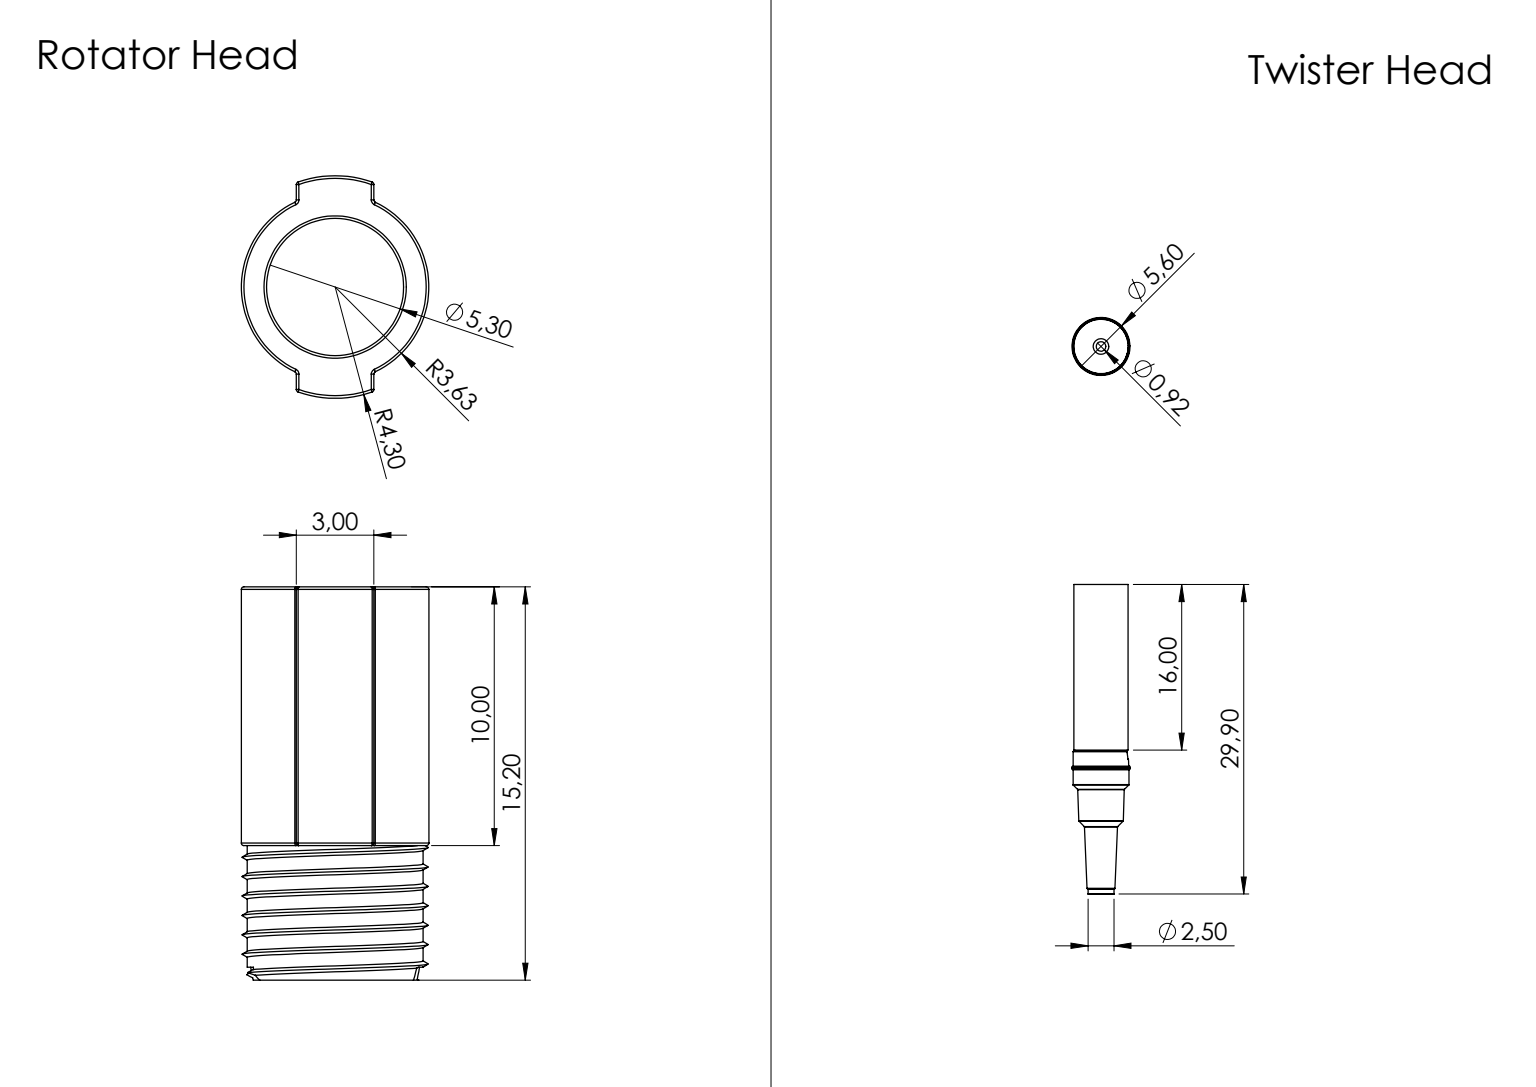
ISO-10303-21;
HEADER;
FILE_DESCRIPTION (('STEP AP214'),
    '1' );
FILE_NAME ('Rotator Head.step',
    '2026-10-06T14:00:01',
    ( '' ),
    ( '' ),
    'SwSTEP 2.0',
    'SolidWorks 2020',
    '' );
FILE_SCHEMA (( 'AUTOMOTIVE_DESIGN' ));
ENDSEC;

DATA;
#20=FACE_OUTER_BOUND ( 'NONE', #25184, .T. ) ;
#32=CARTESIAN_POINT ( 'NONE',  ( -59.59999999999998721, -2.157671697750204842, 1.538490443495526216 ) ) ;
#34=CARTESIAN_POINT ( 'NONE',  ( -60.95655989232410121, 1.962990915244748891, -3.400000000000207301 ) ) ;
#37=PRODUCT_DEFINITION_SHAPE ( 'NONE', 'NONE',  #1193 ) ;
#38=ORIENTED_EDGE ( 'NONE', *, *, #18350, .T. ) ;
#40=CARTESIAN_POINT ( 'NONE',  ( -59.74999999999995737, 2.023778652682510945E-14, -3.400000000000212186 ) ) ;
#45=EDGE_CURVE ( 'NONE', #27818, #13704, #24501, .T. ) ;
#46=CARTESIAN_POINT ( 'NONE',  ( -59.69999999999997442, -3.399999999999991473, -2.235080921937235780E-13 ) ) ;
#65=CARTESIAN_POINT ( 'NONE',  ( -57.19702994616204705, 4.156921938165313080, -1.880369327726949834E-13 ) ) ;
#71=CARTESIAN_POINT ( 'NONE',  ( -55.63452994616205416, 3.117691453623979481, 1.799999999999814415 ) ) ;
#72=EDGE_LOOP ( 'NONE', ( #23840, #15915, #20433, #20236, #22335, #16297, #17891, #10389 ) ) ;
#81=CARTESIAN_POINT ( 'NONE',  ( -59.60604010435355349, 3.187076279294280390, -1.184290838417780600 ) ) ;
#86=CARTESIAN_POINT ( 'NONE',  ( -59.59999999999997300, -2.337126060168364994, -1.249136413240117038 ) ) ;
#92=ORIENTED_EDGE ( 'NONE', *, *, #412, .F. ) ;
#106=( BOUNDED_CURVE ( )  B_SPLINE_CURVE ( 2, ( #27982, #6938, #12441, #31145, #14352, #9477, #26546, #29083, #5166 ),
 .UNSPECIFIED., .F., .T. ) 
 B_SPLINE_CURVE_WITH_KNOTS ( ( 3, 2, 2, 2, 3 ),
 ( 0.5833333333333333703, 0.5925925925925925597, 0.6111111111111111605, 0.6296296296296296502, 0.6388888888888889506 ),
 .UNSPECIFIED. ) 
 CURVE ( )  GEOMETRIC_REPRESENTATION_ITEM ( )  RATIONAL_B_SPLINE_CURVE ( ( 0.9330127018922194093, 0.9330127018922197424, 1.000000000000000000, 0.8660254037844387076, 1.000000000000000000, 0.8660254037844387076, 1.000000000000000000, 0.9330127018922189652, 0.9330127018922194093 ) ) 
 REPRESENTATION_ITEM ( '' )  );
#114=CARTESIAN_POINT ( 'NONE',  ( -56.89405989232413674, -3.920666489018330156E-15, 3.399999999999796962 ) ) ;
#151=DIRECTION ( 'NONE',  ( 1.000000000000000000, -1.219044193948983948E-29, 3.491481338843133355E-15 ) ) ;
#160=CARTESIAN_POINT ( 'NONE',  ( -54.49999999999996447, 1.400000000000023670, -3.959797974644871044 ) ) ;
#174=ORIENTED_EDGE ( 'NONE', *, *, #24601, .T. ) ;
#175=DIRECTION ( 'NONE',  ( -3.491481338843133355E-15, -3.491481338843133355E-15, 1.000000000000000000 ) ) ;
#185=CARTESIAN_POINT ( 'NONE',  ( -59.88452994616203995, -3.117691453623976816, 1.799999999999775335 ) ) ;
#197=CARTESIAN_POINT ( 'NONE',  ( -54.49999999999997868, 8.366749974758489177E-15, -2.216533082070116467E-13 ) ) ;
#202=DIRECTION ( 'NONE',  ( 0.000000000000000000, -1.000000000000000000, 0.000000000000000000 ) ) ;
#208=EDGE_CURVE ( 'NONE', #30643, #11413, #10315, .T. ) ;
#214=CARTESIAN_POINT ( 'NONE',  ( -55.32202994616205416, -4.156921938165296204, -2.115361882398036228E-13 ) ) ;
#222=CARTESIAN_POINT ( 'NONE',  ( -54.99999999999997868, 2.944486372867092250, 1.699999999999816103 ) ) ;
#231=CARTESIAN_POINT ( 'NONE',  ( -59.63746166535423043, 3.180335144039268869, -1.202432085119870431 ) ) ;
#259=CARTESIAN_POINT ( 'NONE',  ( -54.45655989232412963, -3.925981830489445379, -2.076939516179772989E-13 ) ) ;
#267=FACE_OUTER_BOUND ( 'NONE', #20625, .T. ) ;
#287=EDGE_LOOP ( 'NONE', ( #23710, #1168, #11704, #9445, #24779, #21712, #30444 ) ) ;
#294=FACE_OUTER_BOUND ( 'NONE', #8468, .T. ) ;
#298=AXIS2_PLACEMENT_3D ( 'NONE', #23512, #1809, #21167 ) ;
#303=CARTESIAN_POINT ( 'NONE',  ( -54.49999999999996447, -1.499999999999978684, -4.029888335922192866 ) ) ;
#309=ORIENTED_EDGE ( 'NONE', *, *, #15470, .F. ) ;
#331=EDGE_CURVE ( 'NONE', #21866, #1670, #17624, .T. ) ;
#334=DIRECTION ( 'NONE',  ( -3.208218335192195507E-15, 0.9428090415820656878, 0.3333333333333268200 ) ) ;
#336=AXIS2_PLACEMENT_3D ( 'NONE', #3654, #22838, #15841 ) ;
#339=CARTESIAN_POINT ( 'NONE',  ( -58.44702994616205416, -2.078460969082657872, 3.599999999999784261 ) ) ;
#375=CARTESIAN_POINT ( 'NONE',  ( -54.33155989232412253, -1.962990915244706924, -3.400000000000199751 ) ) ;
#387=CARTESIAN_POINT ( 'NONE',  ( -59.66183546925923764, -3.174920041538525251, -1.216504307364950854 ) ) ;
#396=DIRECTION ( 'NONE',  ( 0.000000000000000000, -1.000000000000000000, -3.491481338843133355E-15 ) ) ;
#397=CIRCLE ( 'NONE', #4439, 0.1000000000000000472 ) ;
#400=ORIENTED_EDGE ( 'NONE', *, *, #15115, .F. ) ;
#405=CARTESIAN_POINT ( 'NONE',  ( -54.56249999999997158, -1.962990915244707368, -3.400000000000200640 ) ) ;
#412=EDGE_CURVE ( 'NONE', #3421, #11190, #26852, .T. ) ;
#419=CARTESIAN_POINT ( 'NONE',  ( -44.59999999999998721, -1.557046979865776226, 3.273565289174722448 ) ) ;
#421=CARTESIAN_POINT ( 'NONE',  ( -60.13452994616204705, 3.117691453623979481, 1.799999999999798428 ) ) ;
#429=( BOUNDED_CURVE ( )  B_SPLINE_CURVE ( 2, ( #24054, #26755, #4426, #29116, #12032, #9964, #7268, #5054, #28814 ),
 .UNSPECIFIED., .F., .T. ) 
 B_SPLINE_CURVE_WITH_KNOTS ( ( 3, 2, 2, 2, 3 ),
 ( 0.4722222222222222654, 0.4814814814814814548, 0.5000000000000000000, 0.5185185185185184897, 0.5277777777777777901 ),
 .UNSPECIFIED. ) 
 CURVE ( )  GEOMETRIC_REPRESENTATION_ITEM ( )  RATIONAL_B_SPLINE_CURVE ( ( 0.9330127018922194093, 0.9330127018922197424, 1.000000000000000000, 0.8660254037844387076, 1.000000000000000000, 0.8660254037844387076, 1.000000000000000000, 0.9330127018922194093, 0.9330127018922194093 ) ) 
 REPRESENTATION_ITEM ( '' )  );
#435=CARTESIAN_POINT ( 'NONE',  ( -44.49999999999999289, 1.399999999999998135, 3.363870538531281262 ) ) ;
#437=( LENGTH_UNIT ( ) NAMED_UNIT ( * ) SI_UNIT ( .MILLI., .METRE. ) );
#453=DIRECTION ( 'NONE',  ( -2.095850865446309212E-30, -1.000000000000000000, -2.891205793294679411E-15 ) ) ;
#459=DIRECTION ( 'NONE',  ( 1.000000000000000000, -1.219044193948983948E-29, 3.491481338843133355E-15 ) ) ;
#461=B_SPLINE_CURVE_WITH_KNOTS ( 'NONE', 3,
 ( #4222, #6930, #25918, #30983 ),
 .UNSPECIFIED., .F., .F.,
 ( 4, 4 ),
 ( 0.0002256372043837409917, 0.0002420867138521805458 ),
 .UNSPECIFIED. ) ;
#462=CARTESIAN_POINT ( 'NONE',  ( -59.37009172985672478, 3.234433134214944161, -1.048065980887175952 ) ) ;
#470=CARTESIAN_POINT ( 'NONE',  ( -54.46975615167505680, -2.293836137973780165, -2.770930891520435146 ) ) ;
#488=B_SPLINE_CURVE_WITH_KNOTS ( 'NONE', 3,
 ( #12965, #29908, #15508, #8530, #3628, #17581, #20429, #20126, #6019, #10443, #30224, #18216, #25166, #5538, #13122, #20591 ),
 .UNSPECIFIED., .F., .F.,
 ( 4, 3, 3, 3, 3, 4 ),
 ( -2.161317903555403524E-06, 0.000000000000000000, 3.447636036923519868E-05, 7.048537632665564262E-05, 0.0001024680845135426304, 0.0001336460163216753082 ),
 .UNSPECIFIED. ) ;
#492=CARTESIAN_POINT ( 'NONE',  ( -58.50952994616205416, -4.643455692769885398E-15, 3.599999999999791367 ) ) ;
#495=CARTESIAN_POINT ( 'NONE',  ( -59.69999999999998153, -2.279157448682842091, 1.538811659727345349 ) ) ;
#525=CARTESIAN_POINT ( 'NONE',  ( -58.94702994616203284, -2.078460969082631227, -3.600000000000215472 ) ) ;
#527=CARTESIAN_POINT ( 'NONE',  ( -56.49999999999997868, 2.944486372867090029, 1.699999999999814548 ) ) ;
#532=CARTESIAN_POINT ( 'NONE',  ( -44.59999999999999432, -1.400000000000006795, 3.959797974644484242 ) ) ;
#544=FACE_BOUND ( 'NONE', #24096, .T. ) ;
#553=FACE_OUTER_BOUND ( 'NONE', #21182, .T. ) ;
#556=VERTEX_POINT ( 'NONE', #12979 ) ;
#559=DIRECTION ( 'NONE',  ( 1.000000000000000000, -1.219044193948983948E-29, 3.491481338843133355E-15 ) ) ;
#569=CARTESIAN_POINT ( 'NONE',  ( -59.94702994616205416, -2.078460969082657872, 3.599999999999778932 ) ) ;
#572=DIRECTION ( 'NONE',  ( 0.000000000000000000, -1.000000000000000000, -4.336808689942015369E-15 ) ) ;
#576=CARTESIAN_POINT ( 'NONE',  ( -59.67987798884427519, 2.349476376206463879, -1.226921160904890451 ) ) ;
#577=CIRCLE ( 'NONE', #19806, 3.624999999999996447 ) ;
#591=LINE ( 'NONE', #5506, #15902 ) ;
#625=ORIENTED_EDGE ( 'NONE', *, *, #7840, .T. ) ;
#629=CARTESIAN_POINT ( 'NONE',  ( -59.07202994616203995, -4.156921938165296204, -2.246292432604653256E-13 ) ) ;
#632=AXIS2_PLACEMENT_3D ( 'NONE', #9663, #16780, #24048 ) ;
#639=ORIENTED_EDGE ( 'NONE', *, *, #7228, .F. ) ;
#640=CARTESIAN_POINT ( 'NONE',  ( -59.07202994616203995, -4.156921938165296204, -2.246292432604653256E-13 ) ) ;
#642=CARTESIAN_POINT ( 'NONE',  ( -56.58155989232411542, -1.962990915244702483, -3.400000000000209077 ) ) ;
#645=CARTESIAN_POINT ( 'NONE',  ( -56.89405989232413674, -6.418945959278930492E-15, 3.399999999999796962 ) ) ;
#663=ORIENTED_EDGE ( 'NONE', *, *, #21235, .F. ) ;
#664=DIRECTION ( 'NONE',  ( 1.000000000000000000, -1.219044193948983948E-29, 3.491481338843133355E-15 ) ) ;
#671=CARTESIAN_POINT ( 'NONE',  ( -59.69702994616202574, -2.078460969082631227, -3.600000000000218137 ) ) ;
#676=DIRECTION ( 'NONE',  ( 3.491481338843133355E-15, 3.491481338843133355E-15, -1.000000000000000000 ) ) ;
#677=EDGE_CURVE ( 'NONE', #30092, #3236, #13549, .T. ) ;
#682=DIRECTION ( 'NONE',  ( 3.491481338843133355E-15, 3.491481338843133355E-15, -1.000000000000000000 ) ) ;
#683=CARTESIAN_POINT ( 'NONE',  ( -54.39999999999996305, 1.500000000000021538, -3.363870538531680054 ) ) ;
#713=EDGE_CURVE ( 'NONE', #19668, #15709, #16819, .T. ) ;
#717=CARTESIAN_POINT ( 'NONE',  ( -60.20655989232410832, 1.962990915244748891, -3.400000000000205969 ) ) ;
#721=DIRECTION ( 'NONE',  ( 0.000000000000000000, -1.000000000000000000, -3.491481338843137694E-15 ) ) ;
#725=CARTESIAN_POINT ( 'NONE',  ( -59.13207863537445519, -2.357771006092566513, 1.210922106982256663 ) ) ;
#752=ORIENTED_EDGE ( 'NONE', *, *, #11276, .F. ) ;
#758=CARTESIAN_POINT ( 'NONE',  ( -55.19702994616203284, -2.078460969082631227, -3.600000000000202593 ) ) ;
#780=CIRCLE ( 'NONE', #17971, 0.2000000000000000944 ) ;
#786=CARTESIAN_POINT ( 'NONE',  ( -59.63452994616203284, 2.093608279459373297E-14, -3.600000000000211475 ) ) ;
#789=CIRCLE ( 'NONE', #15973, 4.200000000000016165 ) ;
#794=EDGE_CURVE ( 'NONE', #2131, #1323, #2362, .T. ) ;
#796=AXIS2_PLACEMENT_3D ( 'NONE', #14846, #19782, #453 ) ;
#801=DIRECTION ( 'NONE',  ( 1.000000000000000000, -1.219044193948983948E-29, 3.491481338843133355E-15 ) ) ;
#807=AXIS2_PLACEMENT_3D ( 'NONE', #26000, #20498, #30125 ) ;
#817=EDGE_CURVE ( 'NONE', #4631, #20056, #25479, .T. ) ;
#826=VERTEX_POINT ( 'NONE', #15796 ) ;
#827=CYLINDRICAL_SURFACE ( 'NONE', #3289, 4.300000000000016698 ) ;
#828=ORIENTED_EDGE ( 'NONE', *, *, #31168, .F. ) ;
#836=CARTESIAN_POINT ( 'NONE',  ( -59.25952994616205416, -4.643455692769875931E-15, 3.599999999999788702 ) ) ;
#837=EDGE_LOOP ( 'NONE', ( #6700, #8690, #2350, #12267, #14721 ) ) ;
#840=ORIENTED_EDGE ( 'NONE', *, *, #14681, .F. ) ;
#841=CYLINDRICAL_SURFACE ( 'NONE', #1547, 0.1000000000000000472 ) ;
#842=AXIS2_PLACEMENT_3D ( 'NONE', #30434, #23332, #18747 ) ;
#846=CARTESIAN_POINT ( 'NONE',  ( -54.68749999999998579, -3.925981830489445379, -2.085002746943179415E-13 ) ) ;
#860=B_SPLINE_CURVE_WITH_KNOTS ( 'NONE', 3,
 ( #900, #8173, #17841, #27478, #25267, #5795, #1051, #10702, #11800, #2291 ),
 .UNSPECIFIED., .F., .F.,
 ( 4, 3, 3, 4 ),
 ( 1.063942921725272085E-15, 0.0001291030634103491155, 0.0002330573485935334081, 0.0003370282537953245587 ),
 .UNSPECIFIED. ) ;
#864=EDGE_CURVE ( 'NONE', #2131, #12851, #29047, .T. ) ;
#874=CARTESIAN_POINT ( 'NONE',  ( -59.10095151589816709, 2.309095926083573502, 1.300228524717358836 ) ) ;
#876=CARTESIAN_POINT ( 'NONE',  ( -58.81249999999996447, 3.925981830489463142, -1.945260624050196617E-13 ) ) ;
#887=CARTESIAN_POINT ( 'NONE',  ( -59.06249999999995737, -1.962990915244687828, -3.400000000000226841 ) ) ;
#888=ORIENTED_EDGE ( 'NONE', *, *, #6577, .T. ) ;
#891=CARTESIAN_POINT ( 'NONE',  ( -57.08155989232412963, 3.925981830489463142, -1.884825173204143128E-13 ) ) ;
#896=CARTESIAN_POINT ( 'NONE',  ( -59.19976204860608959, -2.440481952758566830, 1.249999143831215687 ) ) ;
#900=CARTESIAN_POINT ( 'NONE',  ( -59.41132486539680713, 3.361433066165957051, 1.250136525132557574 ) ) ;
#902=FACE_OUTER_BOUND ( 'NONE', #1457, .T. ) ;
#904=ADVANCED_FACE ( 'NONE', ( #16596 ), #23720, .F. ) ;
#908=AXIS2_PLACEMENT_3D ( 'NONE', #25148, #17875, #20268 ) ;
#915=ORIENTED_EDGE ( 'NONE', *, *, #13224, .F. ) ;
#916=CARTESIAN_POINT ( 'NONE',  ( -54.49999999999999289, 1.399999999999998135, 3.363870538531246179 ) ) ;
#920=ORIENTED_EDGE ( 'NONE', *, *, #8697, .T. ) ;
#921=CARTESIAN_POINT ( 'NONE',  ( -44.59999999999998721, 1.399999999999995914, 3.959797974644454488 ) ) ;
#922=LINE ( 'NONE', #27667, #8950 ) ;
#928=EDGE_LOOP ( 'NONE', ( #6714, #5334, #16373 ) ) ;
#931=DIRECTION ( 'NONE',  ( 0.000000000000000000, 1.000000000000000000, 4.336808689942015369E-15 ) ) ;
#945=CARTESIAN_POINT ( 'NONE',  ( -58.94702994616202574, -2.078460969082611243, -3.600000000000227018 ) ) ;
#950=VERTEX_POINT ( 'NONE', #419 ) ;
#952=CARTESIAN_POINT ( 'NONE',  ( -54.49305485193549003, -2.337873507123006345, -2.687031364304292680 ) ) ;
#955=ORIENTED_EDGE ( 'NONE', *, *, #22566, .T. ) ;
#961=CARTESIAN_POINT ( 'NONE',  ( -56.19702994616206837, -2.078460969082657872, 3.599999999999791811 ) ) ;
#968=ORIENTED_EDGE ( 'NONE', *, *, #28279, .T. ) ;
#971=ADVANCED_FACE ( 'NONE', ( #9768 ), #9919, .T. ) ;
#973=LINE ( 'NONE', #29606, #20741 ) ;
#977=CARTESIAN_POINT ( 'NONE',  ( -56.68749999999996447, 1.962990915244759771, -3.400000000000186873 ) ) ;
#981=CARTESIAN_POINT ( 'NONE',  ( -59.24236485150797904, -3.064388189877631063, 1.492323961017689493 ) ) ;
#985=FACE_OUTER_BOUND ( 'NONE', #19485, .T. ) ;
#988=CARTESIAN_POINT ( 'NONE',  ( -59.60127941732039147, -2.337454683938988698, -1.248534441610049450 ) ) ;
#995=CARTESIAN_POINT ( 'NONE',  ( -54.49999999999997868, 8.366749974758391359E-15, -1.938977325913827332E-13 ) ) ;
#1002=CARTESIAN_POINT ( 'NONE',  ( -58.63452994616204705, 3.117691453623979481, 1.799999999999803757 ) ) ;
#1004=ORIENTED_EDGE ( 'NONE', *, *, #24904, .T. ) ;
#1010=CARTESIAN_POINT ( 'NONE',  ( -58.87499999999996447, 2.944486372867106905, -1.700000000000196465 ) ) ;
#1032=CARTESIAN_POINT ( 'NONE',  ( -57.62499999999996447, -2.944486372867076707, -1.700000000000215117 ) ) ;
#1040=DIRECTION ( 'NONE',  ( -1.000000000000000000, 1.219044193948983948E-29, -3.491481338843133355E-15 ) ) ;
#1041=DIRECTION ( 'NONE',  ( 0.000000000000000000, -1.000000000000000000, -5.267838178243386187E-15 ) ) ;
#1043=EDGE_CURVE ( 'NONE', #13704, #26101, #4146, .T. ) ;
#1045=CARTESIAN_POINT ( 'NONE',  ( -57.95655989232411542, 1.962990915244748891, -3.400000000000197087 ) ) ;
#1051=CARTESIAN_POINT ( 'NONE',  ( -59.48031779539610397, 3.173620585043683384, 1.369635785239876169 ) ) ;
#1053=CARTESIAN_POINT ( 'NONE',  ( -54.39999999999996305, -1.599999999999981215, -3.363870538531692045 ) ) ;
#1057=ORIENTED_EDGE ( 'NONE', *, *, #12567, .T. ) ;
#1084=STYLED_ITEM ( 'NONE', ( #12456 ), #4756 ) ;
#1087=EDGE_CURVE ( 'NONE', #6214, #21890, #26505, .T. ) ;
#1090=CARTESIAN_POINT ( 'NONE',  ( -59.25952994616205416, -2.272369910876824241E-14, 3.599999999999788702 ) ) ;
#1095=CARTESIAN_POINT ( 'NONE',  ( -54.62499999999997158, -2.944486372867076707, -1.700000000000204903 ) ) ;
#1096=ORIENTED_EDGE ( 'NONE', *, *, #14201, .T. ) ;
#1106=CARTESIAN_POINT ( 'NONE',  ( -58.57202994616204705, 2.078460969082646770, 3.599999999999799805 ) ) ;
#1112=( BOUNDED_CURVE ( )  B_SPLINE_CURVE ( 2, ( #81, #29045, #4984, #14637, #24302 ),
 .UNSPECIFIED., .F., .T. ) 
 B_SPLINE_CURVE_WITH_KNOTS ( ( 3, 2, 3 ),
 ( 0.7562128299816163191, 0.7592592592592593004, 0.7702506610550023947 ),
 .UNSPECIFIED. ) 
 CURVE ( )  GEOMETRIC_REPRESENTATION_ITEM ( )  RATIONAL_B_SPLINE_CURVE ( ( 0.9631718388946364229, 0.9779602168519400118, 1.000000000000000000, 0.9204812946589053801, 0.9353569697113883752 ) ) 
 REPRESENTATION_ITEM ( '' )  );
#1116=CARTESIAN_POINT ( 'NONE',  ( -61.07202994616202574, 2.078460969082674747, -3.600000000000208367 ) ) ;
#1119=AXIS2_PLACEMENT_3D ( 'NONE', #13564, #20726, #23248 ) ;
#1132=CARTESIAN_POINT ( 'NONE',  ( -59.60063969940316042, -2.337287690019610231, -1.248834004845451373 ) ) ;
#1146=CARTESIAN_POINT ( 'NONE',  ( -56.20655989232413674, 1.962990915244722245, 3.399999999999807621 ) ) ;
#1151=CARTESIAN_POINT ( 'NONE',  ( -56.43749999999998579, 1.962990915244722689, 3.399999999999807621 ) ) ;
#1159=DIRECTION ( 'NONE',  ( 0.000000000000000000, 1.000000000000000000, 3.491481338843130594E-15 ) ) ;
#1161=CARTESIAN_POINT ( 'NONE',  ( -59.69999999999997442, 3.400000000000007905, -2.001823990013003858E-13 ) ) ;
#1168=ORIENTED_EDGE ( 'NONE', *, *, #3930, .F. ) ;
#1171=CARTESIAN_POINT ( 'NONE',  ( -59.09999999999998010, 2.308634493194285486, 1.301040651491358169 ) ) ;
#1174=CARTESIAN_POINT ( 'NONE',  ( -57.68749999999996447, -3.925981830489445379, -2.189747187108473037E-13 ) ) ;
#1178=CARTESIAN_POINT ( 'NONE',  ( -44.59999999999998010, 8.366749974758271452E-15, -1.593320673368357319E-13 ) ) ;
#1186=CARTESIAN_POINT ( 'NONE',  ( -59.26905989232412253, 2.944486372867092250, 1.699999999999800782 ) ) ;
#1187=DIRECTION ( 'NONE',  ( 0.000000000000000000, -1.000000000000000000, -4.336808689942015369E-15 ) ) ;
#1189=DIRECTION ( 'NONE',  ( -1.000000000000000000, 1.219044193948983948E-29, -3.491481338843133355E-15 ) ) ;
#1193=PRODUCT_DEFINITION ( 'UNKNOWN', '', #11600, #13260 ) ;
#1202=CARTESIAN_POINT ( 'NONE',  ( -59.58155989232410832, -1.962990915244687384, -3.400000000000229061 ) ) ;
#1233=ORIENTED_EDGE ( 'NONE', *, *, #11080, .T. ) ;
#1252=CARTESIAN_POINT ( 'NONE',  ( -54.39999999999999147, -1.600000000000004530, 3.363870538531237742 ) ) ;
#1264=DIRECTION ( 'NONE',  ( 1.000000000000000000, -1.219044193948983948E-29, 3.491481338843133355E-15 ) ) ;
#1272=EDGE_CURVE ( 'NONE', #16489, #14828, #18956, .T. ) ;
#1274=DIRECTION ( 'NONE',  ( -1.000000000000000000, 1.219044193948983948E-29, -3.491481338843133355E-15 ) ) ;
#1275=CARTESIAN_POINT ( 'NONE',  ( -59.64819772016205235, -2.360117159334204739, -1.232121303804351919 ) ) ;
#1278=EDGE_LOOP ( 'NONE', ( #7304, #6677, #15002, #25727 ) ) ;
#1281=AXIS2_PLACEMENT_3D ( 'NONE', #11954, #1983, #11794 ) ;
#1286=ORIENTED_EDGE ( 'NONE', *, *, #5679, .F. ) ;
#1292=CARTESIAN_POINT ( 'NONE',  ( -59.33155989232412253, 3.925981830489463142, -1.963383503328113345E-13 ) ) ;
#1295=ORIENTED_EDGE ( 'NONE', *, *, #23328, .F. ) ;
#1299=CARTESIAN_POINT ( 'NONE',  ( -55.49999999999997868, -2.944486372867089141, 1.699999999999791678 ) ) ;
#1306=EDGE_CURVE ( 'NONE', #30092, #16115, #28416, .T. ) ;
#1308=FACE_OUTER_BOUND ( 'NONE', #31128, .T. ) ;
#1311=CARTESIAN_POINT ( 'NONE',  ( -59.69464122902330416, 2.086944863889884871, 1.740854861534822273 ) ) ;
#1323=VERTEX_POINT ( 'NONE', #6412 ) ;
#1324=CARTESIAN_POINT ( 'NONE',  ( -59.19999999999997442, 4.156921938165309527, 1.250136525132554910 ) ) ;
#1326=CARTESIAN_POINT ( 'NONE',  ( -58.37499999999996447, -2.944486372867076707, -1.700000000000217781 ) ) ;
#1329=CIRCLE ( 'NONE', #6904, 3.399999999999999911 ) ;
#1342=CARTESIAN_POINT ( 'NONE',  ( -58.58155989232412253, 3.925981830489463142, -1.937197393286790192E-13 ) ) ;
#1344=ADVANCED_FACE ( 'NONE', ( #13352 ), #18735, .T. ) ;
#1376=DIRECTION ( 'NONE',  ( 1.000000000000000000, -1.219044193948983948E-29, 3.491481338843133355E-15 ) ) ;
#1390=CARTESIAN_POINT ( 'NONE',  ( -59.19999999999996732, -3.264622394567714192, -0.9498634748674711359 ) ) ;
#1409=ORIENTED_EDGE ( 'NONE', *, *, #26244, .T. ) ;
#1419=CARTESIAN_POINT ( 'NONE',  ( -59.35470925280786503, 2.309531243787677379, 1.299482330928217300 ) ) ;
#1425=DIRECTION ( 'NONE',  ( 1.216509871872722247E-14, 3.491481338843133355E-15, -1.000000000000000000 ) ) ;
#1430=CIRCLE ( 'NONE', #23702, 0.09999999999999992228 ) ;
#1439=CARTESIAN_POINT ( 'NONE',  ( -59.60191903105511813, -2.337626997591211619, -1.248237806062580058 ) ) ;
#1441=ORIENTED_EDGE ( 'NONE', *, *, #3910, .T. ) ;
#1451=VERTEX_POINT ( 'NONE', #23907 ) ;
#1452=SURFACE_STYLE_USAGE ( .BOTH. , #15858 ) ;
#1453=CARTESIAN_POINT ( 'NONE',  ( -55.19702994616203995, -2.078460969082628118, -3.600000000000204814 ) ) ;
#1454=CARTESIAN_POINT ( 'NONE',  ( -59.58155989232410832, -1.962990915244706924, -3.400000000000217515 ) ) ;
#1457=EDGE_LOOP ( 'NONE', ( #15335, #7101, #17819, #1921 ) ) ;
#1458=ORIENTED_EDGE ( 'NONE', *, *, #4399, .T. ) ;
#1461=CARTESIAN_POINT ( 'NONE',  ( -55.43749999999997158, -3.925981830489445379, -2.111188856984502568E-13 ) ) ;
#1465=CARTESIAN_POINT ( 'NONE',  ( -54.49999999999996447, -0.3490374893396158695, -3.419248390956425965 ) ) ;
#1470=CARTESIAN_POINT ( 'NONE',  ( -59.63821477905805324, 2.352792697908280495, -1.234285180173720020 ) ) ;
#1485=CARTESIAN_POINT ( 'NONE',  ( -44.59999999999995879, -1.433333333333312254, -4.054078878803053954 ) ) ;
#1486=CARTESIAN_POINT ( 'NONE',  ( -55.06249999999997158, 3.925981830489463142, -1.814330073843579337E-13 ) ) ;
#1488=ORIENTED_EDGE ( 'NONE', *, *, #4608, .T. ) ;
#1494=ORIENTED_EDGE ( 'NONE', *, *, #13570, .F. ) ;
#1507=CIRCLE ( 'NONE', #14142, 3.399999999999999911 ) ;
#1512=CARTESIAN_POINT ( 'NONE',  ( -59.51662234188409428, -2.295381144444371913, 1.432938519450777326 ) ) ;
#1530=ORIENTED_EDGE ( 'NONE', *, *, #16640, .F. ) ;
#1534=CARTESIAN_POINT ( 'NONE',  ( -56.29806624327023457, 3.400000000000004352, 0.9110272542656333572 ) ) ;
#1541=CARTESIAN_POINT ( 'NONE',  ( -57.82202994616206126, 2.078460969082646770, 3.599999999999802025 ) ) ;
#1546=DIRECTION ( 'NONE',  ( 1.000000000000000000, -1.219044193948983948E-29, 3.491481338843133355E-15 ) ) ;
#1547=AXIS2_PLACEMENT_3D ( 'NONE', #10510, #4108, #5912 ) ;
#1558=CARTESIAN_POINT ( 'NONE',  ( -59.50169947458152819, -2.403253767585091349, -1.124049747732174032 ) ) ;
#1560=DIRECTION ( 'NONE',  ( 0.000000000000000000, -1.000000000000000000, 0.000000000000000000 ) ) ;
#1562=CARTESIAN_POINT ( 'NONE',  ( -60.57202994616203995, -4.156921938165296204, -2.298664652687300067E-13 ) ) ;
#1577=DIRECTION ( 'NONE',  ( 0.000000000000000000, -1.000000000000000000, -4.379659758543263321E-15 ) ) ;
#1579=CARTESIAN_POINT ( 'NONE',  ( -54.39999999999996305, 1.400000000000023670, -3.959797974644871044 ) ) ;
#1587=DIRECTION ( 'NONE',  ( 0.000000000000000000, -1.000000000000000000, -3.491481338843133355E-15 ) ) ;
#1593=ORIENTED_EDGE ( 'NONE', *, *, #1272, .T. ) ;
#1597=CARTESIAN_POINT ( 'NONE',  ( -59.69999999999996732, -2.937205337104083380, -1.958225367202403921 ) ) ;
#1600=CARTESIAN_POINT ( 'NONE',  ( -56.45655989232411542, 1.962990915244748891, -3.400000000000191314 ) ) ;
#1602=ORIENTED_EDGE ( 'NONE', *, *, #208, .T. ) ;
#1607=CARTESIAN_POINT ( 'NONE',  ( -57.12499999999997868, -3.920666489018328579E-15, 3.399999999999796518 ) ) ;
#1608=DIRECTION ( 'NONE',  ( 0.000000000000000000, 1.000000000000000000, 3.491481338843130594E-15 ) ) ;
#1611=CARTESIAN_POINT ( 'NONE',  ( -44.49999999999997868, -2.749999999999991562, -1.685844928847700069E-13 ) ) ;
#1615=CARTESIAN_POINT ( 'NONE',  ( -59.65728261716281366, 2.366782727822268839, -1.230152085140874263 ) ) ;
#1622=CARTESIAN_POINT ( 'NONE',  ( -54.49999999999995737, -3.485114741320604281, -0.1344221940317323061 ) ) ;
#1627=CARTESIAN_POINT ( 'NONE',  ( -59.62499999999996447, 2.944486372867106905, -1.700000000000199130 ) ) ;
#1639=CARTESIAN_POINT ( 'NONE',  ( -54.47481206296395584, -2.548105035733319035, -2.538836448934781664 ) ) ;
#1644=DIRECTION ( 'NONE',  ( 7.637891338979824674E-45, -1.000000000000000000, -3.491481338843135327E-15 ) ) ;
#1646=CARTESIAN_POINT ( 'NONE',  ( -59.41132486540516311, 2.423250918913632201, 1.250136525132548027 ) ) ;
#1670=VERTEX_POINT ( 'NONE', #21711 ) ;
#1684=CARTESIAN_POINT ( 'NONE',  ( -58.88452994616202574, 2.093608279459372350E-14, -3.600000000000208811 ) ) ;
#1690=CARTESIAN_POINT ( 'NONE',  ( -54.39999999999997016, 1.514093959731561467, -3.183260039818582854 ) ) ;
#1697=CARTESIAN_POINT ( 'NONE',  ( -57.24999999999997158, 2.944486372867089585, 1.699999999999812772 ) ) ;
#1705=CARTESIAN_POINT ( 'NONE',  ( -59.14665968485343228, -2.559517124687094913, -0.9190674295589560394 ) ) ;
#1707=CARTESIAN_POINT ( 'NONE',  ( -60.00952994616204705, -4.643455692769866465E-15, 3.599999999999786038 ) ) ;
#1711=VECTOR ( 'NONE', #4485, 1000.000000000000000 ) ;
#1724=DIRECTION ( 'NONE',  ( 1.000000000000000000, -1.219044193948983948E-29, 3.491481338843133355E-15 ) ) ;
#1745=DIRECTION ( 'NONE',  ( 0.000000000000000000, -1.000000000000000000, 0.000000000000000000 ) ) ;
#1750=VERTEX_POINT ( 'NONE', #1390 ) ;
#1753=( NAMED_UNIT ( * ) PLANE_ANGLE_UNIT ( ) SI_UNIT ( $, .RADIAN. ) );
#1755=CARTESIAN_POINT ( 'NONE',  ( -57.08155989232412963, 3.925981830489463142, -1.884825173204143128E-13 ) ) ;
#1761=CARTESIAN_POINT ( 'NONE',  ( -59.24999999999997158, -2.944486372867089141, 1.699999999999778799 ) ) ;
#1762=CARTESIAN_POINT ( 'NONE',  ( -54.95655989232412963, 1.962990915244748891, -3.400000000000186873 ) ) ;
#1764=CIRCLE ( 'NONE', #11908, 0.1000000000000000472 ) ;
#1769=FACE_OUTER_BOUND ( 'NONE', #8576, .T. ) ;
#1780=ADVANCED_FACE ( 'NONE', ( #27682 ), #17831, .T. ) ;
#1783=CARTESIAN_POINT ( 'NONE',  ( -59.69142724121850563, 2.412383461849218591, -1.233589124872089826 ) ) ;
#1784=CARTESIAN_POINT ( 'NONE',  ( -55.82202994616203995, 2.078460969082674747, -3.600000000000189715 ) ) ;
#1788=CIRCLE ( 'NONE', #16470, 0.1000000000000000749 ) ;
#1797=AXIS2_PLACEMENT_3D ( 'NONE', #7442, #459, #10123 ) ;
#1798=EDGE_CURVE ( 'NONE', #21024, #15281, #30548, .T. ) ;
#1804=CIRCLE ( 'NONE', #13399, 0.1000000000000000472 ) ;
#1809=DIRECTION ( 'NONE',  ( 1.000000000000000000, -1.219044193948983948E-29, 3.491481338843133355E-15 ) ) ;
#1817=B_SPLINE_CURVE_WITH_KNOTS ( 'NONE', 3,
 ( #2704, #19960, #3016, #15045, #17748, #10143, #7918 ),
 .UNSPECIFIED., .F., .F.,
 ( 4, 3, 4 ),
 ( 0.000000000000000000, 4.155177920956839920E-05, 5.510430741949099299E-05 ),
 .UNSPECIFIED. ) ;
#1820=CIRCLE ( 'NONE', #4856, 0.1000000000000000472 ) ;
#1821=LINE ( 'NONE', #11495, #16058 ) ;
#1825=VERTEX_POINT ( 'NONE', #11482 ) ;
#1840=CARTESIAN_POINT ( 'NONE',  ( -59.69999999999997442, 8.366749974758454467E-15, -2.120534355533670266E-13 ) ) ;
#1848=VECTOR ( 'NONE', #24236, 1000.000000000000000 ) ;
#1854=CARTESIAN_POINT ( 'NONE',  ( -59.57202994616203995, 2.078460969082674747, -3.600000000000202593 ) ) ;
#1855=VECTOR ( 'NONE', #18825, 1000.000000000000000 ) ;
#1857=AXIS2_PLACEMENT_3D ( 'NONE', #23515, #15768, #11021 ) ;
#1873=SPHERICAL_SURFACE ( 'NONE', #24635, 0.1000000000000000056 ) ;
#1874=ORIENTED_EDGE ( 'NONE', *, *, #12571, .T. ) ;
#1879=DIRECTION ( 'NONE',  ( 0.000000000000000000, -1.000000000000000000, -3.491481338843129017E-15 ) ) ;
#1893=CARTESIAN_POINT ( 'NONE',  ( -55.24005354137803181, -3.399999999999995026, 0.9110272542656064898 ) ) ;
#1909=VECTOR ( 'NONE', #16588, 1000.000000000000000 ) ;
#1921=ORIENTED_EDGE ( 'NONE', *, *, #16414, .T. ) ;
#1934=CARTESIAN_POINT ( 'NONE',  ( -60.14405989232410832, 2.944486372867106461, -1.700000000000200684 ) ) ;
#1938=EDGE_LOOP ( 'NONE', ( #12459, #23077, #1593, #2183, #2772, #8705, #7012, #6440, #1602, #10918, #15569, #29963, #25365, #13655, #18880, #9456, #23543 ) ) ;
#1940=CARTESIAN_POINT ( 'NONE',  ( -56.13452994616205416, -3.117691453623976816, 1.799999999999788436 ) ) ;
#1953=CARTESIAN_POINT ( 'NONE',  ( -59.44102194137920492, 2.226395001412990737, 1.446970701571959728 ) ) ;
#1956=LINE ( 'NONE', #28548, #26629 ) ;
#1957=CARTESIAN_POINT ( 'NONE',  ( -54.39999999999999147, -1.433333333333339343, 4.054078878802656938 ) ) ;
#1962=CARTESIAN_POINT ( 'NONE',  ( -59.74999999999995737, 2.023778652682510945E-14, -3.400000000000212186 ) ) ;
#1964=ORIENTED_EDGE ( 'NONE', *, *, #8148, .T. ) ;
#1970=CARTESIAN_POINT ( 'NONE',  ( -54.38452994616203995, 2.093608279459366986E-14, -3.600000000000193268 ) ) ;
#1975=CARTESIAN_POINT ( 'NONE',  ( -54.49400863111429061, -3.204489435302700695, -1.562885166739987008 ) ) ;
#1983=DIRECTION ( 'NONE',  ( -1.000000000000000000, 1.219044193948983948E-29, -3.491481338843133355E-15 ) ) ;
#2008=CARTESIAN_POINT ( 'NONE',  ( -59.19999999999996732, 3.264622394567737729, -0.9498634748674483763 ) ) ;
#2015=CARTESIAN_POINT ( 'NONE',  ( -54.39999999999996305, -1.399999999999979039, -3.959797974644881258 ) ) ;
#2016=CARTESIAN_POINT ( 'NONE',  ( -58.38452994616204705, -3.117691453623976816, 1.799999999999780442 ) ) ;
#2017=CARTESIAN_POINT ( 'NONE',  ( -59.37009172985672478, 3.234433134214944161, -1.048065980887175952 ) ) ;
#2020=CARTESIAN_POINT ( 'NONE',  ( -59.19999999999997442, -3.371540527096009932, 0.6493167879416990029 ) ) ;
#2032=CARTESIAN_POINT ( 'NONE',  ( -57.37499999999996447, 2.944486372867110902, -1.700000000000183809 ) ) ;
#2041=CARTESIAN_POINT ( 'NONE',  ( -54.49999999999996447, 1.400000000000021450, -3.363870538531680943 ) ) ;
#2048=CARTESIAN_POINT ( 'NONE',  ( -59.69464122902330416, 2.086944863889884871, 1.740854861534822273 ) ) ;
#2057=DIRECTION ( 'NONE',  ( 0.000000000000000000, 1.000000000000000000, 3.491481338843132961E-15 ) ) ;
#2065=CARTESIAN_POINT ( 'NONE',  ( -59.69999999999996732, -1.873569517744609447, -3.074042495181142698 ) ) ;
#2072=ORIENTED_EDGE ( 'NONE', *, *, #4979, .F. ) ;
#2083=CARTESIAN_POINT ( 'NONE',  ( -60.33155989232410121, -1.962990915244706924, -3.400000000000220179 ) ) ;
#2087=CARTESIAN_POINT ( 'NONE',  ( -59.56249999999996447, 3.925981830489463142, -1.971446734091520023E-13 ) ) ;
#2088=PLANE ( 'NONE',  #22096 ) ;
#2095=EDGE_CURVE ( 'NONE', #20905, #12969, #10805, .T. ) ;
#2103=EDGE_LOOP ( 'NONE', ( #1874, #13106, #955, #8764, #22442, #24197 ) ) ;
#2109=ORIENTED_EDGE ( 'NONE', *, *, #20115, .T. ) ;
#2111=DIRECTION ( 'NONE',  ( 1.000000000000000000, -1.219044193948983948E-29, 3.491481338843133355E-15 ) ) ;
#2112=CARTESIAN_POINT ( 'NONE',  ( -60.24999999999997158, 2.944486372867092250, 1.699999999999797673 ) ) ;
#2116=CARTESIAN_POINT ( 'NONE',  ( -59.53611077946203523, 3.324882312671999518, -1.143917123867393304 ) ) ;
#2119=AXIS2_PLACEMENT_3D ( 'NONE', #12111, #21793, #7351 ) ;
#2120=CARTESIAN_POINT ( 'NONE',  ( -54.69702994616206837, -2.078460969082657872, 3.599999999999797584 ) ) ;
#2123=CARTESIAN_POINT ( 'NONE',  ( -59.53056271719990633, -2.463209972446139595, -1.140713948626901120 ) ) ;
#2131=VERTEX_POINT ( 'NONE', #683 ) ;
#2135=CARTESIAN_POINT ( 'NONE',  ( -54.39999999999996305, -1.499999999999981126, -3.363870538531691601 ) ) ;
#2157=VERTEX_POINT ( 'NONE', #4300 ) ;
#2165=CARTESIAN_POINT ( 'NONE',  ( -56.50952994616203995, 3.117691453623994580, -1.800000000000187006 ) ) ;
#2172=CARTESIAN_POINT ( 'NONE',  ( -59.19999999999997442, 4.156921938165317520, -0.9498634748674451567 ) ) ;
#2183=ORIENTED_EDGE ( 'NONE', *, *, #11013, .T. ) ;
#2195=CARTESIAN_POINT ( 'NONE',  ( -55.51905989232413674, 2.944486372867090029, 1.699999999999817213 ) ) ;
#2203=CARTESIAN_POINT ( 'NONE',  ( -57.31249999999996447, 3.400000000000008349, -1.881930883448047941E-13 ) ) ;
#2215=CARTESIAN_POINT ( 'NONE',  ( -55.06249999999997158, 3.400000000000007905, -1.826733775103631524E-13 ) ) ;
#2219=CARTESIAN_POINT ( 'NONE',  ( -59.69999999999997442, 3.400000000000007905, -2.001823990013003858E-13 ) ) ;
#2222=VERTEX_POINT ( 'NONE', #11267 ) ;
#2233=CARTESIAN_POINT ( 'NONE',  ( -59.89405989232412963, -3.920666489018293080E-15, 3.399999999999786304 ) ) ;
#2237=B_SPLINE_CURVE_WITH_KNOTS ( 'NONE', 3,
 ( #11135, #20811, #30132, #1622, #10989, #18434, #20669, #18135 ),
 .UNSPECIFIED., .F., .F.,
 ( 4, 2, 2, 4 ),
 ( 0.001352388525252836175, 0.001863402819022369787, 0.002374417112791903615, 0.003396445700330970839 ),
 .UNSPECIFIED. ) ;
#2238=CARTESIAN_POINT ( 'NONE',  ( -54.44702994616203995, -2.078460969082631227, -3.600000000000199485 ) ) ;
#2260=LINE ( 'NONE', #26488, #13429 ) ;
#2263=CIRCLE ( 'NONE', #18464, 0.1000000000000000472 ) ;
#2266=CARTESIAN_POINT ( 'NONE',  ( -54.75952994616206837, -4.643455692769931152E-15, 3.599999999999804245 ) ) ;
#2270=CARTESIAN_POINT ( 'NONE',  ( -59.56618930482535745, 3.265896025948629600, -1.161282968582738162 ) ) ;
#2273=CARTESIAN_POINT ( 'NONE',  ( -54.75952994616206837, -4.643455692769931152E-15, 3.599999999999804245 ) ) ;
#2288=CARTESIAN_POINT ( 'NONE',  ( -59.40743313238012036, 2.395752775956333291, 1.250136525132548027 ) ) ;
#2290=AXIS2_PLACEMENT_3D ( 'NONE', #12031, #18847, #14381 ) ;
#2291=CARTESIAN_POINT ( 'NONE',  ( -59.51024032614731851, 3.088598804228899652, 1.421463128792039843 ) ) ;
#2302=CARTESIAN_POINT ( 'NONE',  ( -59.11588618124505246, -2.336267030162283653, 1.253430707195199334 ) ) ;
#2317=AXIS2_PLACEMENT_3D ( 'NONE', #23251, #22931, #30357 ) ;
#2318=ORIENTED_EDGE ( 'NONE', *, *, #23511, .F. ) ;
#2325=EDGE_CURVE ( 'NONE', #9593, #10413, #9631, .T. ) ;
#2326=CARTESIAN_POINT ( 'NONE',  ( -56.39405989232412253, 2.944486372867106461, -1.700000000000187583 ) ) ;
#2335=CARTESIAN_POINT ( 'NONE',  ( -59.68658240507107138, -2.223882124562203799, 1.531065007683262591 ) ) ;
#2350=ORIENTED_EDGE ( 'NONE', *, *, #13832, .F. ) ;
#2353=FACE_OUTER_BOUND ( 'NONE', #837, .T. ) ;
#2357=EDGE_LOOP ( 'NONE', ( #7788, #752, #639, #20784 ) ) ;
#2362=LINE ( 'NONE', #12030, #8793 ) ;
#2388=CYLINDRICAL_SURFACE ( 'NONE', #28487, 0.09999999999999982514 ) ;
#2406=DIRECTION ( 'NONE',  ( -2.095850865446309212E-30, -1.000000000000000000, -2.891205793294679411E-15 ) ) ;
#2411=CARTESIAN_POINT ( 'NONE',  ( -60.93749999999997868, 1.962990915244722689, 3.399999999999791633 ) ) ;
#2425=DIRECTION ( 'NONE',  ( 0.000000000000000000, 1.000000000000000000, 3.491481338843130594E-15 ) ) ;
#2439=CARTESIAN_POINT ( 'NONE',  ( -57.13452994616205416, 3.117691453623979481, 1.799999999999809086 ) ) ;
#2442=CARTESIAN_POINT ( 'NONE',  ( -59.48573950359912743, 3.423031164920794289, -1.114835254188495162 ) ) ;
#2446=CARTESIAN_POINT ( 'NONE',  ( -56.07202994616204705, -4.156921938165296204, -2.141547992439359634E-13 ) ) ;
#2449=EDGE_CURVE ( 'NONE', #950, #3421, #973, .T. ) ;
#2463=B_SPLINE_CURVE_WITH_KNOTS ( 'NONE', 3,
 ( #10047, #7803, #29654, #14781 ),
 .UNSPECIFIED., .F., .F.,
 ( 4, 4 ),
 ( 0.000000000000000000, 7.924777108412403711E-05 ),
 .UNSPECIFIED. ) ;
#2468=EDGE_CURVE ( 'NONE', #11413, #17625, #14760, .T. ) ;
#2470=CIRCLE ( 'NONE', #20185, 0.1000000000000001721 ) ;
#2480=EDGE_LOOP ( 'NONE', ( #29463, #7474, #4333, #26667, #1530 ) ) ;
#2493=CARTESIAN_POINT ( 'NONE',  ( -56.14405989232413674, -3.920666489018339623E-15, 3.399999999999799627 ) ) ;
#2504=CARTESIAN_POINT ( 'NONE',  ( -44.59999999999997300, -3.624999999999988010, -1.997442628057709707E-13 ) ) ;
#2511=( BOUNDED_CURVE ( )  B_SPLINE_CURVE ( 3, ( #2017, #28308, #24021, #8986 ),
 .UNSPECIFIED., .F., .T. ) 
 B_SPLINE_CURVE_WITH_KNOTS ( ( 4, 4 ),
 ( 4.399031134232678220, 4.429249381401446861 ),
 .UNSPECIFIED. ) 
 CURVE ( )  GEOMETRIC_REPRESENTATION_ITEM ( )  RATIONAL_B_SPLINE_CURVE ( ( 1.000000000000000000, 0.9999239062424463143, 0.9999239062424463143, 1.000000000000000000 ) ) 
 REPRESENTATION_ITEM ( '' )  );
#2512=AXIS2_PLACEMENT_3D ( 'NONE', #8226, #3489, #30379 ) ;
#2530=CARTESIAN_POINT ( 'NONE',  ( -55.18749999999996447, 1.962990915244749557, -3.400000000000187761 ) ) ;
#2542=CARTESIAN_POINT ( 'NONE',  ( -59.51761855918065436, 2.467398989037824286, -1.133240635510041727 ) ) ;
#2549=EDGE_CURVE ( 'NONE', #28731, #28363, #7089, .T. ) ;
#2573=CARTESIAN_POINT ( 'NONE',  ( -57.50952994616203995, -3.117691453623963938, -1.800000000000215206 ) ) ;
#2575=DIRECTION ( 'NONE',  ( 0.000000000000000000, -1.000000000000000000, -3.491481338843139666E-15 ) ) ;
#2592=VERTEX_POINT ( 'NONE', #6332 ) ;
#2601=EDGE_CURVE ( 'NONE', #10532, #10212, #24224, .T. ) ;
#2602=CARTESIAN_POINT ( 'NONE',  ( -57.13452994616205416, 3.117691453623979481, 1.799999999999809086 ) ) ;
#2609=CARTESIAN_POINT ( 'NONE',  ( -54.81249999999998579, -1.962990915244731793, 3.399999999999796962 ) ) ;
#2640=SPHERICAL_SURFACE ( 'NONE', #24366, 0.1000000000000000056 ) ;
#2641=CARTESIAN_POINT ( 'NONE',  ( -55.45655989232413674, 1.962990915244722245, 3.399999999999810285 ) ) ;
#2642=AXIS2_PLACEMENT_3D ( 'NONE', #10077, #5160, #14512 ) ;
#2648=CARTESIAN_POINT ( 'NONE',  ( -59.09999999999997300, -2.465712773623968790, -0.9709585562669303949 ) ) ;
#2652=( BOUNDED_SURFACE ( )  B_SPLINE_SURFACE ( 3, 2, ( 
 ( #8152, #20210, #20514 ),
 ( #17823, #8465, #27782 ),
 ( #29840, #3566, #20039 ),
 ( #13341, #6097, #15119 ) ),
 .UNSPECIFIED., .F., .F., .F. ) 
 B_SPLINE_SURFACE_WITH_KNOTS ( ( 4, 4 ),
 ( 3, 3 ),
 ( 0.8603049414497402347, 1.079657356097645904 ),
 ( 0.000000000000000000, 1.000000000000000000 ),
 .UNSPECIFIED. ) 
 GEOMETRIC_REPRESENTATION_ITEM ( )  RATIONAL_B_SPLINE_SURFACE ( (
 ( 1.000000000000000000, 0.8142797953134848221, 1.000000000000000000),
 ( 1.000000000000000000, 0.8057719789464390381, 1.000000000000000000),
 ( 1.000000000000000000, 0.7963243424565560336, 1.000000000000000000),
 ( 1.000000000000000000, 0.7860710104634932582, 1.000000000000000000) ) ) 
 REPRESENTATION_ITEM ( '' )  SURFACE ( )  );
#2675=CARTESIAN_POINT ( 'NONE',  ( -44.49999999999999289, -1.514093959731547701, 3.183260039818174292 ) ) ;
#2676=CARTESIAN_POINT ( 'NONE',  ( -55.12499999999997158, 2.944486372867106905, -1.700000000000183364 ) ) ;
#2695=DIRECTION ( 'NONE',  ( 0.000000000000000000, 1.000000000000000000, 3.491481338843133355E-15 ) ) ;
#2703=EDGE_LOOP ( 'NONE', ( #25204, #3417, #7605 ) ) ;
#2704=CARTESIAN_POINT ( 'NONE',  ( -59.19999999999997442, 2.449420067797480893, 1.250136525132548693 ) ) ;
#2712=CARTESIAN_POINT ( 'NONE',  ( -60.13452994616204705, 3.117691453623979481, 1.799999999999798428 ) ) ;
#2713=EDGE_CURVE ( 'NONE', #12851, #3601, #26251, .T. ) ;
#2744=CARTESIAN_POINT ( 'NONE',  ( -55.00952994616204705, 3.117691453623994580, -1.800000000000181899 ) ) ;
#2746=CARTESIAN_POINT ( 'NONE',  ( -56.22099364905387375, -3.399999999999995026, 0.9110272542656009387 ) ) ;
#2764=EDGE_LOOP ( 'NONE', ( #7716, #25036, #18191, #9218, #27487 ) ) ;
#2772=ORIENTED_EDGE ( 'NONE', *, *, #817, .T. ) ;
#2785=CARTESIAN_POINT ( 'NONE',  ( -54.76905989232412963, 2.944486372867092250, 1.699999999999816769 ) ) ;
#2802=SURFACE_STYLE_FILL_AREA ( #7571 ) ;
#2808=CARTESIAN_POINT ( 'NONE',  ( -57.45655989232412253, -3.399999999999991029, -2.148039047887444390E-13 ) ) ;
#2865=EDGE_CURVE ( 'NONE', #6165, #5500, #8545, .T. ) ;
#2868=CARTESIAN_POINT ( 'NONE',  ( -59.69702994616202574, -2.078460969082631227, -3.600000000000218137 ) ) ;
#2885=AXIS2_PLACEMENT_3D ( 'NONE', #24703, #175, #26916 ) ;
#2903=VECTOR ( 'NONE', #1376, 1000.000000000000000 ) ;
#2904=CARTESIAN_POINT ( 'NONE',  ( -61.07202994616202574, 2.078460969082674747, -3.600000000000208367 ) ) ;
#2914=B_SPLINE_CURVE_WITH_KNOTS ( 'NONE', 3,
 ( #22658, #17582, #24989, #27524, #29909, #952, #9988, #27055, #19655, #27226, #10604, #3007, #10444, #22333, #470, #12497 ),
 .UNSPECIFIED., .F., .F.,
 ( 4, 2, 2, 2, 2, 2, 2, 4 ),
 ( 4.367276169273258306E-17, 0.0003166453355160177481, 0.0003958066693950119258, 0.0004353873363345080118, 0.0004452825030693815318, 0.0004551776698042549977, 0.0004749680032740019836, 0.0006332906710319628546 ),
 .UNSPECIFIED. ) ;
#2917=AXIS2_PLACEMENT_3D ( 'NONE', #6284, #15934, #25594 ) ;
#2929=EDGE_LOOP ( 'NONE', ( #4413, #1004, #26925, #14132, #17816, #15391 ) ) ;
#2930=EDGE_CURVE ( 'NONE', #27818, #20905, #21739, .T. ) ;
#2937=DIRECTION ( 'NONE',  ( 0.000000000000000000, -1.000000000000000000, -3.491481338843252079E-15 ) ) ;
#2949=EDGE_CURVE ( 'NONE', #30858, #5493, #3451, .T. ) ;
#2951=CARTESIAN_POINT ( 'NONE',  ( -56.01905989232412963, -2.944486372867088697, 1.699999999999789679 ) ) ;
#2960=( BOUNDED_CURVE ( )  B_SPLINE_CURVE ( 2, ( #17855, #15155, #22614 ),
 .UNSPECIFIED., .F., .T. ) 
 B_SPLINE_CURVE_WITH_KNOTS ( ( 3, 3 ),
 ( 0.6944444444444445308, 0.6961765869809276586 ),
 .UNSPECIFIED. ) 
 CURVE ( )  GEOMETRIC_REPRESENTATION_ITEM ( )  RATIONAL_B_SPLINE_CURVE ( ( 0.9330127018922194093, 0.9330127018922194093, 0.9353569697113865988 ) ) 
 REPRESENTATION_ITEM ( '' )  );
#2967=EDGE_CURVE ( 'NONE', #15088, #12969, #19693, .T. ) ;
#2970=ADVANCED_FACE ( 'NONE', ( #20839 ), #16151, .T. ) ;
#2987=CIRCLE ( 'NONE', #21207, 4.299999999999954525 ) ;
#2995=AXIS2_PLACEMENT_3D ( 'NONE', #6423, #20993, #16391 ) ;
#3007=CARTESIAN_POINT ( 'NONE',  ( -54.48229591105965142, -2.371389875144092496, -2.684526205802663767 ) ) ;
#3015=CARTESIAN_POINT ( 'NONE',  ( -59.00952994616203284, -3.117691453623963938, -1.800000000000220757 ) ) ;
#3016=CARTESIAN_POINT ( 'NONE',  ( -59.19766939034450104, 2.421524988789188093, 1.250136525132548693 ) ) ;
#3024=CARTESIAN_POINT ( 'NONE',  ( -57.88452994616205416, 3.117691453623979481, 1.799999999999806422 ) ) ;
#3031=CARTESIAN_POINT ( 'NONE',  ( -59.69999999999997442, 8.366749974758454467E-15, -2.120534355533670266E-13 ) ) ;
#3038=ORIENTED_EDGE ( 'NONE', *, *, #18261, .F. ) ;
#3046=CARTESIAN_POINT ( 'NONE',  ( -58.12499999999996447, 2.944486372867111346, -1.700000000000185585 ) ) ;
#3051=ORIENTED_EDGE ( 'NONE', *, *, #29412, .F. ) ;
#3059=CARTESIAN_POINT ( 'NONE',  ( -60.57202994616203995, -4.156921938165296204, -2.298664652687300067E-13 ) ) ;
#3098=CARTESIAN_POINT ( 'NONE',  ( -59.58155989232410832, -1.962990915244706924, -3.400000000000217515 ) ) ;
#3104=ADVANCED_FACE ( 'NONE', ( #4517 ), #13166, .T. ) ;
#3119=EDGE_LOOP ( 'NONE', ( #8561, #10506, #21653, #15777 ) ) ;
#3128=CARTESIAN_POINT ( 'NONE',  ( -57.58155989232413674, -1.962990915244744006, 3.399999999999780087 ) ) ;
#3135=EDGE_LOOP ( 'NONE', ( #3562, #28766, #24879, #14573 ) ) ;
#3145=EDGE_CURVE ( 'NONE', #23000, #3568, #6893, .T. ) ;
#3150=CARTESIAN_POINT ( 'NONE',  ( -59.40362242792826919, 3.375967812128700452, 1.250136525132546916 ) ) ;
#3165=CARTESIAN_POINT ( 'NONE',  ( -56.63452994616203284, 2.093608279459369510E-14, -3.600000000000201261 ) ) ;
#3175=CARTESIAN_POINT ( 'NONE',  ( -57.32202994616202574, 2.078460969082674747, -3.600000000000194600 ) ) ;
#3177=CARTESIAN_POINT ( 'NONE',  ( -56.45655989232411542, 1.962990915244759771, -3.400000000000185540 ) ) ;
#3178=CARTESIAN_POINT ( 'NONE',  ( -54.49999999999999289, -1.400000000000006795, 3.959797974644449603 ) ) ;
#3190=CARTESIAN_POINT ( 'NONE',  ( -59.09999999999998010, 2.308634493194285486, 1.301040651491358169 ) ) ;
#3207=CARTESIAN_POINT ( 'NONE',  ( -60.50952994616203284, -3.117691453623963938, -1.800000000000225864 ) ) ;
#3211=AXIS2_PLACEMENT_3D ( 'NONE', #5499, #20080, #29257 ) ;
#3213=AXIS2_PLACEMENT_3D ( 'NONE', #19230, #16692, #27261 ) ;
#3218=CARTESIAN_POINT ( 'NONE',  ( -54.49999999999996447, 2.023778652682504319E-14, -3.400000000000193978 ) ) ;
#3228=CARTESIAN_POINT ( 'NONE',  ( -59.69999155897362186, 2.119262223567999648, 1.750121904846017262 ) ) ;
#3234=CARTESIAN_POINT ( 'NONE',  ( -59.69931151237160805, -2.442379059721019541, -1.238141110944712242 ) ) ;
#3236=VERTEX_POINT ( 'NONE', #27428 ) ;
#3248=ORIENTED_EDGE ( 'NONE', *, *, #7501, .F. ) ;
#3257=CARTESIAN_POINT ( 'NONE',  ( -60.89405989232410121, 2.944486372867106461, -1.700000000000203348 ) ) ;
#3281=ORIENTED_EDGE ( 'NONE', *, *, #20931, .F. ) ;
#3289=AXIS2_PLACEMENT_3D ( 'NONE', #995, #664, #22701 ) ;
#3291=ORIENTED_EDGE ( 'NONE', *, *, #3449, .F. ) ;
#3297=CARTESIAN_POINT ( 'NONE',  ( -59.69999999999998153, 0.3248756580930906579, -3.465281767758778386 ) ) ;
#3298=CARTESIAN_POINT ( 'NONE',  ( -54.63452994616206126, -3.117691453623976816, 1.799999999999793765 ) ) ;
#3305=CARTESIAN_POINT ( 'NONE',  ( -58.24005354137801049, -3.399999999999994138, 0.9110272542655853956 ) ) ;
#3306=CARTESIAN_POINT ( 'NONE',  ( -58.44702994616205416, -2.078460969082659648, 3.599999999999782929 ) ) ;
#3319=FACE_OUTER_BOUND ( 'NONE', #18096, .T. ) ;
#3323=EDGE_LOOP ( 'NONE', ( #11808, #25670, #7534, #21347 ) ) ;
#3324=CARTESIAN_POINT ( 'NONE',  ( -56.88452994616205416, -3.117691453623976816, 1.799999999999785993 ) ) ;
#3332=( BOUNDED_CURVE ( )  B_SPLINE_CURVE ( 2, ( #7629, #10156, #18939, #19824, #645, #29455, #29319, #12361, #12673 ),
 .UNSPECIFIED., .F., .T. ) 
 B_SPLINE_CURVE_WITH_KNOTS ( ( 3, 2, 2, 2, 3 ),
 ( 0.3611111111111111605, 0.3703703703703703498, 0.3888888888888888951, 0.4074074074074073848, 0.4166666666666666852 ),
 .UNSPECIFIED. ) 
 CURVE ( )  GEOMETRIC_REPRESENTATION_ITEM ( )  RATIONAL_B_SPLINE_CURVE ( ( 0.9330127018922194093, 0.9330127018922197424, 1.000000000000000000, 0.8660254037844387076, 1.000000000000000000, 0.8660254037844387076, 1.000000000000000000, 0.9330127018922191873, 0.9330127018922194093 ) ) 
 REPRESENTATION_ITEM ( '' )  );
#3336=EDGE_CURVE ( 'NONE', #7185, #19715, #17395, .T. ) ;
#3337=CARTESIAN_POINT ( 'NONE',  ( -54.39999999999997726, -4.766731106216463600E-14, -1.831402436016377855E-13 ) ) ;
#3343=CARTESIAN_POINT ( 'NONE',  ( -55.02900635094608361, 3.400000000000004352, 0.9110272542656342454 ) ) ;
#3344=VECTOR ( 'NONE', #22872, 1000.000000000000000 ) ;
#3352=CARTESIAN_POINT ( 'NONE',  ( -59.67193011664021185, 2.054846984738300186, 1.719925937563907548 ) ) ;
#3374=CARTESIAN_POINT ( 'NONE',  ( -61.13452994616202574, 2.093608279459375190E-14, -3.600000000000216804 ) ) ;
#3378=DIRECTION ( 'NONE',  ( 2.265029845352616032E-44, -1.000000000000000000, -3.491481338843140061E-15 ) ) ;
#3384=CARTESIAN_POINT ( 'NONE',  ( -58.56249999999997868, -1.962990915244731793, 3.399999999999783640 ) ) ;
#3390=CARTESIAN_POINT ( 'NONE',  ( -54.49999999999999289, -1.400000000000007017, 3.959797974644449603 ) ) ;
#3396=CARTESIAN_POINT ( 'NONE',  ( -59.59999999999997300, 2.337126060168390307, -1.249136413240100607 ) ) ;
#3413=CARTESIAN_POINT ( 'NONE',  ( -56.18749999999997158, -3.925981830489445379, -2.137374967025826226E-13 ) ) ;
#3417=ORIENTED_EDGE ( 'NONE', *, *, #15374, .T. ) ;
#3419=VERTEX_POINT ( 'NONE', #14051 ) ;
#3421=VERTEX_POINT ( 'NONE', #16433 ) ;
#3427=CARTESIAN_POINT ( 'NONE',  ( -44.49999999999996447, -1.399999999999981037, -3.363870538531656518 ) ) ;
#3428=CARTESIAN_POINT ( 'NONE',  ( -59.95655989232412963, 1.962990915244722245, 3.399999999999794742 ) ) ;
#3446=CARTESIAN_POINT ( 'NONE',  ( -59.19999999999996732, -2.580747833305891970, -0.9498634748674686934 ) ) ;
#3449=EDGE_CURVE ( 'NONE', #11045, #19715, #20242, .T. ) ;
#3451=B_SPLINE_CURVE_WITH_KNOTS ( 'NONE', 3,
 ( #10380, #27946, #25101, #20064, #896, #6261, #5639 ),
 .UNSPECIFIED., .F., .F.,
 ( 4, 3, 4 ),
 ( 0.000000000000000000, 3.139320973900864084E-05, 4.461998577547471821E-05 ),
 .UNSPECIFIED. ) ;
#3459=CARTESIAN_POINT ( 'NONE',  ( -44.49999999999999289, -1.400000000000004574, 3.363870538531273269 ) ) ;
#3470=EDGE_CURVE ( 'NONE', #11984, #12035, #23081, .T. ) ;
#3474=CARTESIAN_POINT ( 'NONE',  ( -57.25952994616203995, 3.117691453623998576, -1.800000000000181899 ) ) ;
#3481=DIRECTION ( 'NONE',  ( 0.000000000000000000, 1.000000000000000000, 3.491481338843130594E-15 ) ) ;
#3489=DIRECTION ( 'NONE',  ( -1.163827112947670229E-15, 0.9428090415820664649, 0.3333333333333248771 ) ) ;
#3491=CARTESIAN_POINT ( 'NONE',  ( -59.82202994616204705, -4.156921938165296204, -2.272478542645976661E-13 ) ) ;
#3493=( BOUNDED_CURVE ( )  B_SPLINE_CURVE ( 2, ( #6525, #27899, #25515, #8722, #25834, #20939, #30569, #23169, #8880, #13472, #28220, #16185, #8578, #1453, #4141, #13778, #23461, #11111, #11423, #18728, #21113, #30751, #8427, #6067, #15720, #3673, #13309, #23001, #10956, #20644, #18260, #15499, #20422, #25311, #30047, #27690, #19943, #15183, #24685, #10893, #20272, #5840, #8212, #17880, #18206, #25156, #3474, #22944, #29902, #8362, #12956, #27371, #15024, #12791, #22471, #17730, #20582, #13114, #12641, #18044, #3621, #10740, #30217, #7897, #6009, #3306, #27515, #5682, #22649, #22803, #8064, #15663, #29578, #945, #15332, #24981, #8524, #10595, #1090, #17573, #5531, #5363, #3150 ),
 .UNSPECIFIED., .F., .T. ) 
 B_SPLINE_CURVE_WITH_KNOTS ( ( 3, 2, 2, 2, 2, 2, 2, 2, 2, 2, 2, 2, 2, 2, 2, 2, 2, 2, 2, 2, 2, 2, 2, 2, 2, 2, 2, 2, 2, 2, 2, 2, 2, 2, 2, 2, 2, 2, 2, 2, 2, 3 ),
 ( 0.01191687898796012397, 0.01851851851851851749, 0.03703703703703703498, 0.05555555555555555941, 0.07407407407407406996, 0.09259259259259258745, 0.1111111111111111049, 0.1296296296296296224, 0.1481481481481481399, 0.1666666666666666574, 0.1851851851851851749, 0.2037037037037037202, 0.2222222222222222099, 0.2407407407407407274, 0.2592592592592593004, 0.2777777777777777901, 0.2962962962962962798, 0.3148148148148148251, 0.3333333333333333148, 0.3518518518518518601, 0.3703703703703703498, 0.3888888888888888951, 0.4074074074074073293, 0.4259259259259259855, 0.4444444444444444198, 0.4629629629629629650, 0.4814814814814814548, 0.5000000000000000000, 0.5185185185185184897, 0.5370370370370370905, 0.5555555555555555802, 0.5740740740740740700, 0.5925925925925925597, 0.6111111111111111605, 0.6296296296296296502, 0.6481481481481481399, 0.6666666666666666297, 0.6851851851851852304, 0.7037037037037037202, 0.7222222222222220989, 0.7407407407407408106, 0.7438073466758352570 ),
 .UNSPECIFIED. ) 
 CURVE ( )  GEOMETRIC_REPRESENTATION_ITEM ( )  RATIONAL_B_SPLINE_CURVE ( ( 0.9385312603869460091, 0.9522395925147686402, 1.000000000000000000, 0.8660254037844387076, 1.000000000000000000, 0.8660254037844387076, 1.000000000000000000, 0.8660254037844387076, 1.000000000000000000, 0.8660254037844387076, 1.000000000000000000, 0.8660254037844387076, 1.000000000000000000, 0.8660254037844387076, 1.000000000000000000, 0.8660254037844387076, 1.000000000000000000, 0.8660254037844387076, 1.000000000000000000, 0.8660254037844387076, 1.000000000000000000, 0.8660254037844387076, 1.000000000000000000, 0.8660254037844387076, 1.000000000000000000, 0.8660254037844387076, 1.000000000000000000, 0.8660254037844387076, 1.000000000000000000, 0.8660254037844387076, 1.000000000000000000, 0.8660254037844387076, 1.000000000000000000, 0.8660254037844387076, 1.000000000000000000, 0.8660254037844387076, 1.000000000000000000, 0.8660254037844387076, 1.000000000000000000, 0.8660254037844387076, 1.000000000000000000, 0.8660254037844387076, 1.000000000000000000, 0.8660254037844387076, 1.000000000000000000, 0.8660254037844387076, 1.000000000000000000, 0.8660254037844387076, 1.000000000000000000, 0.8660254037844387076, 1.000000000000000000, 0.8660254037844387076, 1.000000000000000000, 0.8660254037844387076, 1.000000000000000000, 0.8660254037844387076, 1.000000000000000000, 0.8660254037844387076, 1.000000000000000000, 0.8660254037844387076, 1.000000000000000000, 0.8660254037844387076, 1.000000000000000000, 0.8660254037844387076, 1.000000000000000000, 0.8660254037844387076, 1.000000000000000000, 0.8660254037844387076, 1.000000000000000000, 0.8660254037844387076, 1.000000000000000000, 0.8660254037844387076, 1.000000000000000000, 0.8660254037844387076, 1.000000000000000000, 0.8660254037844387076, 1.000000000000000000, 0.8660254037844387076, 1.000000000000000000, 0.8660254037844387076, 1.000000000000000000, 0.9778142462370478238, 0.9629762686038090269 ) ) 
 REPRESENTATION_ITEM ( '' )  );
#3499=CARTESIAN_POINT ( 'NONE',  ( -60.32202994616201863, 2.078460969082674747, -3.600000000000205258 ) ) ;
#3513=DIRECTION ( 'NONE',  ( -1.000000000000000000, 1.219044193948983948E-29, -3.491481338843133355E-15 ) ) ;
#3535=CARTESIAN_POINT ( 'NONE',  ( -59.82202994616204705, -4.156921938165296204, -2.272478542645976661E-13 ) ) ;
#3541=CARTESIAN_POINT ( 'NONE',  ( -57.81249999999998579, -1.962990915244731793, 3.399999999999786304 ) ) ;
#3550=CARTESIAN_POINT ( 'NONE',  ( -59.62735476476905205, 2.346806195053369848, -1.237686616523536287 ) ) ;
#3562=ORIENTED_EDGE ( 'NONE', *, *, #16812, .F. ) ;
#3565=CARTESIAN_POINT ( 'NONE',  ( -58.62499999999998579, -3.920666489018310435E-15, 3.399999999999791189 ) ) ;
#3566=CARTESIAN_POINT ( 'NONE',  ( -59.49223166990491762, 2.264560344927355917, 1.390271221205179986 ) ) ;
#3568=VERTEX_POINT ( 'NONE', #19300 ) ;
#3571=CARTESIAN_POINT ( 'NONE',  ( -59.19999999999996732, 2.580747833305914618, -0.9498634748674507078 ) ) ;
#3575=CARTESIAN_POINT ( 'NONE',  ( -59.18749999999995737, -3.399999999999991029, -2.288065396424332102E-13 ) ) ;
#3577=CARTESIAN_POINT ( 'NONE',  ( -58.20655989232411542, -3.925981830489445379, -2.207870066386390016E-13 ) ) ;
#3601=VERTEX_POINT ( 'NONE', #28936 ) ;
#3612=VERTEX_POINT ( 'NONE', #2504 ) ;
#3614=CIRCLE ( 'NONE', #25350, 2.750000000000000000 ) ;
#3620=CARTESIAN_POINT ( 'NONE',  ( -58.26905989232412253, -2.944486372867094914, 1.699999999999771472 ) ) ;
#3621=CARTESIAN_POINT ( 'NONE',  ( -58.13452994616202574, 3.813458051520598461E-14, -3.600000000000206146 ) ) ;
#3628=CARTESIAN_POINT ( 'NONE',  ( -59.11195455104547136, 2.468319916663101576, -0.9648999906351578559 ) ) ;
#3629=FACE_OUTER_BOUND ( 'NONE', #22604, .T. ) ;
#3635=DIRECTION ( 'NONE',  ( -1.000000000000000000, 1.219044193948983948E-29, -3.491481338843133355E-15 ) ) ;
#3640=CARTESIAN_POINT ( 'NONE',  ( -59.39944685111014877, 2.372743686651884953, 1.252203205371202666 ) ) ;
#3643=CARTESIAN_POINT ( 'NONE',  ( -60.25952994616203284, 3.117691453623994580, -1.800000000000200329 ) ) ;
#3648=CARTESIAN_POINT ( 'NONE',  ( -54.39999999999996305, -1.433333333333312254, -4.054078878803088593 ) ) ;
#3654=CARTESIAN_POINT ( 'NONE',  ( -44.59999999999997300, -4.766731106216475591E-14, -1.489237264809750408E-13 ) ) ;
#3660=CARTESIAN_POINT ( 'NONE',  ( -44.49999999999997868, 8.366749974758366115E-15, -1.867384948185803131E-13 ) ) ;
#3667=ORIENTED_EDGE ( 'NONE', *, *, #24173, .T. ) ;
#3673=CARTESIAN_POINT ( 'NONE',  ( -55.94702994616203995, -2.078460969082627230, -3.600000000000206590 ) ) ;
#3674=CARTESIAN_POINT ( 'NONE',  ( -59.14405989232412963, -3.920666489018302546E-15, 3.399999999999788969 ) ) ;
#3678=CARTESIAN_POINT ( 'NONE',  ( -57.43749999999996447, 1.962990915244749557, -3.400000000000195310 ) ) ;
#3687=B_SPLINE_CURVE_WITH_KNOTS ( 'NONE', 3,
 ( #13294, #23303, #30735, #20925 ),
 .UNSPECIFIED., .F., .F.,
 ( 4, 4 ),
 ( 0.000000000000000000, 3.288265101740379156E-05 ),
 .UNSPECIFIED. ) ;
#3694=CARTESIAN_POINT ( 'NONE',  ( -59.48573950359912743, 3.423031164920794289, -1.114835254188495162 ) ) ;
#3700=CARTESIAN_POINT ( 'NONE',  ( -56.81249999999997158, -1.962990915244707368, -3.400000000000208633 ) ) ;
#3703=AXIS2_PLACEMENT_3D ( 'NONE', #27561, #15705, #6053 ) ;
#3715=CARTESIAN_POINT ( 'NONE',  ( -60.64405989232412253, -3.920666489018283614E-15, 3.399999999999783640 ) ) ;
#3722=CYLINDRICAL_SURFACE ( 'NONE', #15409, 3.399999999999999911 ) ;
#3731=CARTESIAN_POINT ( 'NONE',  ( -59.38263816597098099, 3.123852333407923787, -1.389329043195103752 ) ) ;
#3752=CARTESIAN_POINT ( 'NONE',  ( -44.49999999999997868, 8.366749974758269874E-15, -1.589829192029513996E-13 ) ) ;
#3761=CIRCLE ( 'NONE', #4786, 0.1000000000000000472 ) ;
#3790=EDGE_CURVE ( 'NONE', #11190, #29758, #4787, .T. ) ;
#3791=CARTESIAN_POINT ( 'NONE',  ( -61.13452994616202574, 2.093608279459375190E-14, -3.600000000000216804 ) ) ;
#3798=DIRECTION ( 'NONE',  ( 0.000000000000000000, -1.000000000000000000, -4.336808689942015369E-15 ) ) ;
#3800=AXIS2_PLACEMENT_3D ( 'NONE', #1579, #9352, #28351 ) ;
#3801=CARTESIAN_POINT ( 'NONE',  ( -54.49999999999999289, -1.400000000000007017, 4.029888335921757658 ) ) ;
#3804=CIRCLE ( 'NONE', #8860, 0.1000000000000000472 ) ;
#3806=DIRECTION ( 'NONE',  ( 2.265029845352616032E-44, -1.000000000000000000, -3.491481338843140061E-15 ) ) ;
#3810=FACE_OUTER_BOUND ( 'NONE', #12170, .T. ) ;
#3827=CARTESIAN_POINT ( 'NONE',  ( -57.20655989232410832, 1.962990915244748891, -3.400000000000194422 ) ) ;
#3828=EDGE_LOOP ( 'NONE', ( #23113, #13981, #14538, #25545 ) ) ;
#3833=CARTESIAN_POINT ( 'NONE',  ( -57.68749999999996447, -3.925981830489445379, -2.189747187108473037E-13 ) ) ;
#3846=DIRECTION ( 'NONE',  ( 0.000000000000000000, -1.000000000000000000, -3.491481338843130594E-15 ) ) ;
#3851=DIRECTION ( 'NONE',  ( 1.000000000000000000, -1.219044193948983948E-29, 3.491481338843133355E-15 ) ) ;
#3861=CARTESIAN_POINT ( 'NONE',  ( -55.12499999999997158, 2.944486372867106905, -1.700000000000183364 ) ) ;
#3865=ORIENTED_EDGE ( 'NONE', *, *, #9634, .T. ) ;
#3872=CARTESIAN_POINT ( 'NONE',  ( -59.59999999999997300, -2.337126060168364994, -1.249136413240117038 ) ) ;
#3873=CYLINDRICAL_SURFACE ( 'NONE', #8606, 2.649999999999999911 ) ;
#3891=EDGE_CURVE ( 'NONE', #14560, #10413, #6245, .T. ) ;
#3910=EDGE_CURVE ( 'NONE', #14828, #5117, #7265, .T. ) ;
#3914=CARTESIAN_POINT ( 'NONE',  ( -55.95655989232413674, -3.399999999999990585, -2.144552914728849773E-13 ) ) ;
#3921=DIRECTION ( 'NONE',  ( 0.000000000000000000, 1.000000000000000000, 4.336808689942015369E-15 ) ) ;
#3925=CARTESIAN_POINT ( 'NONE',  ( -57.00952994616205416, -4.643455692769903542E-15, 3.599999999999796696 ) ) ;
#3928=AXIS2_PLACEMENT_3D ( 'NONE', #21061, #3635, #28165 ) ;
#3930=EDGE_CURVE ( 'NONE', #12969, #26147, #10284, .T. ) ;
#3937=CARTESIAN_POINT ( 'NONE',  ( -54.49999999999997868, 3.624999999999963585, -2.089966883537054476E-13 ) ) ;
#3948=EDGE_LOOP ( 'NONE', ( #3291, #7536, #24172, #10290, #12318 ) ) ;
#3952=CARTESIAN_POINT ( 'NONE',  ( -59.40743313238012036, 2.395752775956333291, 1.250136525132548027 ) ) ;
#3955=ORIENTED_EDGE ( 'NONE', *, *, #25501, .F. ) ;
#3974=CARTESIAN_POINT ( 'NONE',  ( -59.60675767627768096, -2.338930541566021759, -1.245993773302377816 ) ) ;
#3982=EDGE_LOOP ( 'NONE', ( #16502, #9555, #23547, #29036 ) ) ;
#3987=CARTESIAN_POINT ( 'NONE',  ( -56.01905989232412963, -2.944486372867088697, 1.699999999999789679 ) ) ;
#3994=CIRCLE ( 'NONE', #4994, 0.1000000000000000472 ) ;
#3995=CARTESIAN_POINT ( 'NONE',  ( -57.99999999999997868, 2.944486372867092250, 1.699999999999805667 ) ) ;
#3996=CARTESIAN_POINT ( 'NONE',  ( -54.83155989232413674, 3.400000000000008349, -1.845326485282803322E-13 ) ) ;
#3998=CARTESIAN_POINT ( 'NONE',  ( -57.45655989232412253, -3.399999999999991029, -2.148039047887444390E-13 ) ) ;
#4001=CARTESIAN_POINT ( 'NONE',  ( -59.09999999999997300, 2.465712773623992327, -0.9709585562669131864 ) ) ;
#4015=AXIS2_PLACEMENT_3D ( 'NONE', #27264, #14906, #5582 ) ;
#4019=CARTESIAN_POINT ( 'NONE',  ( -59.06249999999995737, -1.962990915244707368, -3.400000000000216627 ) ) ;
#4029=PLANE ( 'NONE',  #20658 ) ;
#4030=CARTESIAN_POINT ( 'NONE',  ( -54.39999999999999147, -1.500000000000006661, 3.959797974644449603 ) ) ;
#4034=LINE ( 'NONE', #29999, #8663 ) ;
#4064=VERTEX_POINT ( 'NONE', #20627 ) ;
#4067=DIRECTION ( 'NONE',  ( 1.000000000000000000, -1.219044193948984088E-29, 3.491481338843133750E-15 ) ) ;
#4072=EDGE_CURVE ( 'NONE', #7915, #17824, #24438, .T. ) ;
#4079=CARTESIAN_POINT ( 'NONE',  ( -57.57202994616204705, -4.156921938165296204, -2.193920212522006445E-13 ) ) ;
#4090=CARTESIAN_POINT ( 'NONE',  ( -56.99999999999997158, -2.944486372867094470, 1.699999999999777689 ) ) ;
#4098=CARTESIAN_POINT ( 'NONE',  ( -59.67987798884426809, -2.349476376206443007, -1.226921160904901109 ) ) ;
#4100=CARTESIAN_POINT ( 'NONE',  ( -60.75952994616205416, -4.643455692769856999E-15, 3.599999999999783373 ) ) ;
#4108=DIRECTION ( 'NONE',  ( 1.000000000000000000, -1.219044193948983948E-29, 3.491481338843133355E-15 ) ) ;
#4113=CARTESIAN_POINT ( 'NONE',  ( -59.40362242792826919, 3.375967812128700452, 1.250136525132546916 ) ) ;
#4121=CARTESIAN_POINT ( 'NONE',  ( -44.59999999999998010, 2.650000000000008349, -1.759412204284508433E-13 ) ) ;
#4122=CARTESIAN_POINT ( 'NONE',  ( -59.60996874016036173, 2.024041967860128910, 1.710882463691307143 ) ) ;
#4141=CARTESIAN_POINT ( 'NONE',  ( -55.25952994616203995, -3.117691453623963049, -1.800000000000208544 ) ) ;
#4143=CARTESIAN_POINT ( 'NONE',  ( -58.76905989232410832, 2.023778652682509368E-14, -3.400000000000208189 ) ) ;
#4146=CIRCLE ( 'NONE', #21873, 2.649999999999999911 ) ;
#4148=CARTESIAN_POINT ( 'NONE',  ( -55.82202994616203995, 2.078460969082674747, -3.600000000000189715 ) ) ;
#4168=CARTESIAN_POINT ( 'NONE',  ( -55.75952994616203995, 3.117691453623994580, -1.800000000000184563 ) ) ;
#4174=ADVANCED_FACE ( 'NONE', ( #985 ), #10638, .T. ) ;
#4180=CARTESIAN_POINT ( 'NONE',  ( -54.47064643025908737, -2.407416487588556198, -2.678616765879081374 ) ) ;
#4186=ORIENTED_EDGE ( 'NONE', *, *, #4570, .F. ) ;
#4187=FACE_OUTER_BOUND ( 'NONE', #22497, .T. ) ;
#4208=DIRECTION ( 'NONE',  ( 0.000000000000000000, -1.000000000000000000, 0.000000000000000000 ) ) ;
#4213=DIRECTION ( 'NONE',  ( 1.000000000000000000, -1.219044193948983948E-29, 3.491481338843133355E-15 ) ) ;
#4222=CARTESIAN_POINT ( 'NONE',  ( -59.41132486539680713, 3.361433066165957051, 1.250136525132557574 ) ) ;
#4225=CARTESIAN_POINT ( 'NONE',  ( -56.25952994616206126, -4.643455692769913008E-15, 3.599999999999798916 ) ) ;
#4271=CARTESIAN_POINT ( 'NONE',  ( -59.61691039550309767, 2.025699712120192064, 1.710375399846320255 ) ) ;
#4285=ORIENTED_EDGE ( 'NONE', *, *, #12706, .F. ) ;
#4291=FILL_AREA_STYLE_COLOUR ( '', #31325 ) ;
#4293=CARTESIAN_POINT ( 'NONE',  ( -57.39405989232411542, -2.944486372867076263, -1.700000000000214451 ) ) ;
#4298=CARTESIAN_POINT ( 'NONE',  ( -56.00952994616203995, -3.117691453623963938, -1.800000000000210099 ) ) ;
#4300=CARTESIAN_POINT ( 'NONE',  ( -54.39999999999996305, -1.499999999999978906, -3.959797974644881258 ) ) ;
#4306=FACE_OUTER_BOUND ( 'NONE', #17084, .T. ) ;
#4323=CARTESIAN_POINT ( 'NONE',  ( -61.12499999999995737, 2.944486372867106905, -1.700000000000204459 ) ) ;
#4329=AXIS2_PLACEMENT_3D ( 'NONE', #28499, #21246, #18542 ) ;
#4332=FACE_OUTER_BOUND ( 'NONE', #1938, .T. ) ;
#4333=ORIENTED_EDGE ( 'NONE', *, *, #19570, .F. ) ;
#4336=AXIS2_PLACEMENT_3D ( 'NONE', #1053, #10704, #15296 ) ;
#4337=DIRECTION ( 'NONE',  ( 1.000000000000000000, -1.219044193948983948E-29, 3.491481338843133355E-15 ) ) ;
#4341=( BOUNDED_CURVE ( )  B_SPLINE_CURVE ( 3, ( #10055, #17189, #231, #9605 ),
 .UNSPECIFIED., .F., .T. ) 
 B_SPLINE_CURVE_WITH_KNOTS ( ( 4, 4 ),
 ( 4.339533644879389307, 4.356609821944394056 ),
 .UNSPECIFIED. ) 
 CURVE ( )  GEOMETRIC_REPRESENTATION_ITEM ( )  RATIONAL_B_SPLINE_CURVE ( ( 1.000000000000000000, 0.9999757004956882911, 0.9999757004956882911, 1.000000000000000000 ) ) 
 REPRESENTATION_ITEM ( '' )  );
#4354=LINE ( 'NONE', #18632, #29702 ) ;
#4356=AXIS2_PLACEMENT_3D ( 'NONE', #24271, #26938, #2425 ) ;
#4360=AXIS2_PLACEMENT_3D ( 'NONE', #7812, #17487, #20023 ) ;
#4371=EDGE_LOOP ( 'NONE', ( #29066, #28515, #5665 ) ) ;
#4388=CARTESIAN_POINT ( 'NONE',  ( -59.07202994616203995, -4.156921938165296204, -2.246292432604653256E-13 ) ) ;
#4398=DIRECTION ( 'NONE',  ( 0.000000000000000000, -0.4295302013423027421, 0.9030524935654852259 ) ) ;
#4399=EDGE_CURVE ( 'NONE', #30643, #15709, #9682, .T. ) ;
#4403=DIRECTION ( 'NONE',  ( 3.491481338843133355E-15, 3.491481338843133355E-15, -1.000000000000000000 ) ) ;
#4413=ORIENTED_EDGE ( 'NONE', *, *, #19873, .F. ) ;
#4415=CARTESIAN_POINT ( 'NONE',  ( -59.69457535546588645, -2.411387898320983769, -1.235406689480271103 ) ) ;
#4425=CARTESIAN_POINT ( 'NONE',  ( -55.39405989232414385, -4.753426312438548412E-15, 3.399999999999801847 ) ) ;
#4426=CARTESIAN_POINT ( 'NONE',  ( -57.74999999999997158, -2.944486372867094914, 1.699999999999774358 ) ) ;
#4430=ORIENTED_EDGE ( 'NONE', *, *, #4640, .T. ) ;
#4434=ADVANCED_FACE ( 'NONE', ( #24527 ), #14404, .F. ) ;
#4439=AXIS2_PLACEMENT_3D ( 'NONE', #23863, #30345, #8652 ) ;
#4441=DIRECTION ( 'NONE',  ( 0.000000000000000000, -1.000000000000000000, -4.336808689942015369E-15 ) ) ;
#4448=DIRECTION ( 'NONE',  ( 1.000000000000000000, -1.219044193948983948E-29, 3.491481338843133355E-15 ) ) ;
#4460=ORIENTED_EDGE ( 'NONE', *, *, #28019, .T. ) ;
#4462=DIRECTION ( 'NONE',  ( -1.000000000000000000, 1.219044193948983948E-29, -3.491481338843133355E-15 ) ) ;
#4466=ADVANCED_FACE ( 'NONE', ( #24076 ), #28977, .T. ) ;
#4467=ORIENTED_EDGE ( 'NONE', *, *, #11497, .T. ) ;
#4468=ADVANCED_FACE ( 'NONE', ( #20 ), #26603, .F. ) ;
#4469=CARTESIAN_POINT ( 'NONE',  ( -60.87499999999997158, -3.920666489018282036E-15, 3.399999999999783196 ) ) ;
#4473=FACE_OUTER_BOUND ( 'NONE', #10149, .T. ) ;
#4485=DIRECTION ( 'NONE',  ( 1.000000000000000000, -1.219044193948983948E-29, 3.491481338843133355E-15 ) ) ;
#4493=CARTESIAN_POINT ( 'NONE',  ( -59.37499999999997868, -3.920666489018300969E-15, 3.399999999999788525 ) ) ;
#4494=EDGE_LOOP ( 'NONE', ( #21455, #27286, #23573, #6104, #4186 ) ) ;
#4501=CARTESIAN_POINT ( 'NONE',  ( -56.69702994616203284, -2.078460969082631227, -3.600000000000207923 ) ) ;
#4517=FACE_OUTER_BOUND ( 'NONE', #27998, .T. ) ;
#4523=CIRCLE ( 'NONE', #22238, 2.649999999999999911 ) ;
#4539=( BOUNDED_CURVE ( )  B_SPLINE_CURVE ( 2, ( #3996, #23322, #6534, #1762, #16195, #25843, #13785, #11434, #29451 ),
 .UNSPECIFIED., .F., .T. ) 
 B_SPLINE_CURVE_WITH_KNOTS ( ( 3, 2, 2, 2, 3 ),
 ( 0.08333333333333334259, 0.09259259259259258745, 0.1111111111111111049, 0.1296296296296296224, 0.1388888888888888951 ),
 .UNSPECIFIED. ) 
 CURVE ( )  GEOMETRIC_REPRESENTATION_ITEM ( )  RATIONAL_B_SPLINE_CURVE ( ( 0.9330127018922192983, 0.9330127018922194093, 1.000000000000000000, 0.8660254037844387076, 1.000000000000000000, 0.8660254037844387076, 1.000000000000000000, 0.9330127018922191873, 0.9330127018922192983 ) ) 
 REPRESENTATION_ITEM ( '' )  );
#4542=DIRECTION ( 'NONE',  ( 0.000000000000000000, 1.000000000000000000, 3.491481338843252079E-15 ) ) ;
#4552=CARTESIAN_POINT ( 'NONE',  ( -56.75952994616203995, -3.117691453623963938, -1.800000000000212763 ) ) ;
#4553=VECTOR ( 'NONE', #17171, 1000.000000000000000 ) ;
#4559=PLANE ( 'NONE',  #7391 ) ;
#4570=EDGE_CURVE ( 'NONE', #26101, #24402, #488, .T. ) ;
#4573=CARTESIAN_POINT ( 'NONE',  ( -44.59999999999996589, -1.399999999999979039, -3.959797974644846619 ) ) ;
#4578=FACE_OUTER_BOUND ( 'NONE', #5736, .T. ) ;
#4583=EDGE_CURVE ( 'NONE', #16075, #17943, #1430, .T. ) ;
#4597=EDGE_LOOP ( 'NONE', ( #26376, #29185, #8642, #10821 ) ) ;
#4608=EDGE_CURVE ( 'NONE', #15357, #3421, #16631, .T. ) ;
#4613=ORIENTED_EDGE ( 'NONE', *, *, #14032, .F. ) ;
#4619=CARTESIAN_POINT ( 'NONE',  ( -59.49999999999997158, 2.944486372867092250, 1.699999999999800115 ) ) ;
#4622=CARTESIAN_POINT ( 'NONE',  ( -54.49999999999999289, -1.400000000000004574, 3.363870538531238186 ) ) ;
#4631=VERTEX_POINT ( 'NONE', #26096 ) ;
#4640=EDGE_CURVE ( 'NONE', #20201, #3601, #15751, .T. ) ;
#4646=CARTESIAN_POINT ( 'NONE',  ( -59.18749999999996447, -3.925981830489445379, -2.242119407191119848E-13 ) ) ;
#4654=CARTESIAN_POINT ( 'NONE',  ( -58.25952994616203284, -3.117691453623963938, -1.800000000000218092 ) ) ;
#4660=DIRECTION ( 'NONE',  ( -3.491481338843133355E-15, -3.491481338843133355E-15, 1.000000000000000000 ) ) ;
#4674=CARTESIAN_POINT ( 'NONE',  ( -59.15690588169601227, -2.360521237243748072, 1.241563447891223859 ) ) ;
#4678=CIRCLE ( 'NONE', #24396, 0.1000000000000000472 ) ;
#4682=VERTEX_POINT ( 'NONE', #23268 ) ;
#4696=CARTESIAN_POINT ( 'NONE',  ( -60.07202994616204705, 2.078460969082646770, 3.599999999999794031 ) ) ;
#4701=CYLINDRICAL_SURFACE ( 'NONE', #6898, 3.399999999999999911 ) ;
#4704=CARTESIAN_POINT ( 'NONE',  ( -59.09999999999997300, 8.366749974758448157E-15, -2.099585467500611340E-13 ) ) ;
#4711=CARTESIAN_POINT ( 'NONE',  ( -57.62499999999996447, -2.944486372867072710, -1.700000000000221334 ) ) ;
#4718=EDGE_LOOP ( 'NONE', ( #174, #16253, #6562, #13548 ) ) ;
#4746=DIRECTION ( 'NONE',  ( 3.491481338843133355E-15, 3.491481338843133355E-15, -1.000000000000000000 ) ) ;
#4749=ADVANCED_FACE ( 'NONE', ( #26413 ), #17230, .T. ) ;
#4756=MANIFOLD_SOLID_BREP ( 'Stock-MAS-683-1', #4905 ) ;
#4764=CARTESIAN_POINT ( 'NONE',  ( -54.39999999999996305, 1.600000000000021627, -3.363870538531679610 ) ) ;
#4768=CARTESIAN_POINT ( 'NONE',  ( -55.38452994616205416, -3.117691453623976816, 1.799999999999791100 ) ) ;
#4786=AXIS2_PLACEMENT_3D ( 'NONE', #921, #10407, #20401 ) ;
#4787=LINE ( 'NONE', #8906, #1711 ) ;
#4795=CIRCLE ( 'NONE', #23514, 2.750000000000000000 ) ;
#4797=CARTESIAN_POINT ( 'NONE',  ( -56.69702994616203284, -2.078460969082631227, -3.600000000000207923 ) ) ;
#4803=CARTESIAN_POINT ( 'NONE',  ( -56.94702994616206126, -2.078460969082657872, 3.599999999999789591 ) ) ;
#4813=AXIS2_PLACEMENT_3D ( 'NONE', #1178, #20518, #25248 ) ;
#4828=VECTOR ( 'NONE', #28314, 1000.000000000000000 ) ;
#4835=CARTESIAN_POINT ( 'NONE',  ( -54.49999999999997868, 8.366749974758391359E-15, -1.938977325913827332E-13 ) ) ;
#4847=VERTEX_POINT ( 'NONE', #916 ) ;
#4851=CARTESIAN_POINT ( 'NONE',  ( -55.39405989232414385, -3.920666489018348300E-15, 3.399999999999801847 ) ) ;
#4856=AXIS2_PLACEMENT_3D ( 'NONE', #28859, #26634, #7171 ) ;
#4863=AXIS2_PLACEMENT_3D ( 'NONE', #29333, #21923, #202 ) ;
#4905=CLOSED_SHELL ( 'NONE', ( #16569, #14887, #7630, #18173, #29915, #14900, #25480, #971, #3104, #4749, #6069, #18994, #27414, #14476, #17598, #6299, #29577, #9466, #16673, #23950, #30272, #24587, #24972, #24022, #14387, #8811, #1780, #30895, #23989, #18516, #15614, #24209, #15044, #8851, #22821, #4434, #27075, #4466, #29355, #7194, #13533, #14774, #4468, #19070, #22025, #11347, #7135, #26636, #27703, #17566, #22039, #904, #12240, #12061, #1344, #17033, #15188, #8331, #24932, #27519, #25159, #20464, #26612, #9484, #7711, #8771, #17359, #28125, #7481, #16274, #17305, #15132, #12604, #7704, #5784, #23294, #17435, #13081, #24680, #25048, #4174, #8879, #2970, #27983, #17950, #25120, #13264, #20665, #12324, #25310, #8848, #26626, #15233, #31214, #12937, #21898, #10590 ) ) ;
#4915=DIRECTION ( 'NONE',  ( -3.491481338843133355E-15, -3.491481338843133355E-15, 1.000000000000000000 ) ) ;
#4924=AXIS2_PLACEMENT_3D ( 'NONE', #28451, #31133, #4542 ) ;
#4927=ORIENTED_EDGE ( 'NONE', *, *, #4985, .T. ) ;
#4929=CIRCLE ( 'NONE', #3928, 3.625000000000024869 ) ;
#4937=CARTESIAN_POINT ( 'NONE',  ( -59.32202994616204705, 2.078460969082646770, 3.599999999999797140 ) ) ;
#4946=CIRCLE ( 'NONE', #908, 3.625000000000024869 ) ;
#4952=ORIENTED_EDGE ( 'NONE', *, *, #2601, .T. ) ;
#4964=CARTESIAN_POINT ( 'NONE',  ( -57.07202994616206126, 2.078460969082646770, 3.599999999999804690 ) ) ;
#4971=CARTESIAN_POINT ( 'NONE',  ( -55.88452994616203995, 2.093608279459368564E-14, -3.600000000000198597 ) ) ;
#4979=EDGE_CURVE ( 'NONE', #19242, #9490, #7807, .T. ) ;
#4984=CARTESIAN_POINT ( 'NONE',  ( -59.62499999999996447, 2.944486372867118895, -1.700000000000178924 ) ) ;
#4985=EDGE_CURVE ( 'NONE', #14659, #6036, #9850, .T. ) ;
#4994=AXIS2_PLACEMENT_3D ( 'NONE', #9720, #28398, #16362 ) ;
#4998=CARTESIAN_POINT ( 'NONE',  ( -54.62499999999997158, -2.944486372867076707, -1.700000000000204903 ) ) ;
#5001=EDGE_CURVE ( 'NONE', #20368, #25749, #26565, .T. ) ;
#5009=EDGE_LOOP ( 'NONE', ( #28883, #14456, #9053, #30097 ) ) ;
#5013=CARTESIAN_POINT ( 'NONE',  ( -55.01905989232411542, 2.023778652682504950E-14, -3.400000000000195310 ) ) ;
#5016=( GEOMETRIC_REPRESENTATION_CONTEXT ( 3 ) GLOBAL_UNCERTAINTY_ASSIGNED_CONTEXT ( ( #7287 ) ) GLOBAL_UNIT_ASSIGNED_CONTEXT ( ( #16339, #1753, #16184 ) ) REPRESENTATION_CONTEXT ( 'NONE', 'WORKASPACE' ) );
#5042=CARTESIAN_POINT ( 'NONE',  ( -54.39999999999996305, -1.399999999999981037, -3.363870538531691157 ) ) ;
#5054=CARTESIAN_POINT ( 'NONE',  ( -58.02900635094607651, 3.400000000000002576, 0.9110272542656318029 ) ) ;
#5063=CARTESIAN_POINT ( 'NONE',  ( -59.42113335569190014, 3.317668011003051642, -1.077534877302829264 ) ) ;
#5093=CARTESIAN_POINT ( 'NONE',  ( -59.50952994616202574, 3.117691453623994580, -1.800000000000197664 ) ) ;
#5112=ORIENTED_EDGE ( 'NONE', *, *, #11080, .F. ) ;
#5116=CARTESIAN_POINT ( 'NONE',  ( -59.37009172985672478, 3.234433134214944161, -1.048065980887175952 ) ) ;
#5117=VERTEX_POINT ( 'NONE', #6395 ) ;
#5122=CARTESIAN_POINT ( 'NONE',  ( -55.38452994616205416, -3.117691453623976816, 1.799999999999791100 ) ) ;
#5124=CARTESIAN_POINT ( 'NONE',  ( -56.31249999999998579, -1.962990915244736678, 3.399999999999788969 ) ) ;
#5135=CARTESIAN_POINT ( 'NONE',  ( -44.49999999999999289, -1.400000000000007017, 3.959797974644484242 ) ) ;
#5158=ORIENTED_EDGE ( 'NONE', *, *, #13644, .F. ) ;
#5160=DIRECTION ( 'NONE',  ( 1.000000000000000000, -1.219044193948983948E-29, 3.491481338843133355E-15 ) ) ;
#5163=CARTESIAN_POINT ( 'NONE',  ( -55.14405989232412253, -2.944486372867076263, -1.700000000000206235 ) ) ;
#5166=CARTESIAN_POINT ( 'NONE',  ( -58.81249999999996447, 3.400000000000008349, -1.915049148454697437E-13 ) ) ;
#5174=VECTOR ( 'NONE', #10057, 1000.000000000000000 ) ;
#5191=CARTESIAN_POINT ( 'NONE',  ( -59.69999999999997442, 2.444843547360534775, -1.238538609462265905 ) ) ;
#5206=EDGE_CURVE ( 'NONE', #9375, #20708, #13336, .T. ) ;
#5208=FACE_OUTER_BOUND ( 'NONE', #18727, .T. ) ;
#5234=CARTESIAN_POINT ( 'NONE',  ( -59.63452994616203284, 2.093608279459373297E-14, -3.600000000000211475 ) ) ;
#5242=CARTESIAN_POINT ( 'NONE',  ( -58.58155989232410832, 3.400000000000007905, -1.908076882137507950E-13 ) ) ;
#5249=ORIENTED_EDGE ( 'NONE', *, *, #10781, .F. ) ;
#5267=CARTESIAN_POINT ( 'NONE',  ( -55.14405989232412253, -2.944486372867076263, -1.700000000000206235 ) ) ;
#5270=FACE_OUTER_BOUND ( 'NONE', #10710, .T. ) ;
#5290=CARTESIAN_POINT ( 'NONE',  ( -59.15580762875987375, 2.348892103289441202, 1.260680929859216537 ) ) ;
#5303=CARTESIAN_POINT ( 'NONE',  ( -57.39405989232411542, -2.944486372867072710, -1.700000000000220446 ) ) ;
#5307=CARTESIAN_POINT ( 'NONE',  ( -60.25952994616203284, 3.117691453623994580, -1.800000000000200329 ) ) ;
#5314=CARTESIAN_POINT ( 'NONE',  ( -59.19126343180466421, -2.406052454186071277, 1.245092465133171844 ) ) ;
#5332=CARTESIAN_POINT ( 'NONE',  ( -57.83155989232412253, 3.400000000000007905, -1.837192174579415376E-13 ) ) ;
#5334=ORIENTED_EDGE ( 'NONE', *, *, #27663, .T. ) ;
#5335=CARTESIAN_POINT ( 'NONE',  ( -58.17306624327022746, -3.399999999999988365, -0.9110272542660463602 ) ) ;
#5336=CARTESIAN_POINT ( 'NONE',  ( -59.69142724121850563, 2.412383461849218591, -1.233589124872089826 ) ) ;
#5341=AXIS2_PLACEMENT_3D ( 'NONE', #303, #24376, #7139 ) ;
#5345=CARTESIAN_POINT ( 'NONE',  ( -59.69999999999997442, 0.8751759519302413359, -3.334367871151324714 ) ) ;
#5356=EDGE_CURVE ( 'NONE', #16069, #17883, #25759, .T. ) ;
#5363=CARTESIAN_POINT ( 'NONE',  ( -59.39369649845482257, 3.270110022916793646, 1.536003293967694860 ) ) ;
#5377=ORIENTED_EDGE ( 'NONE', *, *, #15516, .T. ) ;
#5379=CARTESIAN_POINT ( 'NONE',  ( -59.27703510351125260, 3.069728509726986854, 1.483074255709971867 ) ) ;
#5384=AXIS2_PLACEMENT_3D ( 'NONE', #26806, #26948, #17622 ) ;
#5397=AXIS2_PLACEMENT_3D ( 'NONE', #6996, #4915, #17124 ) ;
#5398=CARTESIAN_POINT ( 'NONE',  ( -57.13452994616205416, 3.117691453623979481, 1.799999999999809086 ) ) ;
#5401=DIRECTION ( 'NONE',  ( -1.000000000000000000, 1.219044193948983948E-29, -3.491481338843133355E-15 ) ) ;
#5406=DIRECTION ( 'NONE',  ( 1.000000000000000000, -1.219044193948983948E-29, 3.491481338843133355E-15 ) ) ;
#5437=CARTESIAN_POINT ( 'NONE',  ( -60.82202994616204705, 2.078460969082646770, 3.599999999999791367 ) ) ;
#5482=CARTESIAN_POINT ( 'NONE',  ( -57.58155989232413674, -1.962990915244731571, 3.399999999999786748 ) ) ;
#5491=DIRECTION ( 'NONE',  ( 0.000000000000000000, -1.000000000000000000, -3.491481338843252079E-15 ) ) ;
#5493=VERTEX_POINT ( 'NONE', #25630 ) ;
#5499=CARTESIAN_POINT ( 'NONE',  ( -44.59999999999997300, 8.366749974758367693E-15, -1.870876429524646202E-13 ) ) ;
#5500=VERTEX_POINT ( 'NONE', #20894 ) ;
#5506=CARTESIAN_POINT ( 'NONE',  ( -59.19999999999997442, 2.395752775956333291, 1.250136525132548693 ) ) ;
#5517=TOROIDAL_SURFACE ( 'NONE', #9038, 2.750000000000000000, 0.1000000000000000056 ) ;
#5520=( BOUNDED_CURVE ( )  B_SPLINE_CURVE ( 3, ( #31297, #9628, #11986, #21674 ),
 .UNSPECIFIED., .F., .T. ) 
 B_SPLINE_CURVE_WITH_KNOTS ( ( 4, 4 ),
 ( 1.070062165543571808, 1.185496055862915066 ),
 .UNSPECIFIED. ) 
 CURVE ( )  GEOMETRIC_REPRESENTATION_ITEM ( )  RATIONAL_B_SPLINE_CURVE ( ( 1.000000000000000000, 0.9988898929684264516, 0.9988898929684264516, 1.000000000000000000 ) ) 
 REPRESENTATION_ITEM ( '' )  );
#5531=CARTESIAN_POINT ( 'NONE',  ( -59.38452994616203995, 3.117691453623969711, 1.799999999999819522 ) ) ;
#5538=CARTESIAN_POINT ( 'NONE',  ( -59.18700104863290079, 2.529210612537639680, -0.9442207491878787939 ) ) ;
#5549=CARTESIAN_POINT ( 'NONE',  ( -58.25952994616203284, -3.117691453623963938, -1.800000000000218092 ) ) ;
#5550=FACE_OUTER_BOUND ( 'NONE', #22031, .T. ) ;
#5559=ORIENTED_EDGE ( 'NONE', *, *, #13622, .F. ) ;
#5560=EDGE_CURVE ( 'NONE', #950, #29758, #21243, .T. ) ;
#5562=CARTESIAN_POINT ( 'NONE',  ( -60.00952994616204705, -4.643455692769866465E-15, 3.599999999999786038 ) ) ;
#5573=LINE ( 'NONE', #3801, #28114 ) ;
#5575=LINE ( 'NONE', #15069, #23580 ) ;
#5582=DIRECTION ( 'NONE',  ( 0.000000000000000000, -1.000000000000000000, -3.491481338843131383E-15 ) ) ;
#5587=ORIENTED_EDGE ( 'NONE', *, *, #19396, .F. ) ;
#5588=EDGE_CURVE ( 'NONE', #23827, #12035, #13598, .T. ) ;
#5596=CIRCLE ( 'NONE', #19265, 0.1000000000000000472 ) ;
#5598=CARTESIAN_POINT ( 'NONE',  ( -55.45655989232413674, 1.962990915244722245, 3.399999999999810285 ) ) ;
#5603=ORIENTED_EDGE ( 'NONE', *, *, #3930, .T. ) ;
#5622=CARTESIAN_POINT ( 'NONE',  ( -59.17457605456178271, 2.372231461058813107, 1.252354863327886259 ) ) ;
#5626=ORIENTED_EDGE ( 'NONE', *, *, #794, .T. ) ;
#5636=CARTESIAN_POINT ( 'NONE',  ( -59.76905989232412253, -2.944486372867088697, 1.699999999999776579 ) ) ;
#5639=CARTESIAN_POINT ( 'NONE',  ( -59.19999999999997442, -2.449420067797476452, 1.250136525132531817 ) ) ;
#5642=DIRECTION ( 'NONE',  ( 3.491481338843133355E-15, 3.491481338843133355E-15, -1.000000000000000000 ) ) ;
#5659=DIRECTION ( 'NONE',  ( -1.000000000000000000, 1.219044193948983948E-29, -3.491481338843133355E-15 ) ) ;
#5664=CARTESIAN_POINT ( 'NONE',  ( -58.08155989232410832, -1.962990915244700707, -3.400000000000216627 ) ) ;
#5665=ORIENTED_EDGE ( 'NONE', *, *, #16880, .F. ) ;
#5679=EDGE_CURVE ( 'NONE', #13873, #14560, #21649, .T. ) ;
#5680=DIRECTION ( 'NONE',  ( 0.000000000000000000, -1.000000000000000000, -3.491481338843132961E-15 ) ) ;
#5682=CARTESIAN_POINT ( 'NONE',  ( -58.57202994616204705, 2.078460969082640997, 3.599999999999802025 ) ) ;
#5694=DIRECTION ( 'NONE',  ( 1.000000000000000000, -1.219044193948983948E-29, 3.491481338843133355E-15 ) ) ;
#5698=CARTESIAN_POINT ( 'NONE',  ( -58.69702994616204705, 4.156921938165313080, -1.932741547809596393E-13 ) ) ;
#5712=CARTESIAN_POINT ( 'NONE',  ( -59.69591307118649581, -2.246549767191792668, 1.536452070276721926 ) ) ;
#5714=CARTESIAN_POINT ( 'NONE',  ( -56.81249999999995737, -1.962990915244703150, -3.400000000000210409 ) ) ;
#5721=DIRECTION ( 'NONE',  ( 0.000000000000000000, 1.000000000000000000, 0.000000000000000000 ) ) ;
#5733=( BOUNDED_CURVE ( )  B_SPLINE_CURVE ( 2, ( #23565, #21212, #13870, #6620, #26250, #18506, #11206, #6470, #16127 ),
 .UNSPECIFIED., .F., .T. ) 
 B_SPLINE_CURVE_WITH_KNOTS ( ( 3, 2, 2, 2, 3 ),
 ( 0.1944444444444444475, 0.2037037037037036924, 0.2222222222222222099, 0.2407407407407407274, 0.2500000000000000000 ),
 .UNSPECIFIED. ) 
 CURVE ( )  GEOMETRIC_REPRESENTATION_ITEM ( )  RATIONAL_B_SPLINE_CURVE ( ( 0.9330127018922192983, 0.9330127018922194093, 1.000000000000000000, 0.8660254037844387076, 1.000000000000000000, 0.8660254037844387076, 1.000000000000000000, 0.9330127018922191873, 0.9330127018922192983 ) ) 
 REPRESENTATION_ITEM ( '' )  );
#5736=EDGE_LOOP ( 'NONE', ( #1295, #10656, #15055, #28592 ) ) ;
#5743=CARTESIAN_POINT ( 'NONE',  ( -59.63452994616203284, 2.093608279459373297E-14, -3.600000000000211475 ) ) ;
#5747=AXIS2_PLACEMENT_3D ( 'NONE', #12234, #24419, #10166 ) ;
#5751=CARTESIAN_POINT ( 'NONE',  ( -55.18749999999996447, 1.962990915244749557, -3.400000000000187317 ) ) ;
#5762=CARTESIAN_POINT ( 'NONE',  ( -54.39999999999996305, -1.499999999999978684, -4.029888335922192866 ) ) ;
#5773=CARTESIAN_POINT ( 'NONE',  ( -55.81249999999997158, 3.925981830489463142, -1.840516183884902743E-13 ) ) ;
#5783=DIRECTION ( 'NONE',  ( 0.000000000000000000, -1.000000000000000000, -3.491481338843137694E-15 ) ) ;
#5784=ADVANCED_FACE ( 'NONE', ( #2353 ), #13507, .T. ) ;
#5790=CARTESIAN_POINT ( 'NONE',  ( -58.26905989232412253, -2.944486372867088697, 1.699999999999781686 ) ) ;
#5793=DIRECTION ( 'NONE',  ( 0.000000000000000000, -1.000000000000000000, -2.603302919143007729E-15 ) ) ;
#5795=CARTESIAN_POINT ( 'NONE',  ( -59.47025482456093926, 3.201828568350844062, 1.352206208478290872 ) ) ;
#5799=FACE_OUTER_BOUND ( 'NONE', #6066, .T. ) ;
#5814=DIRECTION ( 'NONE',  ( 1.000000000000000000, -1.219044193948983948E-29, 3.491481338843133355E-15 ) ) ;
#5816=CARTESIAN_POINT ( 'NONE',  ( -57.70655989232413674, 1.962990915244717582, 3.399999999999804512 ) ) ;
#5819=CARTESIAN_POINT ( 'NONE',  ( -58.14405989232411542, -2.944486372867072266, -1.700000000000223777 ) ) ;
#5831=CARTESIAN_POINT ( 'NONE',  ( -55.57202994616207548, 2.078460969082646770, 3.599999999999810019 ) ) ;
#5840=CARTESIAN_POINT ( 'NONE',  ( -56.94702994616206126, -2.078460969082670751, 3.599999999999782041 ) ) ;
#5842=DIRECTION ( 'NONE',  ( 0.000000000000000000, 1.000000000000000000, 4.336808689942015369E-15 ) ) ;
#5845=ORIENTED_EDGE ( 'NONE', *, *, #4985, .F. ) ;
#5848=DIRECTION ( 'NONE',  ( -1.000000000000000000, 1.219044193948983948E-29, -3.491481338843133355E-15 ) ) ;
#5857=CARTESIAN_POINT ( 'NONE',  ( -59.75952994616203284, -3.117691453623963938, -1.800000000000223199 ) ) ;
#5867=TOROIDAL_SURFACE ( 'NONE', #2317, 0.2000000000000000111, 0.1000000000000000056 ) ;
#5886=VERTEX_POINT ( 'NONE', #8341 ) ;
#5890=DIRECTION ( 'NONE',  ( 1.000000000000000000, -1.219044193948983948E-29, 3.491481338843133355E-15 ) ) ;
#5900=CARTESIAN_POINT ( 'NONE',  ( -58.20655989232411542, -3.399999999999991029, -2.246812820714294660E-13 ) ) ;
#5906=VECTOR ( 'NONE', #4448, 1000.000000000000000 ) ;
#5908=EDGE_CURVE ( 'NONE', #4682, #30038, #922, .T. ) ;
#5909=CARTESIAN_POINT ( 'NONE',  ( -60.32202994616201863, 2.078460969082674747, -3.600000000000205258 ) ) ;
#5912=DIRECTION ( 'NONE',  ( 0.000000000000000000, 1.000000000000000000, 4.336808689942015369E-15 ) ) ;
#5916=CARTESIAN_POINT ( 'NONE',  ( -56.99999999999997158, -2.944486372867089141, 1.699999999999786571 ) ) ;
#5918=AXIS2_PLACEMENT_3D ( 'NONE', #20657, #11270, #25694 ) ;
#5929=CARTESIAN_POINT ( 'NONE',  ( -59.69740665358683884, 2.094969456803113861, 1.745644717383348477 ) ) ;
#5944=CARTESIAN_POINT ( 'NONE',  ( -58.49999999999997868, -2.944486372867089141, 1.699999999999781242 ) ) ;
#5950=B_SPLINE_CURVE_WITH_KNOTS ( 'NONE', 3,
 ( #3446, #12764, #25118, #29872 ),
 .UNSPECIFIED., .F., .F.,
 ( 4, 4 ),
 ( 0.000000000000000000, 3.288265101740459116E-05 ),
 .UNSPECIFIED. ) ;
#5952=EDGE_CURVE ( 'NONE', #10254, #13776, #11040, .T. ) ;
#5963=CARTESIAN_POINT ( 'NONE',  ( -59.08155989232413674, -1.962990915244731571, 3.399999999999781419 ) ) ;
#5980=ORIENTED_EDGE ( 'NONE', *, *, #15195, .F. ) ;
#5981=CARTESIAN_POINT ( 'NONE',  ( -59.37009172985672478, 3.234433134214944605, -1.048065980887175730 ) ) ;
#5991=DIRECTION ( 'NONE',  ( -1.000000000000000000, 1.219044193948983948E-29, -3.491481338843133355E-15 ) ) ;
#5996=ORIENTED_EDGE ( 'NONE', *, *, #18752, .F. ) ;
#6001=DIRECTION ( 'NONE',  ( 0.000000000000000000, -1.000000000000000000, -3.491481338843132961E-15 ) ) ;
#6009=CARTESIAN_POINT ( 'NONE',  ( -58.38452994616204705, -3.117691453623983033, 1.799999999999769784 ) ) ;
#6019=CARTESIAN_POINT ( 'NONE',  ( -59.15159661603878050, 2.488695505467597879, -0.9494100618347165454 ) ) ;
#6022=VERTEX_POINT ( 'NONE', #18647 ) ;
#6024=CARTESIAN_POINT ( 'NONE',  ( -58.99005354137801049, -3.399999999999994138, 0.9110272542655820649 ) ) ;
#6029=CARTESIAN_POINT ( 'NONE',  ( -60.69702994616205416, -2.078460969082657872, 3.599999999999776712 ) ) ;
#6036=VERTEX_POINT ( 'NONE', #23541 ) ;
#6037=CARTESIAN_POINT ( 'NONE',  ( -61.00952994616203284, 3.117691453623994580, -1.800000000000202993 ) ) ;
#6048=CARTESIAN_POINT ( 'NONE',  ( -59.37499999999997868, -2.099645193746120606E-14, 3.399999999999788525 ) ) ;
#6053=DIRECTION ( 'NONE',  ( 0.000000000000000000, -1.000000000000000000, -3.491481338843137694E-15 ) ) ;
#6065=CARTESIAN_POINT ( 'NONE',  ( -59.19999999999997442, 8.366749974758448157E-15, -2.103076948839454410E-13 ) ) ;
#6066=EDGE_LOOP ( 'NONE', ( #10024, #28475, #28377, #9109 ) ) ;
#6067=CARTESIAN_POINT ( 'NONE',  ( -55.82202994616203995, 2.078460969082679188, -3.600000000000186606 ) ) ;
#6069=ADVANCED_FACE ( 'NONE', ( #16262 ), #25590, .T. ) ;
#6070=CARTESIAN_POINT ( 'NONE',  ( -56.26905989232412963, 2.944486372867092250, 1.699999999999811218 ) ) ;
#6075=CARTESIAN_POINT ( 'NONE',  ( -56.49999999999997868, 2.944486372867092250, 1.699999999999810774 ) ) ;
#6079=CARTESIAN_POINT ( 'NONE',  ( -59.59999999999998721, -2.157671697750204842, 1.538490443495526216 ) ) ;
#6087=EDGE_LOOP ( 'NONE', ( #29477, #28123, #19386, #9693, #9286, #3281, #14063 ) ) ;
#6096=CARTESIAN_POINT ( 'NONE',  ( -57.43749999999996447, 1.962990915244749557, -3.400000000000195310 ) ) ;
#6097=CARTESIAN_POINT ( 'NONE',  ( -59.39297944956340558, 2.353586303871975982, 1.218361332808637121 ) ) ;
#6104=ORIENTED_EDGE ( 'NONE', *, *, #29326, .F. ) ;
#6111=CARTESIAN_POINT ( 'NONE',  ( -59.14405989232412963, -3.920666489018302546E-15, 3.399999999999788969 ) ) ;
#6116=DIRECTION ( 'NONE',  ( 1.000000000000000000, -1.219044193948983948E-29, 3.491481338843133355E-15 ) ) ;
#6125=EDGE_CURVE ( 'NONE', #17201, #5886, #9294, .T. ) ;
#6141=CARTESIAN_POINT ( 'NONE',  ( -55.99005354137803181, -3.399999999999995026, 0.9110272542656013828 ) ) ;
#6148=EDGE_CURVE ( 'NONE', #27932, #21024, #397, .T. ) ;
#6165=VERTEX_POINT ( 'NONE', #31130 ) ;
#6166=DIRECTION ( 'NONE',  ( 0.000000000000000000, 0.4295302013422852561, -0.9030524935654935526 ) ) ;
#6170=ORIENTED_EDGE ( 'NONE', *, *, #15374, .F. ) ;
#6175=CARTESIAN_POINT ( 'NONE',  ( -60.19702994616203995, 4.156921938165313080, -1.985113767892243204E-13 ) ) ;
#6184=CARTESIAN_POINT ( 'NONE',  ( -60.19702994616203995, 4.156921938165313080, -1.985113767892243204E-13 ) ) ;
#6197=AXIS2_PLACEMENT_3D ( 'NONE', #27143, #23998, #29361 ) ;
#6199=CARTESIAN_POINT ( 'NONE',  ( -59.69142724121850563, -2.412383461849193278, -1.233589124872107146 ) ) ;
#6210=FILL_AREA_STYLE ('',( #4291 ) ) ;
#6211=CARTESIAN_POINT ( 'NONE',  ( -55.95655989232412963, -3.925981830489445379, -2.129311736262419800E-13 ) ) ;
#6214=VERTEX_POINT ( 'NONE', #12427 ) ;
#6218=CARTESIAN_POINT ( 'NONE',  ( -56.62499999999996447, 2.944486372867106905, -1.700000000000188471 ) ) ;
#6224=CARTESIAN_POINT ( 'NONE',  ( -54.39999999999997726, -3.624999999999988010, -2.339607799264337154E-13 ) ) ;
#6227=CYLINDRICAL_SURFACE ( 'NONE', #842, 3.624999999999996447 ) ;
#6234=VERTEX_POINT ( 'NONE', #17059 ) ;
#6236=CARTESIAN_POINT ( 'NONE',  ( -59.09999999999997300, 8.366749974758448157E-15, -2.099585467500611340E-13 ) ) ;
#6242=CARTESIAN_POINT ( 'NONE',  ( -57.74999999999997158, -2.944486372867089141, 1.699999999999783906 ) ) ;
#6245=CIRCLE ( 'NONE', #3213, 0.1000000000000000472 ) ;
#6250=EDGE_LOOP ( 'NONE', ( #15388, #10119, #22275 ) ) ;
#6261=CARTESIAN_POINT ( 'NONE',  ( -59.19999999999997442, -2.444956024269904660, 1.250136525132532261 ) ) ;
#6262=DIRECTION ( 'NONE',  ( 0.000000000000000000, -1.000000000000000000, -3.491481338843133355E-15 ) ) ;
#6284=CARTESIAN_POINT ( 'NONE',  ( -54.39999999999999147, -1.400000000000006795, 3.959797974644449603 ) ) ;
#6286=ORIENTED_EDGE ( 'NONE', *, *, #11078, .F. ) ;
#6293=CARTESIAN_POINT ( 'NONE',  ( -56.57202994616203995, 2.078460969082674747, -3.600000000000191935 ) ) ;
#6299=ADVANCED_FACE ( 'NONE', ( #27624 ), #27160, .T. ) ;
#6303=CARTESIAN_POINT ( 'NONE',  ( -59.69999999999997442, -3.399999999999991473, -2.235080921937235780E-13 ) ) ;
#6307=VERTEX_POINT ( 'NONE', #3571 ) ;
#6323=CARTESIAN_POINT ( 'NONE',  ( -59.35358983848620795, 2.308634493194285486, 1.301040651491357503 ) ) ;
#6329=FACE_OUTER_BOUND ( 'NONE', #9620, .T. ) ;
#6332=CARTESIAN_POINT ( 'NONE',  ( -59.69999999999998153, 2.121207708687718352, 1.750136525132546472 ) ) ;
#6336=CARTESIAN_POINT ( 'NONE',  ( -54.49999999999996447, -1.557046979865753578, -3.273565289175143445 ) ) ;
#6342=ORIENTED_EDGE ( 'NONE', *, *, #3470, .F. ) ;
#6352=CIRCLE ( 'NONE', #29093, 0.2000000000000000944 ) ;
#6361=CARTESIAN_POINT ( 'NONE',  ( -56.95655989232412963, 1.962990915244722245, 3.399999999999804956 ) ) ;
#6369=CARTESIAN_POINT ( 'NONE',  ( -57.93749999999998579, 1.962990915244722689, 3.399999999999801847 ) ) ;
#6383=CARTESIAN_POINT ( 'NONE',  ( -59.68033635780795976, -2.213242577962092117, 1.527458850614529018 ) ) ;
#6395=CARTESIAN_POINT ( 'NONE',  ( -54.49999999999997868, -3.524999999999988365, -2.339607799264337154E-13 ) ) ;
#6397=CARTESIAN_POINT ( 'NONE',  ( -57.49999999999995737, 2.023778652682507790E-14, -3.400000000000204636 ) ) ;
#6403=ORIENTED_EDGE ( 'NONE', *, *, #7742, .T. ) ;
#6411=DIRECTION ( 'NONE',  ( -1.000000000000000000, 1.219044193948984088E-29, -3.491481338843133750E-15 ) ) ;
#6412=CARTESIAN_POINT ( 'NONE',  ( -44.59999999999996589, 1.500000000000021538, -3.363870538531645416 ) ) ;
#6423=CARTESIAN_POINT ( 'NONE',  ( -54.39999999999997726, -6.102218906431378987E-14, -2.213041600731275921E-13 ) ) ;
#6424=AXIS2_PLACEMENT_3D ( 'NONE', #23148, #10777, #5721 ) ;
#6440=ORIENTED_EDGE ( 'NONE', *, *, #18781, .T. ) ;
#6459=EDGE_CURVE ( 'NONE', #12851, #18483, #25872, .T. ) ;
#6464=CARTESIAN_POINT ( 'NONE',  ( -56.88452994616205416, -3.117691453623976816, 1.799999999999785993 ) ) ;
#6470=CARTESIAN_POINT ( 'NONE',  ( -55.92306624327023457, -3.399999999999986589, -0.9110272542660333706 ) ) ;
#6476=CARTESIAN_POINT ( 'NONE',  ( -56.97099364905386665, -3.399999999999994138, 0.9110272542655981631 ) ) ;
#6485=EDGE_LOOP ( 'NONE', ( #17135, #21062, #12411 ) ) ;
#6497=CARTESIAN_POINT ( 'NONE',  ( -59.39321376305881728, 3.357136383570068272, 1.250136525132546916 ) ) ;
#6506=CARTESIAN_POINT ( 'NONE',  ( -59.64494627086173040, 2.036191742483342448, 1.711547443303939264 ) ) ;
#6521=CARTESIAN_POINT ( 'NONE',  ( -54.49999999999996447, -1.399999999999979039, -3.959797974644881258 ) ) ;
#6523=CARTESIAN_POINT ( 'NONE',  ( -59.69999999999996732, -1.873569517744609447, -3.074042495181142698 ) ) ;
#6525=CARTESIAN_POINT ( 'NONE',  ( -54.46614378277664059, -2.255560380866761250, -2.805788190199900889 ) ) ;
#6527=CARTESIAN_POINT ( 'NONE',  ( -56.83155989232414385, -1.962990915244731571, 3.399999999999789413 ) ) ;
#6533=CARTESIAN_POINT ( 'NONE',  ( -54.94702994616205416, 4.156921938165313080, -1.801810997602979365E-13 ) ) ;
#6534=CARTESIAN_POINT ( 'NONE',  ( -54.89405989232412963, 2.944486372867106461, -1.700000000000182254 ) ) ;
#6538=LINE ( 'NONE', #27761, #30206 ) ;
#6558=CARTESIAN_POINT ( 'NONE',  ( -54.94702994616205416, 4.156921938165313080, -1.801810997602979365E-13 ) ) ;
#6562=ORIENTED_EDGE ( 'NONE', *, *, #3891, .F. ) ;
#6574=CARTESIAN_POINT ( 'NONE',  ( -55.68749999999999289, 1.962990915244720691, 3.399999999999810285 ) ) ;
#6577=EDGE_CURVE ( 'NONE', #22982, #14560, #14773, .T. ) ;
#6592=ORIENTED_EDGE ( 'NONE', *, *, #23511, .T. ) ;
#6602=ORIENTED_EDGE ( 'NONE', *, *, #17242, .T. ) ;
#6613=CARTESIAN_POINT ( 'NONE',  ( -59.63452994616203284, 2.093608279459373297E-14, -3.600000000000211475 ) ) ;
#6620=CARTESIAN_POINT ( 'NONE',  ( -55.70655989232411542, 1.962990915244752888, -3.400000000000186873 ) ) ;
#6624=CARTESIAN_POINT ( 'NONE',  ( -59.63452994616203284, 2.710830266229639327E-14, -3.600000000000211475 ) ) ;
#6634=ORIENTED_EDGE ( 'NONE', *, *, #13644, .T. ) ;
#6638=DIRECTION ( 'NONE',  ( -1.000000000000000000, 0.000000000000000000, -3.491481338843153471E-15 ) ) ;
#6642=COLOUR_RGB ( '', 0.31764706, 0.68627451, 0.89019608) ;
#6645=FACE_OUTER_BOUND ( 'NONE', #28908, .T. ) ;
#6659=CARTESIAN_POINT ( 'NONE',  ( -59.63444153017528748, 2.031330036680259354, 1.710319191226306712 ) ) ;
#6670=CARTESIAN_POINT ( 'NONE',  ( -54.39999999999999147, 1.399999999999996136, 3.959797974644420737 ) ) ;
#6676=CARTESIAN_POINT ( 'NONE',  ( -56.89405989232413674, -3.920666489018330156E-15, 3.399999999999796962 ) ) ;
#6677=ORIENTED_EDGE ( 'NONE', *, *, #6790, .F. ) ;
#6683=CARTESIAN_POINT ( 'NONE',  ( -54.63452994616206126, -3.117691453623976816, 1.799999999999793765 ) ) ;
#6692=CIRCLE ( 'NONE', #6197, 0.2000000000000000944 ) ;
#6700=ORIENTED_EDGE ( 'NONE', *, *, #9300, .T. ) ;
#6706=CARTESIAN_POINT ( 'NONE',  ( -60.37499999999995737, 2.944486372867106905, -1.700000000000201794 ) ) ;
#6714=ORIENTED_EDGE ( 'NONE', *, *, #24173, .F. ) ;
#6719=ORIENTED_EDGE ( 'NONE', *, *, #21241, .F. ) ;
#6721=EDGE_CURVE ( 'NONE', #16489, #10532, #3493, .T. ) ;
#6736=DIRECTION ( 'NONE',  ( -3.491481338843133355E-15, -1.216509871872716567E-14, 1.000000000000000000 ) ) ;
#6752=( BOUNDED_SURFACE ( )  B_SPLINE_SURFACE ( 3, 2, ( 
 ( #4415, #4098, #26102 ),
 ( #23582, #1558, #9176 ),
 ( #16446, #23423, #18362 ),
 ( #1705, #9008, #14064 ) ),
 .UNSPECIFIED., .F., .F., .F. ) 
 B_SPLINE_SURFACE_WITH_KNOTS ( ( 4, 4 ),
 ( 3, 3 ),
 ( 1.069308579029437212, 1.196413504413466500 ),
 ( 0.000000000000000000, 1.000000000000000000 ),
 .UNSPECIFIED. ) 
 GEOMETRIC_REPRESENTATION_ITEM ( )  RATIONAL_B_SPLINE_SURFACE ( (
 ( 1.000000000000000000, 0.8415238966082415617, 1.000000000000000000),
 ( 1.000000000000000000, 0.8319656872388342395, 1.000000000000000000),
 ( 1.000000000000000000, 0.8219112105083486997, 1.000000000000000000),
 ( 1.000000000000000000, 0.8113889037030929119, 1.000000000000000000) ) ) 
 REPRESENTATION_ITEM ( '' )  SURFACE ( )  );
#6763=CARTESIAN_POINT ( 'NONE',  ( -58.63452994616204705, 3.117691453623979481, 1.799999999999803757 ) ) ;
#6764=CARTESIAN_POINT ( 'NONE',  ( -59.10063086805173072, -2.465840246036694161, -0.9706348448640983451 ) ) ;
#6769=DIRECTION ( 'NONE',  ( -1.499696682456171775E-15, 0.9030524935654854479, 0.4295302013423024645 ) ) ;
#6790=EDGE_CURVE ( 'NONE', #23830, #24402, #5520, .T. ) ;
#6812=EDGE_LOOP ( 'NONE', ( #21115, #13090, #6719, #27620 ) ) ;
#6818=AXIS2_PLACEMENT_3D ( 'NONE', #19737, #6913, #26223 ) ;
#6832=DIRECTION ( 'NONE',  ( 1.000000000000000000, -1.219044193948983948E-29, 3.491481338843133355E-15 ) ) ;
#6840=CARTESIAN_POINT ( 'NONE',  ( -60.81249999999997868, -1.962990915244731793, 3.399999999999776090 ) ) ;
#6864=ORIENTED_EDGE ( 'NONE', *, *, #7588, .T. ) ;
#6867=CARTESIAN_POINT ( 'NONE',  ( -58.93749999999995737, 1.962990915244749557, -3.400000000000200640 ) ) ;
#6871=DIRECTION ( 'NONE',  ( 0.000000000000000000, 1.000000000000000000, 3.491481338843132961E-15 ) ) ;
#6875=CARTESIAN_POINT ( 'NONE',  ( -57.63452994616205416, -3.117691453623976816, 1.799999999999783329 ) ) ;
#6893=CIRCLE ( 'NONE', #14481, 3.399999999999999911 ) ;
#6898=AXIS2_PLACEMENT_3D ( 'NONE', #26729, #9482, #14206 ) ;
#6904=AXIS2_PLACEMENT_3D ( 'NONE', #29826, #17810, #1159 ) ;
#6913=DIRECTION ( 'NONE',  ( -1.000000000000000000, 1.219044193948983948E-29, -3.491481338843133355E-15 ) ) ;
#6921=CARTESIAN_POINT ( 'NONE',  ( -59.69999999999998153, -3.161828374300064581, 1.538811659727342462 ) ) ;
#6924=LINE ( 'NONE', #23393, #28711 ) ;
#6930=CARTESIAN_POINT ( 'NONE',  ( -59.40875807382336404, 3.366278345796976268, 1.250136525132555798 ) ) ;
#6933=CARTESIAN_POINT ( 'NONE',  ( -58.07202994616203995, 2.078460969082674747, -3.600000000000197709 ) ) ;
#6934=CIRCLE ( 'NONE', #15005, 0.09999999999999986677 ) ;
#6938=CARTESIAN_POINT ( 'NONE',  ( -58.47099364905386665, -3.399999999999994138, 0.9110272542655848405 ) ) ;
#6941=EDGE_CURVE ( 'NONE', #19844, #17127, #15403, .T. ) ;
#6954=CARTESIAN_POINT ( 'NONE',  ( -57.34599364905385954, 3.400000000000012346, -0.9110272542660015072 ) ) ;
#6956=EDGE_CURVE ( 'NONE', #24434, #23157, #23796, .T. ) ;
#6959=FACE_OUTER_BOUND ( 'NONE', #2357, .T. ) ;
#6971=CARTESIAN_POINT ( 'NONE',  ( -59.69999999999997442, 8.366749974758454467E-15, -2.120534355533670266E-13 ) ) ;
#6981=CARTESIAN_POINT ( 'NONE',  ( -59.43788607448336592, 2.385332005665378841, -1.158943404468661731 ) ) ;
#6984=CARTESIAN_POINT ( 'NONE',  ( -59.19999999999997442, 4.156921938165309527, 1.250136525132554910 ) ) ;
#6990=CARTESIAN_POINT ( 'NONE',  ( -59.40743313238012036, 2.395752775956333291, 1.250136525132548027 ) ) ;
#6991=CARTESIAN_POINT ( 'NONE',  ( -59.62365256889266618, 2.027865038274679232, 1.710353782976151482 ) ) ;
#6992=VERTEX_POINT ( 'NONE', #22278 ) ;
#6996=CARTESIAN_POINT ( 'NONE',  ( -44.59999999999996589, 1.400000000000023670, -3.959797974644836405 ) ) ;
#7009=ORIENTED_EDGE ( 'NONE', *, *, #19784, .T. ) ;
#7012=ORIENTED_EDGE ( 'NONE', *, *, #677, .T. ) ;
#7014=CARTESIAN_POINT ( 'NONE',  ( -54.75952994616206837, -4.643455692769931152E-15, 3.599999999999804245 ) ) ;
#7024=DIRECTION ( 'NONE',  ( 0.000000000000000000, -0.3333333333333469706, -0.9428090415820586934 ) ) ;
#7040=CARTESIAN_POINT ( 'NONE',  ( -55.32202994616205416, -4.156921938165296204, -2.115361882398036228E-13 ) ) ;
#7048=CARTESIAN_POINT ( 'NONE',  ( -55.50952994616206126, -4.643455692769921685E-15, 3.599999999999801581 ) ) ;
#7058=AXIS2_PLACEMENT_3D ( 'NONE', #28664, #7133, #572 ) ;
#7059=CARTESIAN_POINT ( 'NONE',  ( -59.69999999999997442, -2.455304892039217091, -1.238538609462283446 ) ) ;
#7070=CARTESIAN_POINT ( 'NONE',  ( -59.14778739134288799, -2.353873335156955182, 1.243527661805360340 ) ) ;
#7085=EDGE_CURVE ( 'NONE', #24984, #4847, #5596, .T. ) ;
#7089=CIRCLE ( 'NONE', #14648, 0.1000000000000028644 ) ;
#7090=DIRECTION ( 'NONE',  ( 0.000000000000000000, 1.000000000000000000, 3.491481338843132961E-15 ) ) ;
#7091=CARTESIAN_POINT ( 'NONE',  ( -60.69702994616205416, -2.078460969082657872, 3.599999999999776712 ) ) ;
#7094=EDGE_CURVE ( 'NONE', #23157, #11667, #23274, .T. ) ;
#7101=ORIENTED_EDGE ( 'NONE', *, *, #3891, .T. ) ;
#7108=ORIENTED_EDGE ( 'NONE', *, *, #29412, .T. ) ;
#7114=DIRECTION ( 'NONE',  ( -1.000000000000000000, 1.219044193948983948E-29, -3.491481338843133355E-15 ) ) ;
#7133=DIRECTION ( 'NONE',  ( -1.000000000000000000, 1.219044193948983948E-29, -3.491481338843133355E-15 ) ) ;
#7135=ADVANCED_FACE ( 'NONE', ( #8475 ), #13210, .T. ) ;
#7138=CARTESIAN_POINT ( 'NONE',  ( -44.59999999999995879, -1.399999999999978817, -4.029888335922158227 ) ) ;
#7139=DIRECTION ( 'NONE',  ( 3.491481338843133355E-15, 3.491481338843133355E-15, -1.000000000000000000 ) ) ;
#7142=CARTESIAN_POINT ( 'NONE',  ( -59.59999999999998721, 2.022492213459062160, 1.712315755489264513 ) ) ;
#7145=DIRECTION ( 'NONE',  ( -3.491481338843133355E-15, -3.491481338843133355E-15, 1.000000000000000000 ) ) ;
#7162=CARTESIAN_POINT ( 'NONE',  ( -60.08155989232412253, 3.925981830489463142, -1.989569613369437003E-13 ) ) ;
#7168=CARTESIAN_POINT ( 'NONE',  ( -54.88452994616206126, 3.117691453623979481, 1.799999999999816858 ) ) ;
#7171=DIRECTION ( 'NONE',  ( 0.000000000000000000, -1.000000000000000000, -4.336808689942015369E-15 ) ) ;
#7174=LINE ( 'NONE', #46, #7434 ) ;
#7185=VERTEX_POINT ( 'NONE', #18450 ) ;
#7187=CARTESIAN_POINT ( 'NONE',  ( -54.38452994616203995, 2.093608279459366986E-14, -3.600000000000193268 ) ) ;
#7194=ADVANCED_FACE ( 'NONE', ( #13674 ), #3873, .F. ) ;
#7197=CARTESIAN_POINT ( 'NONE',  ( -56.63452994616203284, 2.093608279459369510E-14, -3.600000000000201261 ) ) ;
#7198=ORIENTED_EDGE ( 'NONE', *, *, #11207, .F. ) ;
#7203=DIRECTION ( 'NONE',  ( 0.000000000000000000, -1.000000000000000000, -4.336808689942015369E-15 ) ) ;
#7212=CARTESIAN_POINT ( 'NONE',  ( -44.49999999999997868, 1.400000000000009681, -1.540948453285710255E-13 ) ) ;
#7227=VERTEX_POINT ( 'NONE', #4030 ) ;
#7228=EDGE_CURVE ( 'NONE', #950, #9817, #9636, .T. ) ;
#7237=CARTESIAN_POINT ( 'NONE',  ( -54.33155989232412253, -1.962990915244706924, -3.400000000000199751 ) ) ;
#7241=DIRECTION ( 'NONE',  ( 0.000000000000000000, 1.000000000000000000, 3.491481338843135722E-15 ) ) ;
#7248=CARTESIAN_POINT ( 'NONE',  ( -59.66183546925923764, -3.174920041538525251, -1.216504307364950854 ) ) ;
#7251=CARTESIAN_POINT ( 'NONE',  ( -57.65400635094607651, -3.399999999999988365, -0.9110272542660372563 ) ) ;
#7255=EDGE_CURVE ( 'NONE', #16970, #21074, #9132, .T. ) ;
#7265=CIRCLE ( 'NONE', #29484, 3.524999999999996358 ) ;
#7268=CARTESIAN_POINT ( 'NONE',  ( -57.99999999999997868, 2.944486372867089141, 1.699999999999810774 ) ) ;
#7282=DIRECTION ( 'NONE',  ( 3.491481338843133355E-15, 3.491481338843133355E-15, -1.000000000000000000 ) ) ;
#7287=UNCERTAINTY_MEASURE_WITH_UNIT (LENGTH_MEASURE( 1.000000000000000082E-05 ), #16339, 'distance_accuracy_value', 'NONE');
#7290=CARTESIAN_POINT ( 'NONE',  ( -44.49999999999996447, 1.514093959731561467, -3.183260039818548215 ) ) ;
#7303=CARTESIAN_POINT ( 'NONE',  ( -59.60130753818947369, -2.158066088952245387, 1.537948259120531125 ) ) ;
#7304=ORIENTED_EDGE ( 'NONE', *, *, #4570, .T. ) ;
#7310=VECTOR ( 'NONE', #5694, 1000.000000000000000 ) ;
#7312=CARTESIAN_POINT ( 'NONE',  ( -56.82202994616205416, -4.156921938165296204, -2.167734102480683039E-13 ) ) ;
#7319=VECTOR ( 'NONE', #10994, 1000.000000000000000 ) ;
#7335=ORIENTED_EDGE ( 'NONE', *, *, #15635, .T. ) ;
#7336=AXIS2_PLACEMENT_3D ( 'NONE', #30565, #23310, #18103 ) ;
#7338=CARTESIAN_POINT ( 'NONE',  ( -58.13452994616202574, 2.093608279459371404E-14, -3.600000000000206146 ) ) ;
#7344=CARTESIAN_POINT ( 'NONE',  ( -56.75952994616203995, -3.117691453623963938, -1.800000000000212763 ) ) ;
#7345=VERTEX_POINT ( 'NONE', #24142 ) ;
#7347=CARTESIAN_POINT ( 'NONE',  ( -44.49999999999997868, -1.399999999999992806, -1.638709930773317737E-13 ) ) ;
#7348=AXIS2_PLACEMENT_3D ( 'NONE', #21289, #21129, #16836 ) ;
#7351=DIRECTION ( 'NONE',  ( 0.000000000000000000, 1.000000000000000000, 4.336808689942015369E-15 ) ) ;
#7389=CARTESIAN_POINT ( 'NONE',  ( -61.13452994616202574, 2.093608279459375190E-14, -3.600000000000216804 ) ) ;
#7391=AXIS2_PLACEMENT_3D ( 'NONE', #2172, #14357, #24028 ) ;
#7392=AXIS2_PLACEMENT_3D ( 'NONE', #3178, #801, #10468 ) ;
#7398=LINE ( 'NONE', #9480, #27087 ) ;
#7400=AXIS2_PLACEMENT_3D ( 'NONE', #14753, #24414, #17293 ) ;
#7425=ORIENTED_EDGE ( 'NONE', *, *, #16880, .T. ) ;
#7434=VECTOR ( 'NONE', #24410, 1000.000000000000000 ) ;
#7442=CARTESIAN_POINT ( 'NONE',  ( -59.69999999999997442, 8.366749974758454467E-15, -2.120534355533670266E-13 ) ) ;
#7459=ORIENTED_EDGE ( 'NONE', *, *, #26901, .T. ) ;
#7470=CARTESIAN_POINT ( 'NONE',  ( -60.89405989232410121, 2.944486372867106461, -1.700000000000203348 ) ) ;
#7474=ORIENTED_EDGE ( 'NONE', *, *, #20115, .F. ) ;
#7476=CARTESIAN_POINT ( 'NONE',  ( -58.63452994616204705, 3.117691453623979481, 1.799999999999803757 ) ) ;
#7477=AXIS2_PLACEMENT_3D ( 'NONE', #14487, #9606, #18943 ) ;
#7481=ADVANCED_FACE ( 'NONE', ( #5270 ), #7623, .T. ) ;
#7489=CARTESIAN_POINT ( 'NONE',  ( -57.83155989232412253, 3.400000000000007905, -1.837192174579415629E-13 ) ) ;
#7491=DIRECTION ( 'NONE',  ( -3.491481338843133355E-15, -3.491481338843133355E-15, 1.000000000000000000 ) ) ;
#7501=EDGE_CURVE ( 'NONE', #20905, #9490, #30366, .T. ) ;
#7505=EDGE_LOOP ( 'NONE', ( #5249, #30293, #6634, #968 ) ) ;
#7510=CARTESIAN_POINT ( 'NONE',  ( -57.25952994616203995, 3.117691453623994580, -1.800000000000189671 ) ) ;
#7534=ORIENTED_EDGE ( 'NONE', *, *, #6125, .T. ) ;
#7536=ORIENTED_EDGE ( 'NONE', *, *, #18504, .T. ) ;
#7551=DIRECTION ( 'NONE',  ( 0.000000000000000000, 1.000000000000000000, 3.491481338843137694E-15 ) ) ;
#7555=CARTESIAN_POINT ( 'NONE',  ( -56.33155989232412253, 3.925981830489463142, -1.858639063162819723E-13 ) ) ;
#7571=FILL_AREA_STYLE ('',( #12300 ) ) ;
#7581=CARTESIAN_POINT ( 'NONE',  ( -57.89405989232411542, 2.944486372867110902, -1.700000000000184697 ) ) ;
#7588=EDGE_CURVE ( 'NONE', #17883, #30573, #17176, .T. ) ;
#7598=CARTESIAN_POINT ( 'NONE',  ( -59.43190135328987367, 3.335228286247303053, -1.083751783614652409 ) ) ;
#7599=CARTESIAN_POINT ( 'NONE',  ( -44.59999999999998010, 8.366749974758271452E-15, -1.593320673368357319E-13 ) ) ;
#7605=ORIENTED_EDGE ( 'NONE', *, *, #16812, .T. ) ;
#7613=DIRECTION ( 'NONE',  ( 0.000000000000000000, -1.000000000000000000, -3.491481338843133355E-15 ) ) ;
#7619=EDGE_LOOP ( 'NONE', ( #31215, #13313, #15842, #28334 ) ) ;
#7623=TOROIDAL_SURFACE ( 'NONE', #25809, 0.2000000000000000111, 0.1000000000000000056 ) ;
#7624=CARTESIAN_POINT ( 'NONE',  ( -57.82202994616206126, 2.078460969082646770, 3.599999999999802025 ) ) ;
#7629=CARTESIAN_POINT ( 'NONE',  ( -56.70655989232412253, -3.399999999999991029, -2.112596694108398482E-13 ) ) ;
#7630=ADVANCED_FACE ( 'NONE', ( #8839 ), #8629, .T. ) ;
#7637=VERTEX_POINT ( 'NONE', #28339 ) ;
#7653=CARTESIAN_POINT ( 'NONE',  ( -54.58155989232414385, -1.962990915244731571, 3.399999999999797851 ) ) ;
#7678=CARTESIAN_POINT ( 'NONE',  ( -59.18789508915042319, 2.395752775956333291, 1.250136525132548915 ) ) ;
#7687=EDGE_CURVE ( 'NONE', #7227, #11190, #9187, .T. ) ;
#7696=CARTESIAN_POINT ( 'NONE',  ( -54.89405989232412963, 2.944486372867106461, -1.700000000000182254 ) ) ;
#7700=DIRECTION ( 'NONE',  ( 1.000000000000000000, -1.219044193948983948E-29, 3.491481338843133355E-15 ) ) ;
#7704=ADVANCED_FACE ( 'NONE', ( #25799 ), #841, .F. ) ;
#7708=ORIENTED_EDGE ( 'NONE', *, *, #16245, .F. ) ;
#7711=ADVANCED_FACE ( 'NONE', ( #6645 ), #22710, .T. ) ;
#7713=B_SPLINE_CURVE_WITH_KNOTS ( 'NONE', 3,
 ( #13321, #1465, #23473, #30117, #15730, #10973 ),
 .UNSPECIFIED., .F., .F.,
 ( 4, 2, 4 ),
 ( 0.000000000000000000, 0.001045838473297321580, 0.002091676946594643160 ),
 .UNSPECIFIED. ) ;
#7716=ORIENTED_EDGE ( 'NONE', *, *, #18779, .T. ) ;
#7720=FACE_OUTER_BOUND ( 'NONE', #287, .T. ) ;
#7723=CARTESIAN_POINT ( 'NONE',  ( -55.93749999999995737, 1.962990915244752888, -3.400000000000188205 ) ) ;
#7726=CARTESIAN_POINT ( 'NONE',  ( -54.39999999999999147, 1.499999999999998002, 3.363870538531247067 ) ) ;
#7742=EDGE_CURVE ( 'NONE', #3419, #20255, #9673, .T. ) ;
#7756=CARTESIAN_POINT ( 'NONE',  ( -59.60065375968532209, -2.157866302380323731, 1.538217518236592474 ) ) ;
#7761=( BOUNDED_CURVE ( )  B_SPLINE_CURVE ( 2, ( #5242, #23843, #10016, #27084, #24717, #14748, #26210, #28582, #23695 ),
 .UNSPECIFIED., .F., .T. ) 
 B_SPLINE_CURVE_WITH_KNOTS ( ( 3, 2, 2, 2, 3 ),
 ( 0.6388888888888889506, 0.6481481481481481399, 0.6666666666666666297, 0.6851851851851852304, 0.6944444444444445308 ),
 .UNSPECIFIED. ) 
 CURVE ( )  GEOMETRIC_REPRESENTATION_ITEM ( )  RATIONAL_B_SPLINE_CURVE ( ( 0.9330127018922194093, 0.9330127018922197424, 1.000000000000000000, 0.8660254037844387076, 1.000000000000000000, 0.8660254037844387076, 1.000000000000000000, 0.9330127018922189652, 0.9330127018922194093 ) ) 
 REPRESENTATION_ITEM ( '' )  );
#7763=CARTESIAN_POINT ( 'NONE',  ( -59.82202994616204705, -4.156921938165296204, -2.272478542645976661E-13 ) ) ;
#7767=B_SPLINE_CURVE_WITH_KNOTS ( 'NONE', 3,
 ( #22316, #24971, #10263, #27034, #3297, #5345, #12943, #15010 ),
 .UNSPECIFIED., .F., .F.,
 ( 4, 2, 2, 4 ),
 ( 1.494941423529140449E-17, 0.001707980657444188501, 0.002561970986166275163, 0.003415961314888361824 ),
 .UNSPECIFIED. ) ;
#7788=ORIENTED_EDGE ( 'NONE', *, *, #12789, .F. ) ;
#7795=CARTESIAN_POINT ( 'NONE',  ( -61.00952994616203284, 3.117691453623994580, -1.800000000000202993 ) ) ;
#7797=CARTESIAN_POINT ( 'NONE',  ( -56.24999999999997868, -2.944486372867090918, 1.699999999999786349 ) ) ;
#7802=VERTEX_POINT ( 'NONE', #9339 ) ;
#7803=CARTESIAN_POINT ( 'NONE',  ( -59.22282295291818599, -3.176879556488940270, 1.263313363143568013 ) ) ;
#7804=CARTESIAN_POINT ( 'NONE',  ( -59.09999999999997300, 2.750000000000007994, -2.003569730682425015E-13 ) ) ;
#7807=CIRCLE ( 'NONE', #6818, 2.750000000000000000 ) ;
#7810=CARTESIAN_POINT ( 'NONE',  ( -59.60604010435355349, 3.187076279294280390, -1.184290838417780600 ) ) ;
#7812=CARTESIAN_POINT ( 'NONE',  ( -54.39999999999999147, 1.599999999999998090, 3.363870538531247512 ) ) ;
#7839=CARTESIAN_POINT ( 'NONE',  ( -59.89405989232412963, -3.920666489018293080E-15, 3.399999999999786304 ) ) ;
#7840=EDGE_CURVE ( 'NONE', #7345, #10060, #429, .T. ) ;
#7847=CARTESIAN_POINT ( 'NONE',  ( -59.69457535546589355, 2.411387898321005530, -1.235406689480260001 ) ) ;
#7867=ORIENTED_EDGE ( 'NONE', *, *, #15803, .F. ) ;
#7869=CARTESIAN_POINT ( 'NONE',  ( -59.69999999999997442, 3.400000000000007905, -2.001823990013003858E-13 ) ) ;
#7874=CARTESIAN_POINT ( 'NONE',  ( -44.49999999999997868, 2.650000000000008349, -1.494059622532430298E-13 ) ) ;
#7893=CARTESIAN_POINT ( 'NONE',  ( -58.51905989232412253, 2.944486372867082924, 1.699999999999820099 ) ) ;
#7897=CARTESIAN_POINT ( 'NONE',  ( -58.32202994616203995, -4.156921938165296204, -2.492539235493512031E-13 ) ) ;
#7898=DIRECTION ( 'NONE',  ( 1.344447539785323523E-44, -1.000000000000000000, -3.491481338843137300E-15 ) ) ;
#7913=TOROIDAL_SURFACE ( 'NONE', #29653, 4.199999999999954881, 0.1000000000000000056 ) ;
#7915=VERTEX_POINT ( 'NONE', #12782 ) ;
#7917=CARTESIAN_POINT ( 'NONE',  ( -59.50952994616202574, 3.117691453623994580, -1.800000000000197664 ) ) ;
#7918=CARTESIAN_POINT ( 'NONE',  ( -59.18789508915042319, 2.395752775956333291, 1.250136525132548915 ) ) ;
#7931=CARTESIAN_POINT ( 'NONE',  ( -57.38452994616203284, 2.093608279459370457E-14, -3.600000000000203926 ) ) ;
#7935=CARTESIAN_POINT ( 'NONE',  ( -56.64405989232412253, -2.944486372867073154, -1.700000000000216893 ) ) ;
#7952=VECTOR ( 'NONE', #20562, 1000.000000000000000 ) ;
#7954=CARTESIAN_POINT ( 'NONE',  ( -54.39999999999999147, -1.500000000000004663, 3.363870538531238186 ) ) ;
#7960=( BOUNDED_CURVE ( )  B_SPLINE_CURVE ( 3, ( #28665, #9028, #6981, #25486 ),
 .UNSPECIFIED., .F., .T. ) 
 B_SPLINE_CURVE_WITH_KNOTS ( ( 4, 4 ),
 ( 5.087525389280254551, 5.203235046317044699 ),
 .UNSPECIFIED. ) 
 CURVE ( )  GEOMETRIC_REPRESENTATION_ITEM ( )  RATIONAL_B_SPLINE_CURVE ( ( 1.000000000000000000, 0.9988845841160336469, 0.9988845841160336469, 1.000000000000000000 ) ) 
 REPRESENTATION_ITEM ( '' )  );
#7971=CARTESIAN_POINT ( 'NONE',  ( -60.13452994616204705, 3.117691453623979481, 1.799999999999798428 ) ) ;
#7990=CARTESIAN_POINT ( 'NONE',  ( -54.49999999999997868, 8.366749974758391359E-15, -1.938977325913827332E-13 ) ) ;
#7996=DIRECTION ( 'NONE',  ( 1.000000000000000000, -1.219044193948983948E-29, 3.491481338843133355E-15 ) ) ;
#8003=ORIENTED_EDGE ( 'NONE', *, *, #21296, .F. ) ;
#8012=CARTESIAN_POINT ( 'NONE',  ( -57.20655989232411542, 1.962990915244760659, -3.400000000000188205 ) ) ;
#8016=CARTESIAN_POINT ( 'NONE',  ( -60.76905989232411542, 2.944486372867092250, 1.699999999999795675 ) ) ;
#8022=AXIS2_PLACEMENT_3D ( 'NONE', #15672, #13261, #6166 ) ;
#8023=AXIS2_PLACEMENT_3D ( 'NONE', #23004, #28048, #17939 ) ;
#8041=ORIENTED_EDGE ( 'NONE', *, *, #2325, .F. ) ;
#8053=EDGE_CURVE ( 'NONE', #19715, #5500, #7767, .T. ) ;
#8055=CARTESIAN_POINT ( 'NONE',  ( -55.63452994616205416, 3.117691453623979481, 1.799999999999814415 ) ) ;
#8064=CARTESIAN_POINT ( 'NONE',  ( -58.75952994616203284, 3.117691453624006126, -1.800000000000174794 ) ) ;
#8082=CARTESIAN_POINT ( 'NONE',  ( -55.94702994616203995, -2.078460969082631227, -3.600000000000205258 ) ) ;
#8086=EDGE_CURVE ( 'NONE', #9490, #19242, #20340, .T. ) ;
#8096=CARTESIAN_POINT ( 'NONE',  ( -54.87499999999998579, -3.920666489018356189E-15, 3.399999999999804068 ) ) ;
#8102=CARTESIAN_POINT ( 'NONE',  ( -59.69464122902330416, 2.086944863889884871, 1.740854861534822273 ) ) ;
#8103=ORIENTED_EDGE ( 'NONE', *, *, #1306, .F. ) ;
#8121=VECTOR ( 'NONE', #26676, 1000.000000000000000 ) ;
#8123=CARTESIAN_POINT ( 'NONE',  ( -59.13452994616204705, -3.117691453623976816, 1.799999999999778000 ) ) ;
#8135=CARTESIAN_POINT ( 'NONE',  ( -44.59999999999995879, 1.433333333333357329, -4.054078878803043295 ) ) ;
#8146=VERTEX_POINT ( 'NONE', #16273 ) ;
#8148=EDGE_CURVE ( 'NONE', #13311, #3612, #577, .T. ) ;
#8149=CARTESIAN_POINT ( 'NONE',  ( -59.12165399575386004, 2.320602887402581249, 1.283384167747377846 ) ) ;
#8151=CARTESIAN_POINT ( 'NONE',  ( -55.93749999999996447, 1.962990915244749557, -3.400000000000189981 ) ) ;
#8152=CARTESIAN_POINT ( 'NONE',  ( -59.69620733439754190, 2.084614077930948550, 1.743567435612995986 ) ) ;
#8162=DIRECTION ( 'NONE',  ( 0.000000000000000000, 0.4295302013422852561, -0.9030524935654935526 ) ) ;
#8167=CARTESIAN_POINT ( 'NONE',  ( -57.33155989232411542, -1.962990915244706924, -3.400000000000209521 ) ) ;
#8173=CARTESIAN_POINT ( 'NONE',  ( -59.42430006944807275, 3.327103312532478263, 1.272610237773433184 ) ) ;
#8212=CARTESIAN_POINT ( 'NONE',  ( -57.00952994616205416, -7.288692778928185739E-15, 3.599999999999796696 ) ) ;
#8226=CARTESIAN_POINT ( 'NONE',  ( -44.59999999999999432, -1.400000000000007017, 3.959797974644484242 ) ) ;
#8228=CARTESIAN_POINT ( 'NONE',  ( -59.25952994616205416, -4.643455692769875931E-15, 3.599999999999788702 ) ) ;
#8238=FACE_OUTER_BOUND ( 'NONE', #18648, .T. ) ;
#8253=EDGE_CURVE ( 'NONE', #11810, #2222, #29365, .T. ) ;
#8256=CARTESIAN_POINT ( 'NONE',  ( -59.68687113065863059, -2.402179451507847396, -1.230958653213905851 ) ) ;
#8269=CARTESIAN_POINT ( 'NONE',  ( -54.89405989232412963, 2.944486372867106461, -1.700000000000182254 ) ) ;
#8276=CARTESIAN_POINT ( 'NONE',  ( -55.93749999999996447, 1.962990915244749557, -3.400000000000189981 ) ) ;
#8280=EDGE_CURVE ( 'NONE', #6307, #6992, #3614, .T. ) ;
#8284=CARTESIAN_POINT ( 'NONE',  ( -54.39999999999999147, 1.399999999999995914, 3.959797974644419849 ) ) ;
#8294=FACE_OUTER_BOUND ( 'NONE', #11412, .T. ) ;
#8299=CARTESIAN_POINT ( 'NONE',  ( -55.56249999999998579, -1.962990915244731793, 3.399999999999794742 ) ) ;
#8308=DIRECTION ( 'NONE',  ( 0.000000000000000000, -1.000000000000000000, -3.491481338843133355E-15 ) ) ;
#8313=CARTESIAN_POINT ( 'NONE',  ( -58.95655989232412253, -3.925981830489445379, -2.234056176427713674E-13 ) ) ;
#8331=ADVANCED_FACE ( 'NONE', ( #14672 ), #2640, .T. ) ;
#8341=CARTESIAN_POINT ( 'NONE',  ( -59.69999999999998153, -3.031840806488110385, 1.538811659727342906 ) ) ;
#8351=CARTESIAN_POINT ( 'NONE',  ( -55.88452994616203995, 2.093608279459368564E-14, -3.600000000000198597 ) ) ;
#8362=CARTESIAN_POINT ( 'NONE',  ( -57.44702994616203284, -2.078460969082625898, -3.600000000000213696 ) ) ;
#8365=ORIENTED_EDGE ( 'NONE', *, *, #8053, .F. ) ;
#8368=VERTEX_POINT ( 'NONE', #3427 ) ;
#8374=CARTESIAN_POINT ( 'NONE',  ( -59.14405989232412963, -2.099645193746120606E-14, 3.399999999999788969 ) ) ;
#8378=CARTESIAN_POINT ( 'NONE',  ( -58.94702994616203284, -2.078460969082631227, -3.600000000000215472 ) ) ;
#8393=FACE_OUTER_BOUND ( 'NONE', #20097, .T. ) ;
#8395=CARTESIAN_POINT ( 'NONE',  ( -59.69376084107991431, -2.238561451677897551, 1.535209479645327946 ) ) ;
#8400=CARTESIAN_POINT ( 'NONE',  ( -44.59999999999999432, -1.433333333333339343, 4.054078878802691577 ) ) ;
#8413=CARTESIAN_POINT ( 'NONE',  ( -59.62735476476905205, -2.346806195053343647, -1.237686616523553607 ) ) ;
#8425=EDGE_LOOP ( 'NONE', ( #16953, #17108, #16825 ) ) ;
#8427=CARTESIAN_POINT ( 'NONE',  ( -55.75952994616203995, 3.117691453623995024, -1.800000000000183897 ) ) ;
#8428=CARTESIAN_POINT ( 'NONE',  ( -59.01905989232412253, -2.944486372867088697, 1.699999999999779243 ) ) ;
#8434=CARTESIAN_POINT ( 'NONE',  ( -58.93749999999995737, 1.962990915244749557, -3.400000000000200640 ) ) ;
#8439=DIRECTION ( 'NONE',  ( -1.000000000000000000, 1.219044193948984088E-29, -3.491481338843133750E-15 ) ) ;
#8464=CARTESIAN_POINT ( 'NONE',  ( -57.37499999999996447, 2.944486372867106905, -1.700000000000191136 ) ) ;
#8465=CARTESIAN_POINT ( 'NONE',  ( -59.58735571801867792, 2.155141953262397436, 1.555030905555851106 ) ) ;
#8468=EDGE_LOOP ( 'NONE', ( #19733, #13047, #3038, #20329 ) ) ;
#8475=FACE_OUTER_BOUND ( 'NONE', #2929, .T. ) ;
#8480=CARTESIAN_POINT ( 'NONE',  ( -60.08155989232412253, 3.925981830489463142, -1.989569613369437003E-13 ) ) ;
#8518=AXIS2_PLACEMENT_3D ( 'NONE', #12496, #16957, #24239 ) ;
#8519=ORIENTED_EDGE ( 'NONE', *, *, #31318, .T. ) ;
#8520=TOROIDAL_SURFACE ( 'NONE', #14582, 2.750000000000000000, 0.1000000000000000056 ) ;
#8524=CARTESIAN_POINT ( 'NONE',  ( -59.13452994616204705, -3.117691453623983477, 1.799999999999766676 ) ) ;
#8530=CARTESIAN_POINT ( 'NONE',  ( -59.10189254050602869, 2.466111651538507310, -0.9699939413580190850 ) ) ;
#8534=VERTEX_POINT ( 'NONE', #20377 ) ;
#8536=EDGE_CURVE ( 'NONE', #16075, #26071, #4034, .T. ) ;
#8544=CARTESIAN_POINT ( 'NONE',  ( -59.35433616094501730, 2.309227654852833211, 1.299999087803395792 ) ) ;
#8545=CIRCLE ( 'NONE', #22222, 3.399999999999999911 ) ;
#8548=DIRECTION ( 'NONE',  ( -1.000000000000000000, 1.219044193948983948E-29, -3.491481338843133355E-15 ) ) ;
#8553=CARTESIAN_POINT ( 'NONE',  ( -54.93749999999998579, 1.962990915244722689, 3.399999999999812506 ) ) ;
#8561=ORIENTED_EDGE ( 'NONE', *, *, #26244, .F. ) ;
#8565=CARTESIAN_POINT ( 'NONE',  ( -59.66583922906154669, -2.374710448338320568, -1.229169263546879165 ) ) ;
#8567=ORIENTED_EDGE ( 'NONE', *, *, #4072, .F. ) ;
#8576=EDGE_LOOP ( 'NONE', ( #27039, #26553, #26747, #1964, #9577, #25764 ) ) ;
#8578=CARTESIAN_POINT ( 'NONE',  ( -55.13452994616203995, 2.181782848997977050E-14, -3.600000000000195932 ) ) ;
#8580=CARTESIAN_POINT ( 'NONE',  ( -58.51905989232412253, 2.944486372867092250, 1.699999999999803446 ) ) ;
#8588=CARTESIAN_POINT ( 'NONE',  ( -55.37499999999996447, -2.944486372867076707, -1.700000000000207345 ) ) ;
#8593=( BOUNDED_SURFACE ( )  B_SPLINE_SURFACE ( 3, 2, ( 
 ( #15143, #16798, #28826 ),
 ( #19905, #21871, #24943 ),
 ( #2542, #26593, #12192 ),
 ( #7847, #576, #26290 ) ),
 .UNSPECIFIED., .F., .F., .F. ) 
 B_SPLINE_SURFACE_WITH_KNOTS ( ( 4, 4 ),
 ( 3, 3 ),
 ( 5.086771802766119954, 5.213876728150149020 ),
 ( 0.000000000000000000, 1.000000000000000000 ),
 .UNSPECIFIED. ) 
 GEOMETRIC_REPRESENTATION_ITEM ( )  RATIONAL_B_SPLINE_SURFACE ( (
 ( 1.000000000000000000, 0.8113889037030935780, 1.000000000000000000),
 ( 1.000000000000000000, 0.8219112105083469233, 1.000000000000000000),
 ( 1.000000000000000000, 0.8319656872388402347, 1.000000000000000000),
 ( 1.000000000000000000, 0.8415238966082420058, 1.000000000000000000) ) ) 
 REPRESENTATION_ITEM ( '' )  SURFACE ( )  );
#8606=AXIS2_PLACEMENT_3D ( 'NONE', #28088, #6411, #5783 ) ;
#8610=CARTESIAN_POINT ( 'NONE',  ( -55.68749999999999289, 1.962990915244722689, 3.399999999999809841 ) ) ;
#8616=ORIENTED_EDGE ( 'NONE', *, *, #8148, .F. ) ;
#8621=CARTESIAN_POINT ( 'NONE',  ( -54.49999999999997158, -3.430639028629426601, -0.8101486624347474796 ) ) ;
#8629=TOROIDAL_SURFACE ( 'NONE', #19774, 3.524999999999996358, 0.1000000000000000056 ) ;
#8632=DIRECTION ( 'NONE',  ( 0.000000000000000000, -4.336808689942024836E-15, 1.000000000000000000 ) ) ;
#8633=EDGE_CURVE ( 'NONE', #17058, #11190, #11729, .T. ) ;
#8642=ORIENTED_EDGE ( 'NONE', *, *, #7085, .F. ) ;
#8650=ORIENTED_EDGE ( 'NONE', *, *, #10469, .T. ) ;
#8652=DIRECTION ( 'NONE',  ( 0.000000000000000000, -1.000000000000000000, -4.336808689942015369E-15 ) ) ;
#8655=LINE ( 'NONE', #10873, #7952 ) ;
#8656=CARTESIAN_POINT ( 'NONE',  ( -56.01905989232412963, -2.944486372867090918, 1.699999999999787015 ) ) ;
#8662=CARTESIAN_POINT ( 'NONE',  ( -54.69702994616206837, -2.078460969082657872, 3.599999999999797584 ) ) ;
#8663=VECTOR ( 'NONE', #8766, 1000.000000000000000 ) ;
#8671=ORIENTED_EDGE ( 'NONE', *, *, #24321, .T. ) ;
#8689=CARTESIAN_POINT ( 'NONE',  ( -59.40397935374117111, 2.384164297664157495, 1.250136525132547805 ) ) ;
#8690=ORIENTED_EDGE ( 'NONE', *, *, #30295, .F. ) ;
#8695=FACE_OUTER_BOUND ( 'NONE', #18389, .T. ) ;
#8697=EDGE_CURVE ( 'NONE', #22982, #8368, #12729, .T. ) ;
#8705=ORIENTED_EDGE ( 'NONE', *, *, #13622, .T. ) ;
#8717=DIRECTION ( 'NONE',  ( 0.000000000000000000, 1.000000000000000000, -8.673617379884030739E-15 ) ) ;
#8722=CARTESIAN_POINT ( 'NONE',  ( -54.57202994616206126, -4.156921938165296204, -2.089175772356712318E-13 ) ) ;
#8723=CARTESIAN_POINT ( 'NONE',  ( -57.83155989232412253, 3.925981830489463142, -1.911011283245466534E-13 ) ) ;
#8728=CARTESIAN_POINT ( 'NONE',  ( -56.81249999999997158, -1.962990915244707368, -3.400000000000208633 ) ) ;
#8750=CARTESIAN_POINT ( 'NONE',  ( -55.18749999999996447, 1.962990915244749557, -3.400000000000187317 ) ) ;
#8753=AXIS2_PLACEMENT_3D ( 'NONE', #17921, #5890, #9207 ) ;
#8764=ORIENTED_EDGE ( 'NONE', *, *, #5206, .F. ) ;
#8765=( BOUNDED_CURVE ( )  B_SPLINE_CURVE ( 3, ( #11449, #16049, #1953, #11278 ),
 .UNSPECIFIED., .F., .T. ) 
 B_SPLINE_CURVE_WITH_KNOTS ( ( 4, 4 ),
 ( 0.8682581838661508344, 1.057606415020297064 ),
 .UNSPECIFIED. ) 
 CURVE ( )  GEOMETRIC_REPRESENTATION_ITEM ( )  RATIONAL_B_SPLINE_CURVE ( ( 1.000000000000000000, 0.9970145015783106190, 0.9970145015783106190, 1.000000000000000000 ) ) 
 REPRESENTATION_ITEM ( '' )  );
#8766=DIRECTION ( 'NONE',  ( -3.491481338843133355E-15, -3.491481338843133355E-15, 1.000000000000000000 ) ) ;
#8771=ADVANCED_FACE ( 'NONE', ( #10513 ), #20189, .T. ) ;
#8784=EDGE_CURVE ( 'NONE', #14413, #16551, #2463, .T. ) ;
#8791=ORIENTED_EDGE ( 'NONE', *, *, #3790, .F. ) ;
#8793=VECTOR ( 'NONE', #30033, 1000.000000000000000 ) ;
#8805=CYLINDRICAL_SURFACE ( 'NONE', #26086, 0.1000000000000000472 ) ;
#8807=CARTESIAN_POINT ( 'NONE',  ( -57.25952994616203995, 3.117691453623994580, -1.800000000000189671 ) ) ;
#8811=ADVANCED_FACE ( 'NONE', ( #29204 ), #12182, .T. ) ;
#8817=CARTESIAN_POINT ( 'NONE',  ( -59.57202994616203995, 2.078460969082689846, -3.600000000000193268 ) ) ;
#8825=DIRECTION ( 'NONE',  ( -1.000000000000000000, 1.219044193948983948E-29, -3.491481338843133355E-15 ) ) ;
#8828=ORIENTED_EDGE ( 'NONE', *, *, #13570, .T. ) ;
#8839=FACE_OUTER_BOUND ( 'NONE', #21108, .T. ) ;
#8841=CIRCLE ( 'NONE', #4813, 2.649999999999999911 ) ;
#8846=ORIENTED_EDGE ( 'NONE', *, *, #14484, .F. ) ;
#8848=ADVANCED_FACE ( 'NONE', ( #18232 ), #25374, .T. ) ;
#8851=ADVANCED_FACE ( 'NONE', ( #6329 ), #25185, .F. ) ;
#8852=DIRECTION ( 'NONE',  ( -0.000000000000000000, 1.000000000000000000, 3.491481338843133355E-15 ) ) ;
#8860=AXIS2_PLACEMENT_3D ( 'NONE', #28394, #3851, #26004 ) ;
#8862=FACE_OUTER_BOUND ( 'NONE', #22448, .T. ) ;
#8878=( NAMED_UNIT ( * ) PLANE_ANGLE_UNIT ( ) SI_UNIT ( $, .RADIAN. ) );
#8879=ADVANCED_FACE ( 'NONE', ( #8238 ), #7913, .T. ) ;
#8880=CARTESIAN_POINT ( 'NONE',  ( -54.88452994616206126, 3.117691453623979481, 1.799999999999816858 ) ) ;
#8881=CARTESIAN_POINT ( 'NONE',  ( -58.20655989232411542, -3.925981830489445379, -2.207870066386390016E-13 ) ) ;
#8887=CARTESIAN_POINT ( 'NONE',  ( -56.31249999999998579, -1.962990915244731793, 3.399999999999792077 ) ) ;
#8906=CARTESIAN_POINT ( 'NONE',  ( -44.49999999999999289, -1.500000000000004663, 3.363870538531272825 ) ) ;
#8911=CIRCLE ( 'NONE', #5397, 0.1000000000000000472 ) ;
#8916=CARTESIAN_POINT ( 'NONE',  ( -55.25952994616203995, -3.117691453623963938, -1.800000000000207434 ) ) ;
#8935=DIRECTION ( 'NONE',  ( -1.000000000000000000, 1.219044193948983948E-29, -3.491481338843133355E-15 ) ) ;
#8948=CARTESIAN_POINT ( 'NONE',  ( -59.28507118137919463, -2.275557563509374326, 1.363277995769353934 ) ) ;
#8950=VECTOR ( 'NONE', #5991, 1000.000000000000000 ) ;
#8962=DIRECTION ( 'NONE',  ( 1.000000000000000000, -1.219044193948983948E-29, 3.491481338843133355E-15 ) ) ;
#8975=CYLINDRICAL_SURFACE ( 'NONE', #4924, 0.1000000000000000472 ) ;
#8985=CARTESIAN_POINT ( 'NONE',  ( -59.50952994616202574, 3.117691453623994580, -1.800000000000197664 ) ) ;
#8986=CARTESIAN_POINT ( 'NONE',  ( -59.19999999999996732, 3.264622394567737729, -0.9498634748674483763 ) ) ;
#8990=CIRCLE ( 'NONE', #25095, 3.399999999999999911 ) ;
#9008=CARTESIAN_POINT ( 'NONE',  ( -59.13463329438567229, -2.488830503680597328, -0.9121239897850130784 ) ) ;
#9018=AXIS2_PLACEMENT_3D ( 'NONE', #25987, #9060, #11596 ) ;
#9019=CARTESIAN_POINT ( 'NONE',  ( -59.38356253233095572, 2.342592582602649021, 1.264794915520445429 ) ) ;
#9027=CARTESIAN_POINT ( 'NONE',  ( -59.38281074049554320, 3.338301835134465101, 1.250136525132569787 ) ) ;
#9028=CARTESIAN_POINT ( 'NONE',  ( -59.27103329757905925, 2.428242106091510699, -1.066113908650129893 ) ) ;
#9035=DIRECTION ( 'NONE',  ( -1.000000000000000000, 1.219044193948983948E-29, -3.491481338843133355E-15 ) ) ;
#9038=AXIS2_PLACEMENT_3D ( 'NONE', #7599, #29579, #7898 ) ;
#9052=DIRECTION ( 'NONE',  ( 0.000000000000000000, -1.000000000000000000, -3.491481338843132961E-15 ) ) ;
#9053=ORIENTED_EDGE ( 'NONE', *, *, #14681, .T. ) ;
#9058=CARTESIAN_POINT ( 'NONE',  ( -58.95655989232412253, -3.925981830489445379, -2.234056176427713674E-13 ) ) ;
#9060=DIRECTION ( 'NONE',  ( 0.000000000000000000, 0.000000000000000000, 1.000000000000000000 ) ) ;
#9065=CARTESIAN_POINT ( 'NONE',  ( -60.12499999999997868, -3.920666489018291502E-15, 3.399999999999785860 ) ) ;
#9066=CARTESIAN_POINT ( 'NONE',  ( -59.19999999999997442, 8.366749974758448157E-15, -2.103076948839454410E-13 ) ) ;
#9085=AXIS2_PLACEMENT_3D ( 'NONE', #13233, #5814, #27824 ) ;
#9090=CARTESIAN_POINT ( 'NONE',  ( -59.99999999999997158, -2.944486372867089141, 1.699999999999775913 ) ) ;
#9109=ORIENTED_EDGE ( 'NONE', *, *, #10356, .F. ) ;
#9120=AXIS2_PLACEMENT_3D ( 'NONE', #23208, #27629, #1041 ) ;
#9132=( BOUNDED_CURVE ( )  B_SPLINE_CURVE ( 3, ( #21631, #26501, #2123, #28414 ),
 .UNSPECIFIED., .F., .T. ) 
 B_SPLINE_CURVE_WITH_KNOTS ( ( 4, 4 ),
 ( 5.097689251316671388, 5.213123141636014424 ),
 .UNSPECIFIED. ) 
 CURVE ( )  GEOMETRIC_REPRESENTATION_ITEM ( )  RATIONAL_B_SPLINE_CURVE ( ( 1.000000000000000000, 0.9988898929684264516, 0.9988898929684264516, 1.000000000000000000 ) ) 
 REPRESENTATION_ITEM ( '' )  );
#9135=CARTESIAN_POINT ( 'NONE',  ( -44.49999999999996447, 1.600000000000021627, -3.363870538531644971 ) ) ;
#9144=APPLICATION_CONTEXT ( 'automotive_design' ) ;
#9154=CARTESIAN_POINT ( 'NONE',  ( -57.88452994616205416, 3.117691453623979481, 1.799999999999806422 ) ) ;
#9155=CARTESIAN_POINT ( 'NONE',  ( -59.14880559183723108, -2.486640902962416799, -0.9502595626627227121 ) ) ;
#9162=AXIS2_PLACEMENT_3D ( 'NONE', #1252, #10615, #27239 ) ;
#9165=CARTESIAN_POINT ( 'NONE',  ( -59.66491930162565893, -1.010609427307466612, -3.600000000000221245 ) ) ;
#9174=ORIENTED_EDGE ( 'NONE', *, *, #28595, .F. ) ;
#9176=CARTESIAN_POINT ( 'NONE',  ( -59.46761860684627266, -2.377675374897907812, -1.175485268738968081 ) ) ;
#9187=LINE ( 'NONE', #18848, #11164 ) ;
#9196=CARTESIAN_POINT ( 'NONE',  ( -54.39999999999997726, 8.366749974758487600E-15, -2.213041600731273397E-13 ) ) ;
#9207=DIRECTION ( 'NONE',  ( 0.000000000000000000, 1.000000000000000000, 0.000000000000000000 ) ) ;
#9216=ORIENTED_EDGE ( 'NONE', *, *, #14012, .F. ) ;
#9218=ORIENTED_EDGE ( 'NONE', *, *, #7094, .F. ) ;
#9221=FACE_OUTER_BOUND ( 'NONE', #19280, .T. ) ;
#9224=EDGE_LOOP ( 'NONE', ( #3865, #309, #29515, #5845 ) ) ;
#9228=CARTESIAN_POINT ( 'NONE',  ( -60.37499999999995737, 2.944486372867106905, -1.700000000000201794 ) ) ;
#9252=CARTESIAN_POINT ( 'NONE',  ( -54.44702994616203995, -2.078460969082631227, -3.600000000000199485 ) ) ;
#9253=ORIENTED_EDGE ( 'NONE', *, *, #21296, .T. ) ;
#9259=CARTESIAN_POINT ( 'NONE',  ( -57.50952994616203995, -3.117691453623963938, -1.800000000000215206 ) ) ;
#9280=DIRECTION ( 'NONE',  ( 0.000000000000000000, -1.000000000000000000, -3.491481338843133355E-15 ) ) ;
#9282=CIRCLE ( 'NONE', #3211, 3.624999999999996447 ) ;
#9286=ORIENTED_EDGE ( 'NONE', *, *, #16418, .F. ) ;
#9294=LINE ( 'NONE', #6921, #1909 ) ;
#9297=FACE_OUTER_BOUND ( 'NONE', #24923, .T. ) ;
#9300=EDGE_CURVE ( 'NONE', #11459, #30275, #25634, .T. ) ;
#9307=CARTESIAN_POINT ( 'NONE',  ( -56.07202994616204705, -4.156921938165296204, -2.141547992439359634E-13 ) ) ;
#9314=ORIENTED_EDGE ( 'NONE', *, *, #19570, .T. ) ;
#9319=CARTESIAN_POINT ( 'NONE',  ( -59.69999999999997442, -3.237160264815294841, -1.238538609462289219 ) ) ;
#9339=CARTESIAN_POINT ( 'NONE',  ( -55.81249999999997868, 3.400000000000007905, -1.865662262041272555E-13 ) ) ;
#9346=B_SPLINE_CURVE_WITH_KNOTS ( 'NONE', 3,
 ( #3396, #13649, #10814, #20349, #13496, #30588, #23188, #3550, #1470, #23333, #1615, #11130, #13042, #30126, #20956, #22724 ),
 .UNSPECIFIED., .F., .F.,
 ( 4, 3, 3, 3, 3, 4 ),
 ( -2.177409780395868905E-06, 0.000000000000000000, 1.647199373531835971E-05, 5.453032561112356195E-05, 8.914430023005045502E-05, 0.0001239676331529235916 ),
 .UNSPECIFIED. ) ;
#9348=FACE_OUTER_BOUND ( 'NONE', #11422, .T. ) ;
#9349=EDGE_CURVE ( 'NONE', #556, #10413, #18065, .T. ) ;
#9352=DIRECTION ( 'NONE',  ( -3.491481338843133355E-15, -3.491481338843133355E-15, 1.000000000000000000 ) ) ;
#9370=ORIENTED_EDGE ( 'NONE', *, *, #18752, .T. ) ;
#9374=CARTESIAN_POINT ( 'NONE',  ( -44.59999999999996589, -1.599999999999981215, -3.363870538531657850 ) ) ;
#9375=VERTEX_POINT ( 'NONE', #29492 ) ;
#9379=CARTESIAN_POINT ( 'NONE',  ( -60.99999999999997158, 2.944486372867092250, 1.699999999999795008 ) ) ;
#9389=CARTESIAN_POINT ( 'NONE',  ( -54.39999999999999147, 1.399999999999996136, 3.959797974644419849 ) ) ;
#9406=CARTESIAN_POINT ( 'NONE',  ( -59.49999999999997158, 2.944486372867092250, 1.699999999999800115 ) ) ;
#9414=CARTESIAN_POINT ( 'NONE',  ( -57.75952994616205416, -4.643455692769894075E-15, 3.599999999999794031 ) ) ;
#9417=EDGE_CURVE ( 'NONE', #11849, #9375, #12476, .T. ) ;
#9430=CARTESIAN_POINT ( 'NONE',  ( -54.46614378277664059, -2.255560380866761250, -2.805788190199900889 ) ) ;
#9441=EDGE_LOOP ( 'NONE', ( #16704, #8828, #23110, #663, #15315, #5377, #7108, #18670 ) ) ;
#9445=ORIENTED_EDGE ( 'NONE', *, *, #19784, .F. ) ;
#9447=CARTESIAN_POINT ( 'NONE',  ( -59.09999999999998010, -2.331118226142294247, 1.260312586522342349 ) ) ;
#9450=CIRCLE ( 'NONE', #4863, 0.1000000000000000472 ) ;
#9451=EDGE_CURVE ( 'NONE', #8146, #24802, #7713, .T. ) ;
#9456=ORIENTED_EDGE ( 'NONE', *, *, #14437, .T. ) ;
#9464=ORIENTED_EDGE ( 'NONE', *, *, #16414, .F. ) ;
#9466=ADVANCED_FACE ( 'NONE', ( #20801 ), #18583, .T. ) ;
#9473=CARTESIAN_POINT ( 'NONE',  ( -57.13452994616205416, 3.117691453623979481, 1.799999999999809086 ) ) ;
#9477=CARTESIAN_POINT ( 'NONE',  ( -58.68749999999998579, 1.962990915244717138, 3.399999999999802291 ) ) ;
#9480=CARTESIAN_POINT ( 'NONE',  ( -59.69999999999997442, -3.399999999999991473, -2.235080921937235780E-13 ) ) ;
#9482=DIRECTION ( 'NONE',  ( 1.000000000000000000, -1.219044193948983948E-29, 3.491481338843133355E-15 ) ) ;
#9484=ADVANCED_FACE ( 'NONE', ( #10666 ), #15871, .T. ) ;
#9486=AXIS2_PLACEMENT_3D ( 'NONE', #9135, #8962, #4208 ) ;
#9490=VERTEX_POINT ( 'NONE', #1611 ) ;
#9502=CARTESIAN_POINT ( 'NONE',  ( -44.59999999999998721, -1.600000000000004530, 3.363870538531271936 ) ) ;
#9503=AXIS2_PLACEMENT_3D ( 'NONE', #7138, #9525, #10387 ) ;
#9505=LINE ( 'NONE', #28484, #16582 ) ;
#9509=CYLINDRICAL_SURFACE ( 'NONE', #632, 0.1000000000000000472 ) ;
#9516=AXIS2_PLACEMENT_3D ( 'NONE', #17381, #24360, #29557 ) ;
#9525=DIRECTION ( 'NONE',  ( -3.491481338843133355E-15, -3.491481338843133355E-15, 1.000000000000000000 ) ) ;
#9527=EDGE_CURVE ( 'NONE', #26147, #1670, #20703, .T. ) ;
#9555=ORIENTED_EDGE ( 'NONE', *, *, #18781, .F. ) ;
#9556=CARTESIAN_POINT ( 'NONE',  ( -54.57202994616205416, -4.156921938165296204, -2.089175772356712570E-13 ) ) ;
#9569=EDGE_CURVE ( 'NONE', #8368, #11984, #6538, .T. ) ;
#9577=ORIENTED_EDGE ( 'NONE', *, *, #21026, .T. ) ;
#9579=CARTESIAN_POINT ( 'NONE',  ( -60.62499999999995737, -2.944486372867076707, -1.700000000000225775 ) ) ;
#9588=CARTESIAN_POINT ( 'NONE',  ( -58.50952994616205416, -4.643455692769885398E-15, 3.599999999999791367 ) ) ;
#9593=VERTEX_POINT ( 'NONE', #6224 ) ;
#9599=CARTESIAN_POINT ( 'NONE',  ( -59.19999999999997442, -3.222669219888746550, 1.250136525132528931 ) ) ;
#9605=CARTESIAN_POINT ( 'NONE',  ( -59.60604010435355349, 3.187076279294280390, -1.184290838417780600 ) ) ;
#9606=DIRECTION ( 'NONE',  ( -1.000000000000000000, 1.219044193948983948E-29, -3.491481338843133355E-15 ) ) ;
#9620=EDGE_LOOP ( 'NONE', ( #16962, #17829, #7459, #25452 ) ) ;
#9628=CARTESIAN_POINT ( 'NONE',  ( -59.53056271719990633, 2.463209972446164908, -1.140713948626884244 ) ) ;
#9631=CIRCLE ( 'NONE', #27299, 3.624999999999996447 ) ;
#9633=CARTESIAN_POINT ( 'NONE',  ( -55.76905989232411542, 2.023778652682505897E-14, -3.400000000000197975 ) ) ;
#9634=EDGE_CURVE ( 'NONE', #14659, #24201, #26675, .T. ) ;
#9635=CARTESIAN_POINT ( 'NONE',  ( -59.09999999999997300, -2.465712773623968790, -0.9709585562669303949 ) ) ;
#9636=CIRCLE ( 'NONE', #10126, 0.1000000000000001166 ) ;
#9645=ORIENTED_EDGE ( 'NONE', *, *, #24321, .F. ) ;
#9663=CARTESIAN_POINT ( 'NONE',  ( -44.59999999999999432, 1.399999999999995692, 4.029888335921785192 ) ) ;
#9665=CYLINDRICAL_SURFACE ( 'NONE', #10399, 3.399999999999999911 ) ;
#9673=CIRCLE ( 'NONE', #23817, 3.524999999999996358 ) ;
#9682=LINE ( 'NONE', #12053, #11557 ) ;
#9693=ORIENTED_EDGE ( 'NONE', *, *, #10815, .T. ) ;
#9694=CARTESIAN_POINT ( 'NONE',  ( -59.62447745295619939, -2.166872014472563279, 1.529642084025434556 ) ) ;
#9702=CARTESIAN_POINT ( 'NONE',  ( -56.32202994616206126, 2.078460969082646770, 3.599999999999807354 ) ) ;
#9720=CARTESIAN_POINT ( 'NONE',  ( -54.39999999999999147, -1.400000000000006795, 3.959797974644449603 ) ) ;
#9723=ORIENTED_EDGE ( 'NONE', *, *, #15195, .T. ) ;
#9726=CARTESIAN_POINT ( 'NONE',  ( -58.50952994616205416, -4.643455692769885398E-15, 3.599999999999791367 ) ) ;
#9732=CARTESIAN_POINT ( 'NONE',  ( -56.19702994616206837, -2.078460969082657872, 3.599999999999791811 ) ) ;
#9752=LINE ( 'NONE', #14494, #17887 ) ;
#9763=ORIENTED_EDGE ( 'NONE', *, *, #9417, .T. ) ;
#9768=FACE_OUTER_BOUND ( 'NONE', #26838, .T. ) ;
#9770=CARTESIAN_POINT ( 'NONE',  ( -56.95655989232412963, 1.962990915244722245, 3.399999999999804956 ) ) ;
#9798=CARTESIAN_POINT ( 'NONE',  ( -44.59999999999999432, 1.399999999999995914, 3.959797974644454044 ) ) ;
#9812=CARTESIAN_POINT ( 'NONE',  ( -59.38710602098247193, 3.262177753127958102, -1.057889186448619512 ) ) ;
#9817=VERTEX_POINT ( 'NONE', #2675 ) ;
#9838=ORIENTED_EDGE ( 'NONE', *, *, #6125, .F. ) ;
#9840=TOROIDAL_SURFACE ( 'NONE', #21969, 3.524999999999996358, 0.1000000000000000056 ) ;
#9841=EDGE_CURVE ( 'NONE', #13311, #20255, #15540, .T. ) ;
#9843=CARTESIAN_POINT ( 'NONE',  ( -59.57202994616203995, 2.078460969082674747, -3.600000000000202593 ) ) ;
#9850=CIRCLE ( 'NONE', #30066, 4.300000000000016698 ) ;
#9857=CARTESIAN_POINT ( 'NONE',  ( -54.49999999999998579, 1.514093959731539263, 3.183260039818149423 ) ) ;
#9876=CARTESIAN_POINT ( 'NONE',  ( -56.13452994616205416, -3.117691453623976816, 1.799999999999788436 ) ) ;
#9878=CARTESIAN_POINT ( 'NONE',  ( -56.43749999999998579, 1.962990915244719803, 3.399999999999808509 ) ) ;
#9884=CARTESIAN_POINT ( 'NONE',  ( -55.06249999999997158, 3.925981830489463142, -1.814330073843579337E-13 ) ) ;
#9894=DIRECTION ( 'NONE',  ( -1.000000000000000000, 1.219044193948983948E-29, -3.491481338843133355E-15 ) ) ;
#9918=DIRECTION ( 'NONE',  ( 0.000000000000000000, -1.000000000000000000, -1.715124499442879341E-15 ) ) ;
#9919=CYLINDRICAL_SURFACE ( 'NONE', #2642, 3.399999999999999911 ) ;
#9923=CARTESIAN_POINT ( 'NONE',  ( -55.89405989232412253, -2.944486372867076263, -1.700000000000208900 ) ) ;
#9934=CARTESIAN_POINT ( 'NONE',  ( -58.95655989232411542, -3.399999999999991029, -2.281093130107142867E-13 ) ) ;
#9964=CARTESIAN_POINT ( 'NONE',  ( -57.93749999999998579, 1.962990915244718026, 3.399999999999803624 ) ) ;
#9966=AXIS2_PLACEMENT_3D ( 'NONE', #22868, #20345, #13182 ) ;
#9988=CARTESIAN_POINT ( 'NONE',  ( -54.49227792872101617, -2.349139337603836530, -2.680014161610996037 ) ) ;
#10010=CARTESIAN_POINT ( 'NONE',  ( -56.88452994616205416, -3.117691453623976816, 1.799999999999785993 ) ) ;
#10016=CARTESIAN_POINT ( 'NONE',  ( -58.64405989232411542, 2.944486372867117563, -1.700000000000176259 ) ) ;
#10024=ORIENTED_EDGE ( 'NONE', *, *, #8633, .T. ) ;
#10026=VECTOR ( 'NONE', #4746, 1000.000000000000000 ) ;
#10029=DIRECTION ( 'NONE',  ( -1.000000000000000000, 1.219044193948983948E-29, -3.491481338843133355E-15 ) ) ;
#10040=CARTESIAN_POINT ( 'NONE',  ( -54.39405989232412253, -2.944486372867076263, -1.700000000000203793 ) ) ;
#10041=ORIENTED_EDGE ( 'NONE', *, *, #7588, .F. ) ;
#10047=CARTESIAN_POINT ( 'NONE',  ( -59.23418654921033522, -3.153953023162030078, 1.269874138521803975 ) ) ;
#10055=CARTESIAN_POINT ( 'NONE',  ( -59.69999999999997442, 3.166389444283797872, -1.238538609462263462 ) ) ;
#10057=DIRECTION ( 'NONE',  ( 0.000000000000000000, -1.000000000000000000, -3.491481338843133355E-15 ) ) ;
#10059=EDGE_CURVE ( 'NONE', #7802, #1825, #22091, .T. ) ;
#10060=VERTEX_POINT ( 'NONE', #17385 ) ;
#10065=CARTESIAN_POINT ( 'NONE',  ( -54.74999999999997868, -2.944486372867089141, 1.699999999999794342 ) ) ;
#10075=DIRECTION ( 'NONE',  ( -3.491481338843133355E-15, -3.491481338843133355E-15, 1.000000000000000000 ) ) ;
#10077=CARTESIAN_POINT ( 'NONE',  ( -59.69999999999997442, 8.366749974758454467E-15, -2.120534355533670266E-13 ) ) ;
#10079=CARTESIAN_POINT ( 'NONE',  ( -56.51905989232411542, 2.023778652682506843E-14, -3.400000000000200640 ) ) ;
#10098=ORIENTED_EDGE ( 'NONE', *, *, #1087, .F. ) ;
#10099=SURFACE_SIDE_STYLE ('',( #2802 ) ) ;
#10112=CARTESIAN_POINT ( 'NONE',  ( -55.84599364905386665, 3.400000000000011902, -0.9110272542660028394 ) ) ;
#10119=ORIENTED_EDGE ( 'NONE', *, *, #30959, .T. ) ;
#10123=DIRECTION ( 'NONE',  ( 0.000000000000000000, 1.000000000000000000, 3.491481338843130594E-15 ) ) ;
#10126=AXIS2_PLACEMENT_3D ( 'NONE', #23357, #20979, #8162 ) ;
#10143=CARTESIAN_POINT ( 'NONE',  ( -59.18987816865176654, 2.399875262006965215, 1.250136525132548915 ) ) ;
#10149=EDGE_LOOP ( 'NONE', ( #15248, #20159, #24888, #25915 ) ) ;
#10152=CARTESIAN_POINT ( 'NONE',  ( -58.32202994616204705, -4.156921938165296204, -2.220106322563329850E-13 ) ) ;
#10156=CARTESIAN_POINT ( 'NONE',  ( -56.74005354137802470, -3.399999999999994138, 0.9110272542655987182 ) ) ;
#10161=FACE_OUTER_BOUND ( 'NONE', #9441, .T. ) ;
#10166=DIRECTION ( 'NONE',  ( 0.000000000000000000, 1.000000000000000000, 3.491481338843137694E-15 ) ) ;
#10181=CARTESIAN_POINT ( 'NONE',  ( -58.88452994616202574, 2.093608279459372350E-14, -3.600000000000208811 ) ) ;
#10202=LINE ( 'NONE', #19871, #5174 ) ;
#10212=VERTEX_POINT ( 'NONE', #24113 ) ;
#10227=CARTESIAN_POINT ( 'NONE',  ( -60.44702994616202574, -2.078460969082631227, -3.600000000000220801 ) ) ;
#10242=ORIENTED_EDGE ( 'NONE', *, *, #12789, .T. ) ;
#10249=ORIENTED_EDGE ( 'NONE', *, *, #8784, .T. ) ;
#10254=VERTEX_POINT ( 'NONE', #7489 ) ;
#10256=CARTESIAN_POINT ( 'NONE',  ( -59.69459045457838187, 2.420214307862085246, -1.235415406956913653 ) ) ;
#10257=EDGE_CURVE ( 'NONE', #9817, #30573, #20576, .T. ) ;
#10263=CARTESIAN_POINT ( 'NONE',  ( -59.69999999999993889, -0.8057164866800677894, -3.484314813711807624 ) ) ;
#10268=EDGE_CURVE ( 'NONE', #556, #24802, #26112, .T. ) ;
#10270=CYLINDRICAL_SURFACE ( 'NONE', #1797, 3.399999999999999911 ) ;
#10279=ORIENTED_EDGE ( 'NONE', *, *, #19396, .T. ) ;
#10284=CIRCLE ( 'NONE', #5747, 2.649999999999999911 ) ;
#10290=ORIENTED_EDGE ( 'NONE', *, *, #20931, .T. ) ;
#10291=CARTESIAN_POINT ( 'NONE',  ( -59.57202994616203995, 2.078460969082674747, -3.600000000000202593 ) ) ;
#10299=CARTESIAN_POINT ( 'NONE',  ( -59.13452994616204705, -3.117691453623976816, 1.799999999999778000 ) ) ;
#10315=( BOUNDED_CURVE ( )  B_SPLINE_CURVE ( 2, ( #30660, #6141, #8656, #23394, #18336, #27972, #25595, #1534, #11193 ),
 .UNSPECIFIED., .F., .T. ) 
 B_SPLINE_CURVE_WITH_KNOTS ( ( 3, 2, 2, 2, 3 ),
 ( 0.2500000000000000000, 0.2592592592592592449, 0.2777777777777777901, 0.2962962962962962798, 0.3055555555555555802 ),
 .UNSPECIFIED. ) 
 CURVE ( )  GEOMETRIC_REPRESENTATION_ITEM ( )  RATIONAL_B_SPLINE_CURVE ( ( 0.9330127018922192983, 0.9330127018922194093, 1.000000000000000000, 0.8660254037844387076, 1.000000000000000000, 0.8660254037844387076, 1.000000000000000000, 0.9330127018922191873, 0.9330127018922194093 ) ) 
 REPRESENTATION_ITEM ( '' )  );
#10331=CARTESIAN_POINT ( 'NONE',  ( -60.00952994616204705, -4.643455692769866465E-15, 3.599999999999786038 ) ) ;
#10356=EDGE_CURVE ( 'NONE', #17058, #26017, #5573, .T. ) ;
#10372=DIRECTION ( 'NONE',  ( 1.000000000000000000, -1.219044193948983948E-29, 3.491481338843133355E-15 ) ) ;
#10377=CARTESIAN_POINT ( 'NONE',  ( -60.33155989232410121, -1.962990915244706924, -3.400000000000220179 ) ) ;
#10380=CARTESIAN_POINT ( 'NONE',  ( -59.19126343180466421, -2.406052454186071277, 1.245092465133171844 ) ) ;
#10385=CARTESIAN_POINT ( 'NONE',  ( -59.09664939113120852, -2.332125100258536143, 1.258448456133006710 ) ) ;
#10387=DIRECTION ( 'NONE',  ( 0.000000000000000000, 1.000000000000000000, 0.000000000000000000 ) ) ;
#10389=ORIENTED_EDGE ( 'NONE', *, *, #2095, .F. ) ;
#10397=CARTESIAN_POINT ( 'NONE',  ( -59.69142724121850563, -2.412383461849193278, -1.233589124872107146 ) ) ;
#10399=AXIS2_PLACEMENT_3D ( 'NONE', #6971, #21862, #24970 ) ;
#10407=DIRECTION ( 'NONE',  ( -1.000000000000000000, 1.219044193948983948E-29, -3.491481338843133355E-15 ) ) ;
#10413=VERTEX_POINT ( 'NONE', #30396 ) ;
#10415=CARTESIAN_POINT ( 'NONE',  ( -56.06249999999995737, -1.962990915244703816, -3.400000000000207745 ) ) ;
#10418=AXIS2_PLACEMENT_3D ( 'NONE', #23605, #1724, #2057 ) ;
#10421=CARTESIAN_POINT ( 'NONE',  ( -55.25952994616203995, -3.117691453623963938, -1.800000000000207434 ) ) ;
#10423=AXIS2_PLACEMENT_3D ( 'NONE', #28930, #7700, #7241 ) ;
#10426=AXIS2_PLACEMENT_3D ( 'NONE', #30252, #10776, #29939 ) ;
#10438=ORIENTED_EDGE ( 'NONE', *, *, #23484, .F. ) ;
#10443=CARTESIAN_POINT ( 'NONE',  ( -59.16035890245980511, 2.496590366952375017, -0.9473018300160132021 ) ) ;
#10444=CARTESIAN_POINT ( 'NONE',  ( -54.48133250964848884, -2.367385699161606016, -2.689772239255368902 ) ) ;
#10455=CARTESIAN_POINT ( 'NONE',  ( -56.00952994616203995, -3.117691453623963938, -1.800000000000210099 ) ) ;
#10464=CARTESIAN_POINT ( 'NONE',  ( -60.44702994616202574, -2.078460969082631227, -3.600000000000220801 ) ) ;
#10468=DIRECTION ( 'NONE',  ( 0.000000000000000000, 1.000000000000000000, 0.000000000000000000 ) ) ;
#10469=EDGE_CURVE ( 'NONE', #6234, #6022, #13426, .T. ) ;
#10489=CARTESIAN_POINT ( 'NONE',  ( -54.39999999999999147, 1.499999999999996003, 3.959797974644419849 ) ) ;
#10505=CARTESIAN_POINT ( 'NONE',  ( -60.44702994616202574, -2.078460969082631227, -3.600000000000220801 ) ) ;
#10506=ORIENTED_EDGE ( 'NONE', *, *, #30536, .F. ) ;
#10510=CARTESIAN_POINT ( 'NONE',  ( -54.49999999999996447, 1.600000000000021627, -3.363870538531680054 ) ) ;
#10513=FACE_OUTER_BOUND ( 'NONE', #928, .T. ) ;
#10519=VECTOR ( 'NONE', #4067, 1000.000000000000000 ) ;
#10532=VERTEX_POINT ( 'NONE', #25813 ) ;
#10533=CARTESIAN_POINT ( 'NONE',  ( -59.10142724674265935, 2.309330906357313307, 1.299824891736185206 ) ) ;
#10535=CARTESIAN_POINT ( 'NONE',  ( -58.18749999999995737, 1.962990915244749557, -3.400000000000197531 ) ) ;
#10541=ORIENTED_EDGE ( 'NONE', *, *, #10815, .F. ) ;
#10548=CARTESIAN_POINT ( 'NONE',  ( -59.83155989232413674, -1.962990915244731571, 3.399999999999779199 ) ) ;
#10554=LINE ( 'NONE', #22903, #15493 ) ;
#10559=FACE_OUTER_BOUND ( 'NONE', #1278, .T. ) ;
#10563=DIRECTION ( 'NONE',  ( 1.000000000000000000, -1.219044193948983948E-29, 3.491481338843133355E-15 ) ) ;
#10590=ADVANCED_FACE ( 'NONE', ( #17402 ), #5517, .T. ) ;
#10592=EDGE_CURVE ( 'NONE', #28731, #4847, #19648, .T. ) ;
#10595=CARTESIAN_POINT ( 'NONE',  ( -59.19702994616205416, -2.078460969082660537, 3.599999999999779821 ) ) ;
#10604=CARTESIAN_POINT ( 'NONE',  ( -54.48513940398811428, -2.374617027978079609, -2.675739047658152625 ) ) ;
#10608=CARTESIAN_POINT ( 'NONE',  ( -59.69999999999997442, 3.400000000000007905, -2.001823990013003858E-13 ) ) ;
#10611=CARTESIAN_POINT ( 'NONE',  ( -57.00952994616205416, -4.643455692769903542E-15, 3.599999999999796696 ) ) ;
#10615=DIRECTION ( 'NONE',  ( 1.000000000000000000, -1.219044193948983948E-29, 3.491481338843133355E-15 ) ) ;
#10628=CARTESIAN_POINT ( 'NONE',  ( -59.69873842481536030, -2.257036478699359972, 1.538083288954898542 ) ) ;
#10629=CARTESIAN_POINT ( 'NONE',  ( -56.87499999999996447, -2.944486372867073598, -1.700000000000217781 ) ) ;
#10635=ORIENTED_EDGE ( 'NONE', *, *, #29326, .T. ) ;
#10636=( BOUNDED_CURVE ( )  B_SPLINE_CURVE ( 3, ( #17290, #15063, #26474, #19520 ),
 .UNSPECIFIED., .F., .T. ) 
 B_SPLINE_CURVE_WITH_KNOTS ( ( 4, 4 ),
 ( 4.242719404917985493, 4.329617956773491372 ),
 .UNSPECIFIED. ) 
 CURVE ( )  GEOMETRIC_REPRESENTATION_ITEM ( )  RATIONAL_B_SPLINE_CURVE ( ( 1.000000000000000000, 0.9993708191325071377, 0.9993708191325071377, 1.000000000000000000 ) ) 
 REPRESENTATION_ITEM ( '' )  );
#10638=CYLINDRICAL_SURFACE ( 'NONE', #8753, 0.1000000000000000472 ) ;
#10640=CARTESIAN_POINT ( 'NONE',  ( -59.61160122551025609, -2.340542558125645822, -1.243912201914837423 ) ) ;
#10650=DIRECTION ( 'NONE',  ( 1.000000000000000000, -1.219044193948983948E-29, 3.491481338843133355E-15 ) ) ;
#10655=CARTESIAN_POINT ( 'NONE',  ( -54.64405989232413674, -3.920666489018357767E-15, 3.399999999999804512 ) ) ;
#10656=ORIENTED_EDGE ( 'NONE', *, *, #26854, .F. ) ;
#10662=CARTESIAN_POINT ( 'NONE',  ( -56.93749999999997158, -3.925981830489445379, -2.163561077067149631E-13 ) ) ;
#10666=FACE_OUTER_BOUND ( 'NONE', #17919, .T. ) ;
#10676=CARTESIAN_POINT ( 'NONE',  ( -59.69142724121850563, -2.412383461849193278, -1.233589124872107146 ) ) ;
#10681=CARTESIAN_POINT ( 'NONE',  ( -55.31249999999997158, -1.962990915244707368, -3.400000000000203304 ) ) ;
#10693=CARTESIAN_POINT ( 'NONE',  ( -58.87499999999996447, 2.944486372867118007, -1.700000000000177147 ) ) ;
#10695=CARTESIAN_POINT ( 'NONE',  ( -58.89405989232411542, -2.944486372867076263, -1.700000000000219558 ) ) ;
#10702=CARTESIAN_POINT ( 'NONE',  ( -59.49038236770705623, 3.145408112564967773, 1.387068135838901428 ) ) ;
#10704=DIRECTION ( 'NONE',  ( -1.000000000000000000, 1.219044193948983948E-29, -3.491481338843133355E-15 ) ) ;
#10710=EDGE_LOOP ( 'NONE', ( #15384, #19596, #31067, #17692 ) ) ;
#10716=CYLINDRICAL_SURFACE ( 'NONE', #9085, 0.1000000000000000472 ) ;
#10729=CARTESIAN_POINT ( 'NONE',  ( -54.51905989232412963, -2.944486372867088697, 1.699999999999795008 ) ) ;
#10740=CARTESIAN_POINT ( 'NONE',  ( -58.19702994616203284, -2.078460969082624565, -3.600000000000216360 ) ) ;
#10752=CARTESIAN_POINT ( 'NONE',  ( -59.08155989232413674, -1.962990915244734236, 3.399999999999780975 ) ) ;
#10756=CARTESIAN_POINT ( 'NONE',  ( -57.75952994616205416, -4.643455692769894075E-15, 3.599999999999794031 ) ) ;
#10762=CARTESIAN_POINT ( 'NONE',  ( -59.59999999999998721, 2.022492213459062160, 1.712315755489264513 ) ) ;
#10776=DIRECTION ( 'NONE',  ( -1.727378680347082743E-15, 0.9428090415820579162, -0.3333333333333488580 ) ) ;
#10777=DIRECTION ( 'NONE',  ( -3.491481338843133355E-15, -3.491481338843133355E-15, 1.000000000000000000 ) ) ;
#10781=EDGE_CURVE ( 'NONE', #18960, #15811, #19152, .T. ) ;
#10798=CARTESIAN_POINT ( 'NONE',  ( -57.76905989232412963, 2.944486372867092250, 1.699999999999806111 ) ) ;
#10803=CARTESIAN_POINT ( 'NONE',  ( -58.68749999999998579, 1.962990915244722689, 3.399999999999799627 ) ) ;
#10805=LINE ( 'NONE', #20489, #30419 ) ;
#10812=EDGE_CURVE ( 'NONE', #17625, #1825, #24914, .T. ) ;
#10814=CARTESIAN_POINT ( 'NONE',  ( -59.60127941732040568, 2.337454683939000688, -1.248534441610057444 ) ) ;
#10815=EDGE_CURVE ( 'NONE', #21074, #16500, #11676, .T. ) ;
#10816=CARTESIAN_POINT ( 'NONE',  ( -59.69619597676793887, 2.090631638210891374, 1.743547763621478452 ) ) ;
#10821=ORIENTED_EDGE ( 'NONE', *, *, #15594, .T. ) ;
#10823=DIRECTION ( 'NONE',  ( 1.000000000000000000, -1.219044193948983948E-29, 3.491481338843133355E-15 ) ) ;
#10826=CARTESIAN_POINT ( 'NONE',  ( -59.11151511461849850, 2.314313660749603763, 1.291265858342419248 ) ) ;
#10830=CARTESIAN_POINT ( 'NONE',  ( -56.43749999999998579, 1.962990915244722689, 3.399999999999807621 ) ) ;
#10839=CARTESIAN_POINT ( 'NONE',  ( -59.43788607448336592, -2.385332005665353972, -1.158943404468679494 ) ) ;
#10843=CARTESIAN_POINT ( 'NONE',  ( -59.39405989232410832, 2.944486372867106461, -1.700000000000198019 ) ) ;
#10844=LINE ( 'NONE', #28098, #22549 ) ;
#10847=CARTESIAN_POINT ( 'NONE',  ( -59.69999999999997442, 8.366749974758454467E-15, -2.120534355533670266E-13 ) ) ;
#10848=DIRECTION ( 'NONE',  ( -3.491481338843133355E-15, -3.491481338843133355E-15, 1.000000000000000000 ) ) ;
#10859=CARTESIAN_POINT ( 'NONE',  ( -59.64405989232410832, -2.944486372867071378, -1.700000000000230438 ) ) ;
#10871=ORIENTED_EDGE ( 'NONE', *, *, #864, .F. ) ;
#10873=CARTESIAN_POINT ( 'NONE',  ( -54.49999999999996447, -1.433333333333312254, -4.054078878803088593 ) ) ;
#10891=EDGE_CURVE ( 'NONE', #20368, #13704, #13076, .T. ) ;
#10893=CARTESIAN_POINT ( 'NONE',  ( -56.82202994616205416, -4.156921938165296204, -2.272120436513089232E-13 ) ) ;
#10901=CARTESIAN_POINT ( 'NONE',  ( -59.69999999999997442, 8.366749974758454467E-15, -2.120534355533670266E-13 ) ) ;
#10909=CARTESIAN_POINT ( 'NONE',  ( -60.88452994616204705, 3.117691453623979481, 1.799999999999795985 ) ) ;
#10918=ORIENTED_EDGE ( 'NONE', *, *, #2468, .T. ) ;
#10956=CARTESIAN_POINT ( 'NONE',  ( -56.13452994616205416, -3.117691453623978592, 1.799999999999785771 ) ) ;
#10957=CARTESIAN_POINT ( 'NONE',  ( -59.39405989232410832, 2.944486372867106461, -1.700000000000198019 ) ) ;
#10959=TOROIDAL_SURFACE ( 'NONE', #11458, 0.2000000000000000111, 0.1000000000000000056 ) ;
#10966=CARTESIAN_POINT ( 'NONE',  ( -57.18749999999998579, 1.962990915244722689, 3.399999999999804956 ) ) ;
#10973=CARTESIAN_POINT ( 'NONE',  ( -54.49999999999996447, -1.993349740317589935, -2.907263629733159327 ) ) ;
#10989=CARTESIAN_POINT ( 'NONE',  ( -54.49999999999999289, -3.477081265201396931, 0.03376528397541268128 ) ) ;
#10994=DIRECTION ( 'NONE',  ( 0.000000000000000000, -1.000000000000000000, -3.491481338843133355E-15 ) ) ;
#10996=CARTESIAN_POINT ( 'NONE',  ( -56.93749999999997158, -3.925981830489445379, -2.163561077067149631E-13 ) ) ;
#10999=ORIENTED_EDGE ( 'NONE', *, *, #10891, .F. ) ;
#11000=FACE_OUTER_BOUND ( 'NONE', #3828, .T. ) ;
#11013=EDGE_CURVE ( 'NONE', #14828, #4631, #2237, .T. ) ;
#11021=DIRECTION ( 'NONE',  ( 0.000000000000000000, 0.3333333333333378667, -0.9428090415820618020 ) ) ;
#11031=ORIENTED_EDGE ( 'NONE', *, *, #10059, .F. ) ;
#11032=CARTESIAN_POINT ( 'NONE',  ( -59.51905989232410121, 2.606710529076650314E-14, -3.400000000000210854 ) ) ;
#11040=LINE ( 'NONE', #7869, #2903 ) ;
#11045=VERTEX_POINT ( 'NONE', #3694 ) ;
#11051=DIRECTION ( 'NONE',  ( -1.000000000000000000, 1.219044193948983948E-29, -3.491481338843133355E-15 ) ) ;
#11053=AXIS2_PLACEMENT_3D ( 'NONE', #12200, #19487, #2695 ) ;
#11060=DIRECTION ( 'NONE',  ( 1.000000000000000000, -1.219044193948983948E-29, 3.491481338843133355E-15 ) ) ;
#11073=CARTESIAN_POINT ( 'NONE',  ( -54.49999999999999289, 1.499999999999996003, 3.959797974644419849 ) ) ;
#11078=EDGE_CURVE ( 'NONE', #6036, #17943, #19066, .T. ) ;
#11079=CARTESIAN_POINT ( 'NONE',  ( -54.49999999999996447, -1.993349740317589935, -2.907263629733159327 ) ) ;
#11080=EDGE_CURVE ( 'NONE', #17704, #11119, #2987, .T. ) ;
#11098=PLANE ( 'NONE',  #16530 ) ;
#11099=CARTESIAN_POINT ( 'NONE',  ( -59.19999999999997442, 4.156921938165309527, 1.250136525132554910 ) ) ;
#11107=CARTESIAN_POINT ( 'NONE',  ( -59.19999999999997442, -3.382957286162487698, 0.3399999999999019917 ) ) ;
#11110=( NAMED_UNIT ( * ) SI_UNIT ( $, .STERADIAN. ) SOLID_ANGLE_UNIT ( ) );
#11111=CARTESIAN_POINT ( 'NONE',  ( -55.44702994616206126, -2.078460969082661869, 3.599999999999792255 ) ) ;
#11114=CARTESIAN_POINT ( 'NONE',  ( -59.64405989232410832, -2.944486372867076263, -1.700000000000222222 ) ) ;
#11119=VERTEX_POINT ( 'NONE', #1957 ) ;
#11121=CARTESIAN_POINT ( 'NONE',  ( -55.62499999999998579, -3.920666489018346722E-15, 3.399999999999801403 ) ) ;
#11130=CARTESIAN_POINT ( 'NONE',  ( -59.66583922906154669, 2.374710448338345437, -1.229169263546862734 ) ) ;
#11135=CARTESIAN_POINT ( 'NONE',  ( -54.49999999999997158, -3.430639028629426601, -0.8101486624347474796 ) ) ;
#11136=EDGE_CURVE ( 'NONE', #7227, #11119, #3994, .T. ) ;
#11142=CARTESIAN_POINT ( 'NONE',  ( -57.06249999999997868, -1.962990915244731793, 3.399999999999788969 ) ) ;
#11147=ORIENTED_EDGE ( 'NONE', *, *, #8086, .T. ) ;
#11148=DIRECTION ( 'NONE',  ( 3.491481338843133355E-15, 3.491481338843133355E-15, -1.000000000000000000 ) ) ;
#11155=CARTESIAN_POINT ( 'NONE',  ( -59.41132486540516311, 4.156921938165309527, 1.250136525132554244 ) ) ;
#11164=VECTOR ( 'NONE', #12855, 1000.000000000000000 ) ;
#11166=DIRECTION ( 'NONE',  ( -1.000000000000000000, 1.219044193948983948E-29, -3.491481338843133355E-15 ) ) ;
#11169=CARTESIAN_POINT ( 'NONE',  ( -44.59999999999996589, -1.399999999999979039, -3.959797974644846619 ) ) ;
#11170=CARTESIAN_POINT ( 'NONE',  ( -59.46662241479518229, -2.211912709635374785, 1.464285061855378656 ) ) ;
#11184=LINE ( 'NONE', #15638, #13494 ) ;
#11189=( BOUNDED_CURVE ( )  B_SPLINE_CURVE ( 3, ( #2335, #12002, #21832, #5314 ),
 .UNSPECIFIED., .F., .T. ) 
 B_SPLINE_CURVE_WITH_KNOTS ( ( 4, 4 ),
 ( 0.9419121880553512627, 1.065287454991164173 ),
 .UNSPECIFIED. ) 
 CURVE ( )  GEOMETRIC_REPRESENTATION_ITEM ( )  RATIONAL_B_SPLINE_CURVE ( ( 1.000000000000000000, 0.9987319474856933832, 0.9987319474856933832, 1.000000000000000000 ) ) 
 REPRESENTATION_ITEM ( '' )  );
#11190=VERTEX_POINT ( 'NONE', #7954 ) ;
#11193=CARTESIAN_POINT ( 'NONE',  ( -56.33155989232412963, 3.400000000000008349, -1.856946929144785632E-13 ) ) ;
#11200=DIRECTION ( 'NONE',  ( 0.000000000000000000, -1.000000000000000000, -3.491481338843132961E-15 ) ) ;
#11201=CARTESIAN_POINT ( 'NONE',  ( -58.25952994616203284, -3.117691453623963938, -1.800000000000218092 ) ) ;
#11206=CARTESIAN_POINT ( 'NONE',  ( -55.89405989232412253, -2.944486372867073598, -1.700000000000213563 ) ) ;
#11207=EDGE_CURVE ( 'NONE', #17943, #23827, #23746, .T. ) ;
#11221=CARTESIAN_POINT ( 'NONE',  ( -60.32202994616201863, 2.078460969082674747, -3.600000000000205258 ) ) ;
#11223=VERTEX_POINT ( 'NONE', #22517 ) ;
#11228=DIRECTION ( 'NONE',  ( 3.491481338843133355E-15, 3.491481338843133355E-15, -1.000000000000000000 ) ) ;
#11234=SPHERICAL_SURFACE ( 'NONE', #16475, 0.1000000000000000056 ) ;
#11239=CARTESIAN_POINT ( 'NONE',  ( -44.59999999999998721, -1.400000000000006795, 3.959797974644484242 ) ) ;
#11254=DIRECTION ( 'NONE',  ( -1.000000000000000000, 1.219044193948983948E-29, -3.491481338843133355E-15 ) ) ;
#11261=CARTESIAN_POINT ( 'NONE',  ( -57.70655989232413674, 1.962990915244722245, 3.399999999999802291 ) ) ;
#11265=CARTESIAN_POINT ( 'NONE',  ( -55.87499999999996447, 2.944486372867106905, -1.700000000000186029 ) ) ;
#11267=CARTESIAN_POINT ( 'NONE',  ( -59.69999999999998153, 2.914965204491517081, 1.750136525132549137 ) ) ;
#11270=DIRECTION ( 'NONE',  ( 1.000000000000000000, -1.219044193948983948E-29, 3.491481338843133355E-15 ) ) ;
#11274=DIRECTION ( 'NONE',  ( -1.000000000000000000, 1.219044193948983948E-29, -3.491481338843133355E-15 ) ) ;
#11276=EDGE_CURVE ( 'NONE', #9817, #3419, #19708, .T. ) ;
#11278=CARTESIAN_POINT ( 'NONE',  ( -59.35358983848620795, 2.308634493194285486, 1.301040651491357503 ) ) ;
#11287=CARTESIAN_POINT ( 'NONE',  ( -58.87499999999996447, 2.944486372867106905, -1.700000000000196465 ) ) ;
#11302=CARTESIAN_POINT ( 'NONE',  ( -55.56249999999999289, -1.962990915244736234, 3.399999999999792522 ) ) ;
#11310=DIRECTION ( 'NONE',  ( -1.000000000000000000, -0.000000000000000000, 0.000000000000000000 ) ) ;
#11318=EDGE_CURVE ( 'NONE', #17824, #21074, #23331, .T. ) ;
#11333=DIRECTION ( 'NONE',  ( 0.000000000000000000, 1.000000000000000000, 3.491481338843130594E-15 ) ) ;
#11337=DIRECTION ( 'NONE',  ( 1.000000000000000000, -1.219044193948983948E-29, 3.491481338843133355E-15 ) ) ;
#11345=CARTESIAN_POINT ( 'NONE',  ( -59.32202994616204705, 2.078460969082646770, 3.599999999999797140 ) ) ;
#11347=ADVANCED_FACE ( 'NONE', ( #3810 ), #23155, .T. ) ;
#11352=AXIS2_PLACEMENT_3D ( 'NONE', #8284, #13492, #29972 ) ;
#11353=FACE_OUTER_BOUND ( 'NONE', #13026, .T. ) ;
#11365=CARTESIAN_POINT ( 'NONE',  ( -57.27900635094609072, 3.400000000000004352, 0.9110272542656309147 ) ) ;
#11366=ORIENTED_EDGE ( 'NONE', *, *, #5908, .T. ) ;
#11375=CARTESIAN_POINT ( 'NONE',  ( -60.44702994616202574, -2.078460969082631227, -3.600000000000220801 ) ) ;
#11404=ORIENTED_EDGE ( 'NONE', *, *, #21476, .F. ) ;
#11411=AXIS2_PLACEMENT_3D ( 'NONE', #18310, #16246, #18631 ) ;
#11412=EDGE_LOOP ( 'NONE', ( #27053, #10999, #23287, #21102, #23082 ) ) ;
#11413=VERTEX_POINT ( 'NONE', #25972 ) ;
#11422=EDGE_LOOP ( 'NONE', ( #1057, #19618, #12110, #25052, #17207, #4952, #8003, #26995 ) ) ;
#11423=CARTESIAN_POINT ( 'NONE',  ( -55.50952994616206126, -5.525201388156016014E-15, 3.599999999999801581 ) ) ;
#11424=CARTESIAN_POINT ( 'NONE',  ( -55.89405989232412253, -2.944486372867076263, -1.700000000000208900 ) ) ;
#11432=CARTESIAN_POINT ( 'NONE',  ( -60.68749999999996447, -3.925981830489445379, -2.294491627273766911E-13 ) ) ;
#11434=CARTESIAN_POINT ( 'NONE',  ( -55.17306624327023457, -3.399999999999988365, -0.9110272542660268202 ) ) ;
#11438=DIRECTION ( 'NONE',  ( 0.000000000000000000, 0.3333333333333287629, 0.9428090415820650216 ) ) ;
#11443=DIRECTION ( 'NONE',  ( 0.000000000000000000, -1.000000000000000000, -3.491481338843132961E-15 ) ) ;
#11449=CARTESIAN_POINT ( 'NONE',  ( -59.59999999999998721, 2.022492213459062160, 1.712315755489264513 ) ) ;
#11458=AXIS2_PLACEMENT_3D ( 'NONE', #20920, #9035, #28196 ) ;
#11459=VERTEX_POINT ( 'NONE', #7290 ) ;
#11462=CARTESIAN_POINT ( 'NONE',  ( -55.88452994616203995, 2.093608279459368564E-14, -3.600000000000198597 ) ) ;
#11472=CARTESIAN_POINT ( 'NONE',  ( -59.27103329757905925, -2.428242106091486274, -1.066113908650147879 ) ) ;
#11481=CARTESIAN_POINT ( 'NONE',  ( -55.47099364905386665, -3.399999999999995026, 0.9110272542656059347 ) ) ;
#11482=CARTESIAN_POINT ( 'NONE',  ( -56.18749999999997868, -3.399999999999991029, -2.152687225432237718E-13 ) ) ;
#11488=DIRECTION ( 'NONE',  ( 0.000000000000000000, 1.000000000000000000, 3.491481338843137694E-15 ) ) ;
#11494=CARTESIAN_POINT ( 'NONE',  ( -59.67277382079201686, -2.169063742562021613, 1.523092617832624729 ) ) ;
#11495=CARTESIAN_POINT ( 'NONE',  ( -59.19999999999996732, 4.156921938165317520, -0.9498634748674451567 ) ) ;
#11496=AXIS2_PLACEMENT_3D ( 'NONE', #5042, #22307, #14697 ) ;
#11497=EDGE_CURVE ( 'NONE', #11984, #23827, #14122, .T. ) ;
#11499=TOROIDAL_SURFACE ( 'NONE', #29199, 4.200000000000016165, 0.1000000000000000056 ) ;
#11502=ORIENTED_EDGE ( 'NONE', *, *, #28754, .T. ) ;
#11504=CARTESIAN_POINT ( 'NONE',  ( -59.11126200777224682, -2.334442485522809196, 1.255257642634187043 ) ) ;
#11515=ORIENTED_EDGE ( 'NONE', *, *, #10268, .T. ) ;
#11527=CARTESIAN_POINT ( 'NONE',  ( -59.75952994616203284, -3.117691453623963938, -1.800000000000223199 ) ) ;
#11531=VECTOR ( 'NONE', #24550, 1000.000000000000000 ) ;
#11557=VECTOR ( 'NONE', #21729, 1000.000000000000000 ) ;
#11558=CARTESIAN_POINT ( 'NONE',  ( -55.26905989232413674, -2.944486372867090473, 1.699999999999790345 ) ) ;
#11572=FACE_OUTER_BOUND ( 'NONE', #9224, .T. ) ;
#11583=EDGE_CURVE ( 'NONE', #1670, #24820, #4523, .T. ) ;
#11591=ORIENTED_EDGE ( 'NONE', *, *, #19481, .T. ) ;
#11594=CARTESIAN_POINT ( 'NONE',  ( -60.39405989232410121, -2.944486372867076263, -1.700000000000224665 ) ) ;
#11596=DIRECTION ( 'NONE',  ( 1.000000000000000000, 0.000000000000000000, 0.000000000000000000 ) ) ;
#11600=PRODUCT_DEFINITION_FORMATION_WITH_SPECIFIED_SOURCE ( 'ANY', '', #26984, .NOT_KNOWN. ) ;
#11602=CARTESIAN_POINT ( 'NONE',  ( -59.93749999999996447, -3.925981830489445379, -2.268305517232443506E-13 ) ) ;
#11625=EDGE_CURVE ( 'NONE', #5886, #2222, #1507, .T. ) ;
#11628=CARTESIAN_POINT ( 'NONE',  ( -58.99999999999995737, 2.023778652682509683E-14, -3.400000000000209521 ) ) ;
#11634=CARTESIAN_POINT ( 'NONE',  ( -54.44702994616203995, -2.078460969082631227, -3.600000000000199485 ) ) ;
#11636=CARTESIAN_POINT ( 'NONE',  ( -59.09999999999997300, -2.465712773623968790, -0.9709585562669303949 ) ) ;
#11643=CARTESIAN_POINT ( 'NONE',  ( -55.49999999999997868, -2.944486372867090473, 1.699999999999789679 ) ) ;
#11661=ORIENTED_EDGE ( 'NONE', *, *, #24738, .T. ) ;
#11664=CARTESIAN_POINT ( 'NONE',  ( -54.39999999999996305, 1.500000000000023759, -3.959797974644871044 ) ) ;
#11667=VERTEX_POINT ( 'NONE', #22812 ) ;
#11676=B_SPLINE_CURVE_WITH_KNOTS ( 'NONE', 3,
 ( #10676, #27302, #29091, #3234, #14684, #31312, #17658 ),
 .UNSPECIFIED., .F., .F.,
 ( 4, 3, 4 ),
 ( 0.000000000000000000, 3.134674146556711401E-05, 4.413594575983409879E-05 ),
 .UNSPECIFIED. ) ;
#11680=DIRECTION ( 'NONE',  ( 0.000000000000000000, -4.336808689942024836E-15, 1.000000000000000000 ) ) ;
#11681=CARTESIAN_POINT ( 'NONE',  ( -58.75952994616203284, 3.117691453623994580, -1.800000000000195000 ) ) ;
#11682=CARTESIAN_POINT ( 'NONE',  ( -59.12853372169517741, -2.475303475092485606, -0.9578223113486030726 ) ) ;
#11683=CARTESIAN_POINT ( 'NONE',  ( -59.19999999999997442, -3.317600071788705307, 0.9555264641437645201 ) ) ;
#11704=ORIENTED_EDGE ( 'NONE', *, *, #2967, .F. ) ;
#11709=AXIS2_PLACEMENT_3D ( 'NONE', #22149, #26873, #24491 ) ;
#11729=CIRCLE ( 'NONE', #22356, 0.1000000000000000472 ) ;
#11747=CARTESIAN_POINT ( 'NONE',  ( -61.01905989232410121, 2.023778652682512207E-14, -3.400000000000216183 ) ) ;
#11751=CARTESIAN_POINT ( 'NONE',  ( -59.87499999999995737, -2.944486372867076707, -1.700000000000223332 ) ) ;
#11752=DIRECTION ( 'NONE',  ( 1.000000000000000000, -1.219044193948983948E-29, 3.491481338843133355E-15 ) ) ;
#11755=B_SPLINE_CURVE_WITH_KNOTS ( 'NONE', 3,
 ( #2288, #31273, #23365, #1646 ),
 .UNSPECIFIED., .F., .F.,
 ( 4, 4 ),
 ( 0.000000000000000000, 2.777217045962147943E-05 ),
 .UNSPECIFIED. ) ;
#11776=CARTESIAN_POINT ( 'NONE',  ( -60.99999999999997158, 2.944486372867092250, 1.699999999999795008 ) ) ;
#11782=CARTESIAN_POINT ( 'NONE',  ( -58.00952994616203284, 3.117691453623994580, -1.800000000000192557 ) ) ;
#11788=ORIENTED_EDGE ( 'NONE', *, *, #11078, .T. ) ;
#11794=DIRECTION ( 'NONE',  ( 1.344447539785323523E-44, -1.000000000000000000, -3.491481338843137300E-15 ) ) ;
#11800=CARTESIAN_POINT ( 'NONE',  ( -59.50035777917753421, 3.117067508592329617, 1.404346055332197585 ) ) ;
#11808=ORIENTED_EDGE ( 'NONE', *, *, #21725, .T. ) ;
#11810=VERTEX_POINT ( 'NONE', #16136 ) ;
#11827=CARTESIAN_POINT ( 'NONE',  ( -59.63860681421865451, 2.978809096019410685, 1.643800408120751566 ) ) ;
#11828=CARTESIAN_POINT ( 'NONE',  ( -57.63452994616205416, -3.117691453623976816, 1.799999999999783329 ) ) ;
#11829=LINE ( 'NONE', #18659, #23606 ) ;
#11849=VERTEX_POINT ( 'NONE', #21988 ) ;
#11850=DIRECTION ( 'NONE',  ( -0.000000000000000000, 1.000000000000000000, 3.491481338843133355E-15 ) ) ;
#11877=FACE_OUTER_BOUND ( 'NONE', #23617, .T. ) ;
#11887=AXIS2_PLACEMENT_3D ( 'NONE', #11169, #11310, #8632 ) ;
#11897=CARTESIAN_POINT ( 'NONE',  ( -60.83155989232411542, 3.925981830489463142, -2.015755723410760408E-13 ) ) ;
#11903=CARTESIAN_POINT ( 'NONE',  ( -59.18749999999996447, -3.925981830489445379, -2.242119407191119848E-13 ) ) ;
#11908=AXIS2_PLACEMENT_3D ( 'NONE', #18084, #1264, #3798 ) ;
#11914=CARTESIAN_POINT ( 'NONE',  ( -58.43749999999997158, -3.399999999999991029, -2.253785087031484148E-13 ) ) ;
#11923=DIRECTION ( 'NONE',  ( 1.000000000000000000, -1.219044193948983948E-29, 3.491481338843133355E-15 ) ) ;
#11929=CARTESIAN_POINT ( 'NONE',  ( -55.63452994616205416, 3.117691453623979481, 1.799999999999814415 ) ) ;
#11938=CARTESIAN_POINT ( 'NONE',  ( -58.44702994616205416, -2.078460969082657872, 3.599999999999784261 ) ) ;
#11954=CARTESIAN_POINT ( 'NONE',  ( -44.59999999999998010, 8.366749974758271452E-15, -1.593320673368357319E-13 ) ) ;
#11982=CARTESIAN_POINT ( 'NONE',  ( -54.39999999999999147, -1.400000000000006795, 3.959797974644448715 ) ) ;
#11984=VERTEX_POINT ( 'NONE', #30021 ) ;
#11986=CARTESIAN_POINT ( 'NONE',  ( -59.36488781976483864, 2.508594352967818963, -1.045061501994789976 ) ) ;
#11993=CARTESIAN_POINT ( 'NONE',  ( -60.75952994616205416, -4.643455692769856999E-15, 3.599999999999783373 ) ) ;
#11994=CARTESIAN_POINT ( 'NONE',  ( -59.16607095580928899, -2.501426125405462386, -0.9458072644521190453 ) ) ;
#11995=VECTOR ( 'NONE', #30029, 1000.000000000000000 ) ;
#12002=CARTESIAN_POINT ( 'NONE',  ( -59.52807307762599720, -2.290451074298654799, 1.439549604813781913 ) ) ;
#12012=ORIENTED_EDGE ( 'NONE', *, *, #10268, .F. ) ;
#12021=DIRECTION ( 'NONE',  ( -1.510019896901732094E-45, -1.000000000000000000, -3.491481338843132566E-15 ) ) ;
#12030=CARTESIAN_POINT ( 'NONE',  ( -44.49999999999996447, 1.500000000000021538, -3.363870538531645416 ) ) ;
#12031=CARTESIAN_POINT ( 'NONE',  ( -44.59999999999996589, 1.400000000000023670, -3.959797974644836405 ) ) ;
#12032=CARTESIAN_POINT ( 'NONE',  ( -57.87499999999997868, -1.933093229062082319E-14, 3.399999999999793854 ) ) ;
#12035=VERTEX_POINT ( 'NONE', #13379 ) ;
#12039=AXIS2_PLACEMENT_3D ( 'NONE', #16904, #28783, #28463 ) ;
#12042=DIRECTION ( 'NONE',  ( -1.000000000000000000, -0.000000000000000000, 0.000000000000000000 ) ) ;
#12043=FACE_OUTER_BOUND ( 'NONE', #4494, .T. ) ;
#12051=CARTESIAN_POINT ( 'NONE',  ( -44.49999999999998579, 2.395752775956332847, 1.350136525132600296 ) ) ;
#12053=CARTESIAN_POINT ( 'NONE',  ( -59.69999999999997442, -3.399999999999991473, -2.235080921937235780E-13 ) ) ;
#12061=ADVANCED_FACE ( 'NONE', ( #30186 ), #10716, .T. ) ;
#12074=CARTESIAN_POINT ( 'NONE',  ( -55.50952994616206126, -4.643455692769921685E-15, 3.599999999999801581 ) ) ;
#12079=CARTESIAN_POINT ( 'NONE',  ( -54.39999999999996305, -1.399999999999979039, -3.959797974644881258 ) ) ;
#12081=VECTOR ( 'NONE', #7282, 1000.000000000000000 ) ;
#12096=EDGE_CURVE ( 'NONE', #3236, #19668, #22918, .T. ) ;
#12098=CYLINDRICAL_SURFACE ( 'NONE', #30991, 3.625000000000024869 ) ;
#12099=CARTESIAN_POINT ( 'NONE',  ( -57.44702994616203284, -2.078460969082631227, -3.600000000000210587 ) ) ;
#12102=CARTESIAN_POINT ( 'NONE',  ( -59.54613710108586844, 3.305219929794498857, -1.149705823355897438 ) ) ;
#12105=CARTESIAN_POINT ( 'NONE',  ( -55.44702994616206126, -2.078460969082657872, 3.599999999999794920 ) ) ;
#12106=ORIENTED_EDGE ( 'NONE', *, *, #19645, .F. ) ;
#12109=DIRECTION ( 'NONE',  ( -7.637891338979715149E-45, -1.000000000000000000, -3.491481338843131383E-15 ) ) ;
#12110=ORIENTED_EDGE ( 'NONE', *, *, #16640, .T. ) ;
#12111=CARTESIAN_POINT ( 'NONE',  ( -44.59999999999996589, -1.399999999999981037, -3.363870538531656962 ) ) ;
#12137=CARTESIAN_POINT ( 'NONE',  ( -59.19999999999997442, 8.366749974758448157E-15, -2.103076948839454410E-13 ) ) ;
#12147=CARTESIAN_POINT ( 'NONE',  ( -59.69999999999998153, 2.914965204491517081, 1.750136525132549137 ) ) ;
#12148=CARTESIAN_POINT ( 'NONE',  ( -56.76905989232412963, -2.944486372867088697, 1.699999999999787015 ) ) ;
#12166=SURFACE_STYLE_USAGE ( .BOTH. , #10099 ) ;
#12170=EDGE_LOOP ( 'NONE', ( #9838, #28355, #17056, #25535, #6592, #24312, #21279 ) ) ;
#12171=CARTESIAN_POINT ( 'NONE',  ( -44.59999999999997300, 8.366749974758367693E-15, -1.870876429524646202E-13 ) ) ;
#12179=CARTESIAN_POINT ( 'NONE',  ( -55.37499999999996447, -2.944486372867075819, -1.700000000000208455 ) ) ;
#12180=FACE_OUTER_BOUND ( 'NONE', #12415, .T. ) ;
#12182=( BOUNDED_SURFACE ( )  B_SPLINE_SURFACE ( 1, 2, ( 
 ( #3218, #14633, #12859, #846, #29818, #2609, #12254, #21939, #222, #9884, #25689, #5751, #20341, #23177, #8588, #1461, #1299, #27757, #11121, #13317, #29968, #15868, #11265, #8276, #20798, #27907, #30278, #30112, #18267, #8887, #15575, #1151, #6075, #13639, #6218, #30427, #16031, #8728, #18415, #10662, #5916, #15401, #1607, #10966, #22864, #27589, #25375, #3678, #25223, #25520, #27438, #3833, #28053, #3541, #13482, #6369, #3995, #23321, #20651, #20946, #17944, #25054, #13177, #30578, #20487, #3384, #13031, #10803, #22715, #23008, #1010, #8434, #18118, #15726, #21283, #11903, #1761, #14123, #30911, #18886, #4619, #2087, #23797, #30756, #40, #21122, #11751, #11602, #23944, #24100, #9065, #31230, #16505, #21425, #9228, #26162, #28703, #28530, #21587, #11432, #31056, #6840, #4469, #2411, #9379, #19048, #18738, #28378, #23643 ),
 ( #19214, #2238, #14279, #9556, #6683, #28855, #7014, #14427, #7168, #6533, #21751, #16678, #13784, #26321, #16830, #26468, #4768, #16345, #12074, #18578, #28225, #16194, #25841, #4148, #25992, #23468, #4298, #13946, #1940, #15211, #24857, #9702, #29160, #29002, #17428, #19968, #19365, #29604, #14743, #7312, #10010, #19673, #29313, #12356, #5398, #16980, #22042, #3175, #7931, #26630, #2573, #15057, #22203, #24712, #14886, #7624, #3024, #26926, #12218, #29450, #12815, #21901, #12668, #10152, #12520, #339, #492, #22499, #7476, #24403, #17283, #27245, #19818, #22349, #17600, #640, #10299, #24261, #19512, #4937, #14595, #24549, #5093, #9843, #5234, #2868, #17142, #7763, #185, #27078, #5562, #26789, #2712, #6184, #3643, #3499, #27868, #10464, #13139, #25645, #30389, #20146, #25009, #15829, #13279, #25482, #6037, #1116, #3791 ) ),
 .UNSPECIFIED., .F., .F., .T. ) 
 B_SPLINE_SURFACE_WITH_KNOTS ( ( 2, 2 ),
 ( 3, 2, 2, 2, 2, 2, 2, 2, 2, 2, 2, 2, 2, 2, 2, 2, 2, 2, 2, 2, 2, 2, 2, 2, 2, 2, 2, 2, 2, 2, 2, 2, 2, 2, 2, 2, 2, 2, 2, 2, 2, 2, 2, 2, 2, 2, 2, 2, 2, 2, 2, 2, 2, 2, 3 ),
 ( 0.000000000000000000, 1.000000000000000000 ),
 ( 0.000000000000000000, 0.01851851851851851749, 0.03703703703703703498, 0.05555555555555555247, 0.07407407407407406996, 0.09259259259259258745, 0.1111111111111111049, 0.1296296296296296224, 0.1481481481481481399, 0.1666666666666666574, 0.1851851851851851749, 0.2037037037037036924, 0.2222222222222222099, 0.2407407407407407274, 0.2592592592592592449, 0.2777777777777777901, 0.2962962962962962798, 0.3148148148148148251, 0.3333333333333333148, 0.3518518518518518601, 0.3703703703703703498, 0.3888888888888888951, 0.4074074074074073848, 0.4259259259259259300, 0.4444444444444444198, 0.4629629629629629650, 0.4814814814814814548, 0.5000000000000000000, 0.5185185185185184897, 0.5370370370370370905, 0.5555555555555555802, 0.5740740740740740700, 0.5925925925925925597, 0.6111111111111111605, 0.6296296296296296502, 0.6481481481481481399, 0.6666666666666666297, 0.6851851851851852304, 0.7037037037037037202, 0.7222222222222222099, 0.7407407407407406996, 0.7592592592592593004, 0.7777777777777777901, 0.7962962962962962798, 0.8148148148148147696, 0.8333333333333333703, 0.8518518518518518601, 0.8703703703703703498, 0.8888888888888888395, 0.9074074074074074403, 0.9259259259259259300, 0.9444444444444444198, 0.9629629629629629095, 0.9814814814814815103, 1.000000000000000000 ),
 .UNSPECIFIED. ) 
 GEOMETRIC_REPRESENTATION_ITEM ( )  RATIONAL_B_SPLINE_SURFACE ( (
 ( 1.000000000000000000, 0.8660254037844387076, 1.000000000000000000, 0.8660254037844387076, 1.000000000000000000, 0.8660254037844387076, 1.000000000000000000, 0.8660254037844387076, 1.000000000000000000, 0.8660254037844387076, 1.000000000000000000, 0.8660254037844387076, 1.000000000000000000, 0.8660254037844387076, 1.000000000000000000, 0.8660254037844387076, 1.000000000000000000, 0.8660254037844387076, 1.000000000000000000, 0.8660254037844387076, 1.000000000000000000, 0.8660254037844387076, 1.000000000000000000, 0.8660254037844387076, 1.000000000000000000, 0.8660254037844387076, 1.000000000000000000, 0.8660254037844387076, 1.000000000000000000, 0.8660254037844387076, 1.000000000000000000, 0.8660254037844387076, 1.000000000000000000, 0.8660254037844387076, 1.000000000000000000, 0.8660254037844387076, 1.000000000000000000, 0.8660254037844387076, 1.000000000000000000, 0.8660254037844387076, 1.000000000000000000, 0.8660254037844387076, 1.000000000000000000, 0.8660254037844387076, 1.000000000000000000, 0.8660254037844387076, 1.000000000000000000, 0.8660254037844387076, 1.000000000000000000, 0.8660254037844387076, 1.000000000000000000, 0.8660254037844387076, 1.000000000000000000, 0.8660254037844387076, 1.000000000000000000, 0.8660254037844387076, 1.000000000000000000, 0.8660254037844387076, 1.000000000000000000, 0.8660254037844387076, 1.000000000000000000, 0.8660254037844387076, 1.000000000000000000, 0.8660254037844387076, 1.000000000000000000, 0.8660254037844387076, 1.000000000000000000, 0.8660254037844387076, 1.000000000000000000, 0.8660254037844387076, 1.000000000000000000, 0.8660254037844387076, 1.000000000000000000, 0.8660254037844387076, 1.000000000000000000, 0.8660254037844387076, 1.000000000000000000, 0.8660254037844387076, 1.000000000000000000, 0.8660254037844387076, 1.000000000000000000, 0.8660254037844387076, 1.000000000000000000, 0.8660254037844387076, 1.000000000000000000, 0.8660254037844387076, 1.000000000000000000, 0.8660254037844387076, 1.000000000000000000, 0.8660254037844387076, 1.000000000000000000, 0.8660254037844387076, 1.000000000000000000, 0.8660254037844387076, 1.000000000000000000, 0.8660254037844387076, 1.000000000000000000, 0.8660254037844387076, 1.000000000000000000, 0.8660254037844387076, 1.000000000000000000, 0.8660254037844387076, 1.000000000000000000, 0.8660254037844387076, 1.000000000000000000, 0.8660254037844387076, 1.000000000000000000, 0.8660254037844387076, 1.000000000000000000),
 ( 1.000000000000000000, 0.8660254037844387076, 1.000000000000000000, 0.8660254037844387076, 1.000000000000000000, 0.8660254037844387076, 1.000000000000000000, 0.8660254037844387076, 1.000000000000000000, 0.8660254037844387076, 1.000000000000000000, 0.8660254037844387076, 1.000000000000000000, 0.8660254037844387076, 1.000000000000000000, 0.8660254037844387076, 1.000000000000000000, 0.8660254037844387076, 1.000000000000000000, 0.8660254037844387076, 1.000000000000000000, 0.8660254037844387076, 1.000000000000000000, 0.8660254037844387076, 1.000000000000000000, 0.8660254037844387076, 1.000000000000000000, 0.8660254037844387076, 1.000000000000000000, 0.8660254037844387076, 1.000000000000000000, 0.8660254037844387076, 1.000000000000000000, 0.8660254037844387076, 1.000000000000000000, 0.8660254037844387076, 1.000000000000000000, 0.8660254037844387076, 1.000000000000000000, 0.8660254037844387076, 1.000000000000000000, 0.8660254037844387076, 1.000000000000000000, 0.8660254037844387076, 1.000000000000000000, 0.8660254037844387076, 1.000000000000000000, 0.8660254037844387076, 1.000000000000000000, 0.8660254037844387076, 1.000000000000000000, 0.8660254037844387076, 1.000000000000000000, 0.8660254037844387076, 1.000000000000000000, 0.8660254037844387076, 1.000000000000000000, 0.8660254037844387076, 1.000000000000000000, 0.8660254037844387076, 1.000000000000000000, 0.8660254037844387076, 1.000000000000000000, 0.8660254037844387076, 1.000000000000000000, 0.8660254037844387076, 1.000000000000000000, 0.8660254037844387076, 1.000000000000000000, 0.8660254037844387076, 1.000000000000000000, 0.8660254037844387076, 1.000000000000000000, 0.8660254037844387076, 1.000000000000000000, 0.8660254037844387076, 1.000000000000000000, 0.8660254037844387076, 1.000000000000000000, 0.8660254037844387076, 1.000000000000000000, 0.8660254037844387076, 1.000000000000000000, 0.8660254037844387076, 1.000000000000000000, 0.8660254037844387076, 1.000000000000000000, 0.8660254037844387076, 1.000000000000000000, 0.8660254037844387076, 1.000000000000000000, 0.8660254037844387076, 1.000000000000000000, 0.8660254037844387076, 1.000000000000000000, 0.8660254037844387076, 1.000000000000000000, 0.8660254037844387076, 1.000000000000000000, 0.8660254037844387076, 1.000000000000000000, 0.8660254037844387076, 1.000000000000000000, 0.8660254037844387076, 1.000000000000000000, 0.8660254037844387076, 1.000000000000000000, 0.8660254037844387076, 1.000000000000000000) ) ) 
 REPRESENTATION_ITEM ( '' )  SURFACE ( )  );
#12192=CARTESIAN_POINT ( 'NONE',  ( -59.46761860684633660, 2.377675374897951333, -1.175485268738917677 ) ) ;
#12200=CARTESIAN_POINT ( 'NONE',  ( -59.19999999999996732, 4.156921938165317520, -0.9498634748674451567 ) ) ;
#12216=( BOUNDED_CURVE ( )  B_SPLINE_CURVE ( 2, ( #17878, #3305, #3620, #12952, #13111, #22647, #7893, #25308, #19940 ),
 .UNSPECIFIED., .F., .T. ) 
 B_SPLINE_CURVE_WITH_KNOTS ( ( 3, 2, 2, 2, 3 ),
 ( 0.5833333333333333703, 0.5925925925925925597, 0.6111111111111111605, 0.6296296296296296502, 0.6388888888888889506 ),
 .UNSPECIFIED. ) 
 CURVE ( )  GEOMETRIC_REPRESENTATION_ITEM ( )  RATIONAL_B_SPLINE_CURVE ( ( 0.9330127018922194093, 0.9330127018922197424, 1.000000000000000000, 0.8660254037844387076, 1.000000000000000000, 0.8660254037844387076, 1.000000000000000000, 0.9330127018922189652, 0.9330127018922194093 ) ) 
 REPRESENTATION_ITEM ( '' )  );
#12218=CARTESIAN_POINT ( 'NONE',  ( -58.00952994616203284, 3.117691453623994580, -1.800000000000192557 ) ) ;
#12234=CARTESIAN_POINT ( 'NONE',  ( -59.09999999999997300, 8.366749974758448157E-15, -2.099585467500611340E-13 ) ) ;
#12240=ADVANCED_FACE ( 'NONE', ( #26380 ), #24620, .T. ) ;
#12248=CARTESIAN_POINT ( 'NONE',  ( -55.13452994616203995, 2.093608279459367933E-14, -3.600000000000195932 ) ) ;
#12253=ORIENTED_EDGE ( 'NONE', *, *, #3910, .F. ) ;
#12254=CARTESIAN_POINT ( 'NONE',  ( -54.87499999999998579, -3.920666489018356189E-15, 3.399999999999804068 ) ) ;
#12267=ORIENTED_EDGE ( 'NONE', *, *, #22720, .F. ) ;
#12283=CARTESIAN_POINT ( 'NONE',  ( -55.64405989232412253, 2.944486372867106461, -1.700000000000184919 ) ) ;
#12298=LINE ( 'NONE', #16438, #30500 ) ;
#12300=FILL_AREA_STYLE_COLOUR ( '', #6642 ) ;
#12312=CARTESIAN_POINT ( 'NONE',  ( -55.99999999999995737, 2.190330617366546392E-14, -3.400000000000199307 ) ) ;
#12314=CARTESIAN_POINT ( 'NONE',  ( -55.40400635094609072, -3.399999999999988365, -0.9110272542660277084 ) ) ;
#12318=ORIENTED_EDGE ( 'NONE', *, *, #3336, .T. ) ;
#12322=ADVANCED_BREP_SHAPE_REPRESENTATION ( '', ( #4756, #9018 ), #5016 ) ;
#12324=ADVANCED_FACE ( 'NONE', ( #15599 ), #2652, .T. ) ;
#12333=ORIENTED_EDGE ( 'NONE', *, *, #5560, .T. ) ;
#12356=CARTESIAN_POINT ( 'NONE',  ( -57.07202994616206126, 2.078460969082646770, 3.599999999999804690 ) ) ;
#12361=CARTESIAN_POINT ( 'NONE',  ( -57.04806624327023457, 3.400000000000003908, 0.9110272542656316919 ) ) ;
#12378=ORIENTED_EDGE ( 'NONE', *, *, #29511, .T. ) ;
#12383=ORIENTED_EDGE ( 'NONE', *, *, #25413, .T. ) ;
#12390=CARTESIAN_POINT ( 'NONE',  ( -55.75952994616203995, 3.117691453623994580, -1.800000000000184563 ) ) ;
#12391=ORIENTED_EDGE ( 'NONE', *, *, #23328, .T. ) ;
#12405=CIRCLE ( 'NONE', #30098, 0.1000000000000000472 ) ;
#12411=ORIENTED_EDGE ( 'NONE', *, *, #5588, .F. ) ;
#12415=EDGE_LOOP ( 'NONE', ( #21350, #14955, #21685, #17818 ) ) ;
#12421=AXIS2_PLACEMENT_3D ( 'NONE', #22010, #12484, #17114 ) ;
#12422=ORIENTED_EDGE ( 'NONE', *, *, #21476, .T. ) ;
#12427=CARTESIAN_POINT ( 'NONE',  ( -58.81249999999996447, 3.400000000000008349, -1.915049148454697437E-13 ) ) ;
#12436=CARTESIAN_POINT ( 'NONE',  ( -55.51905989232413674, 2.944486372867092250, 1.699999999999814104 ) ) ;
#12438=AXIS2_PLACEMENT_3D ( 'NONE', #29941, #3513, #13152 ) ;
#12441=CARTESIAN_POINT ( 'NONE',  ( -58.49999999999997868, -2.944486372867095358, 1.699999999999771028 ) ) ;
#12453=ORIENTED_EDGE ( 'NONE', *, *, #18350, .F. ) ;
#12456=PRESENTATION_STYLE_ASSIGNMENT (( #12166 ) ) ;
#12459=ORIENTED_EDGE ( 'NONE', *, *, #2601, .F. ) ;
#12461=CARTESIAN_POINT ( 'NONE',  ( -57.64405989232413674, -1.933093229062082635E-14, 3.399999999999794298 ) ) ;
#12476=CIRCLE ( 'NONE', #27150, 3.399999999999999911 ) ;
#12484=DIRECTION ( 'NONE',  ( 1.000000000000000000, -1.219044193948983948E-29, 3.491481338843133355E-15 ) ) ;
#12486=PLANE ( 'NONE',  #5341 ) ;
#12491=ORIENTED_EDGE ( 'NONE', *, *, #11583, .F. ) ;
#12496=CARTESIAN_POINT ( 'NONE',  ( -59.69999999999997442, 8.366749974758454467E-15, -2.120534355533670266E-13 ) ) ;
#12497=CARTESIAN_POINT ( 'NONE',  ( -54.46614378277664059, -2.255560380866761250, -2.805788190199900889 ) ) ;
#12498=CARTESIAN_POINT ( 'NONE',  ( -44.59999999999996589, -1.399999999999979261, -3.959797974644847507 ) ) ;
#12520=CARTESIAN_POINT ( 'NONE',  ( -58.38452994616204705, -3.117691453623976816, 1.799999999999780442 ) ) ;
#12550=CARTESIAN_POINT ( 'NONE',  ( -59.88452994616203995, -3.117691453623976816, 1.799999999999775335 ) ) ;
#12567=EDGE_CURVE ( 'NONE', #20708, #25749, #1817, .T. ) ;
#12571=EDGE_CURVE ( 'NONE', #13230, #6307, #29442, .T. ) ;
#12576=ORIENTED_EDGE ( 'NONE', *, *, #29439, .F. ) ;
#12577=CARTESIAN_POINT ( 'NONE',  ( -59.16647130186552772, 2.362152846858203592, 1.255950301266114622 ) ) ;
#12591=CARTESIAN_POINT ( 'NONE',  ( -57.11505354137801049, 3.400000000000011902, -0.9110272542660005080 ) ) ;
#12594=ORIENTED_EDGE ( 'NONE', *, *, #331, .F. ) ;
#12596=CARTESIAN_POINT ( 'NONE',  ( -60.00952994616204705, -4.643455692769866465E-15, 3.599999999999786038 ) ) ;
#12604=ADVANCED_FACE ( 'NONE', ( #5550 ), #27065, .T. ) ;
#12641=CARTESIAN_POINT ( 'NONE',  ( -58.00952994616203284, 3.117691453623999021, -1.800000000000183897 ) ) ;
#12658=CARTESIAN_POINT ( 'NONE',  ( -58.32202994616204705, -4.156921938165296204, -2.220106322563329850E-13 ) ) ;
#12666=ORIENTED_EDGE ( 'NONE', *, *, #18779, .F. ) ;
#12668=CARTESIAN_POINT ( 'NONE',  ( -58.25952994616203284, -3.117691453623963938, -1.800000000000218092 ) ) ;
#12669=CARTESIAN_POINT ( 'NONE',  ( -59.69999999999997442, 3.400000000000007905, -2.001823990013003858E-13 ) ) ;
#12673=CARTESIAN_POINT ( 'NONE',  ( -57.08155989232412963, 3.400000000000007905, -1.873796572744660248E-13 ) ) ;
#12694=ORIENTED_EDGE ( 'NONE', *, *, #5356, .T. ) ;
#12701=CARTESIAN_POINT ( 'NONE',  ( -60.94702994616203995, 4.156921938165313080, -2.011299877933566609E-13 ) ) ;
#12706=EDGE_CURVE ( 'NONE', #28363, #4064, #30232, .T. ) ;
#12708=ORIENTED_EDGE ( 'NONE', *, *, #27206, .F. ) ;
#12727=CARTESIAN_POINT ( 'NONE',  ( -59.69999999999997442, -3.399999999999991473, -2.235080921937235780E-13 ) ) ;
#12729=CIRCLE ( 'NONE', #2119, 0.1000000000000000472 ) ;
#12743=CARTESIAN_POINT ( 'NONE',  ( -58.81249999999996447, 3.400000000000008349, -1.915049148454697437E-13 ) ) ;
#12749=CARTESIAN_POINT ( 'NONE',  ( -58.33155989232413674, -1.962990915244731571, 3.399999999999784528 ) ) ;
#12764=CARTESIAN_POINT ( 'NONE',  ( -59.19999999999996732, -2.569786949633424022, -0.9498634748674686934 ) ) ;
#12773=CARTESIAN_POINT ( 'NONE',  ( -58.20655989232411542, -3.399999999999991029, -2.246812820714294660E-13 ) ) ;
#12778=CARTESIAN_POINT ( 'NONE',  ( -55.87499999999996447, 2.944486372867106905, -1.700000000000185363 ) ) ;
#12780=CARTESIAN_POINT ( 'NONE',  ( -54.79806624327024167, 3.400000000000004796, 0.9110272542656339123 ) ) ;
#12782=CARTESIAN_POINT ( 'NONE',  ( -59.59999999999997300, 2.337126060168390307, -1.249136413240100607 ) ) ;
#12784=CARTESIAN_POINT ( 'NONE',  ( -54.94702994616205416, 4.156921938165313080, -1.801810997602979365E-13 ) ) ;
#12789=EDGE_CURVE ( 'NONE', #3419, #3612, #29663, .T. ) ;
#12791=CARTESIAN_POINT ( 'NONE',  ( -57.69702994616205416, -2.078460969082671195, 3.599999999999778932 ) ) ;
#12807=CARTESIAN_POINT ( 'NONE',  ( -58.38452994616204705, -3.117691453623976816, 1.799999999999780442 ) ) ;
#12815=CARTESIAN_POINT ( 'NONE',  ( -58.13452994616202574, 2.093608279459371404E-14, -3.600000000000206146 ) ) ;
#12817=CARTESIAN_POINT ( 'NONE',  ( -56.51905989232411542, 2.273606599708566482E-14, -3.400000000000200640 ) ) ;
#12828=CARTESIAN_POINT ( 'NONE',  ( -59.31249999999997868, -1.962990915244734236, 3.399999999999780975 ) ) ;
#12831=( BOUNDED_CURVE ( )  B_SPLINE_CURVE ( 2, ( #17160, #15232, #3046, #29331, #29020, #14764, #22225, #24569, #17620 ),
 .UNSPECIFIED., .F., .T. ) 
 B_SPLINE_CURVE_WITH_KNOTS ( ( 3, 2, 2, 2, 3 ),
 ( 0.5277777777777777901, 0.5370370370370370905, 0.5555555555555555802, 0.5740740740740740700, 0.5833333333333333703 ),
 .UNSPECIFIED. ) 
 CURVE ( )  GEOMETRIC_REPRESENTATION_ITEM ( )  RATIONAL_B_SPLINE_CURVE ( ( 0.9330127018922194093, 0.9330127018922194093, 1.000000000000000000, 0.8660254037844387076, 1.000000000000000000, 0.8660254037844387076, 1.000000000000000000, 0.9330127018922189652, 0.9330127018922194093 ) ) 
 REPRESENTATION_ITEM ( '' )  );
#12850=CARTESIAN_POINT ( 'NONE',  ( -55.51905989232413674, 2.944486372867092250, 1.699999999999814104 ) ) ;
#12851=VERTEX_POINT ( 'NONE', #2041 ) ;
#12852=DIRECTION ( 'NONE',  ( 1.344447539785323523E-44, -1.000000000000000000, -3.491481338843137300E-15 ) ) ;
#12855=DIRECTION ( 'NONE',  ( 3.491481338843133355E-15, 3.491481338843133355E-15, -1.000000000000000000 ) ) ;
#12859=CARTESIAN_POINT ( 'NONE',  ( -54.62499999999997158, -2.944486372867076707, -1.700000000000204903 ) ) ;
#12866=EDGE_CURVE ( 'NONE', #29758, #8534, #9505, .T. ) ;
#12881=CARTESIAN_POINT ( 'NONE',  ( -58.43749999999997158, -3.925981830489445379, -2.215933297149796442E-13 ) ) ;
#12893=AXIS2_PLACEMENT_3D ( 'NONE', #24135, #18764, #6871 ) ;
#12894=CARTESIAN_POINT ( 'NONE',  ( -54.39999999999999147, 1.399999999999998135, 3.363870538531246623 ) ) ;
#12896=CARTESIAN_POINT ( 'NONE',  ( -58.99999999999995737, 2.523434546734630224E-14, -3.400000000000209521 ) ) ;
#12899=CARTESIAN_POINT ( 'NONE',  ( -60.95655989232410121, 1.962990915244748891, -3.400000000000207301 ) ) ;
#12901=DIRECTION ( 'NONE',  ( -1.000000000000000000, 1.219044193948983948E-29, -3.491481338843133355E-15 ) ) ;
#12917=AXIS2_PLACEMENT_3D ( 'NONE', #7804, #682, #15098 ) ;
#12922=EDGE_CURVE ( 'NONE', #18983, #23830, #20354, .T. ) ;
#12937=ADVANCED_FACE ( 'NONE', ( #7720 ), #25665, .T. ) ;
#12943=CARTESIAN_POINT ( 'NONE',  ( -59.69999999999996732, 1.144555898245933179, -3.233327234211546219 ) ) ;
#12952=CARTESIAN_POINT ( 'NONE',  ( -58.33155989232412963, -1.962990915244733348, 3.399999999999783640 ) ) ;
#12956=CARTESIAN_POINT ( 'NONE',  ( -57.50952994616203995, -3.117691453623959941, -1.800000000000221645 ) ) ;
#12958=CARTESIAN_POINT ( 'NONE',  ( -54.49999999999999289, 1.599999999999998090, 3.363870538531247067 ) ) ;
#12965=CARTESIAN_POINT ( 'NONE',  ( -59.09999999999997300, 2.465712773623992327, -0.9709585562669131864 ) ) ;
#12969=VERTEX_POINT ( 'NONE', #21855 ) ;
#12975=CARTESIAN_POINT ( 'NONE',  ( -57.38452994616203284, 2.093608279459370457E-14, -3.600000000000203926 ) ) ;
#12979=CARTESIAN_POINT ( 'NONE',  ( -54.49999999999996447, -1.514093959731525496, -3.183260039818593512 ) ) ;
#12987=DIRECTION ( 'NONE',  ( -1.000000000000000000, 1.219044193948983948E-29, -3.491481338843133355E-15 ) ) ;
#12996=CARTESIAN_POINT ( 'NONE',  ( -56.93749999999996447, -3.399999999999991473, -2.119568960425587465E-13 ) ) ;
#12998=AXIS2_PLACEMENT_3D ( 'NONE', #12079, #16510, #11438 ) ;
#13002=CARTESIAN_POINT ( 'NONE',  ( -59.66355212511316353, 2.047887940248842575, 1.716336187188254314 ) ) ;
#13018=CARTESIAN_POINT ( 'NONE',  ( -54.39999999999997726, 3.624999999999963585, -1.915392816594897935E-13 ) ) ;
#13025=CARTESIAN_POINT ( 'NONE',  ( -54.45655989232412963, -3.925981830489445379, -2.076939516179772989E-13 ) ) ;
#13026=EDGE_LOOP ( 'NONE', ( #1233, #18454, #23864, #26846 ) ) ;
#13031=CARTESIAN_POINT ( 'NONE',  ( -58.62499999999998579, -3.920666489018310435E-15, 3.399999999999791189 ) ) ;
#13034=DIRECTION ( 'NONE',  ( -1.000000000000000000, 1.219044193948983948E-29, -3.491481338843133355E-15 ) ) ;
#13042=CARTESIAN_POINT ( 'NONE',  ( -59.67318048135356179, 2.383480368854711262, -1.229362881338640801 ) ) ;
#13044=EDGE_CURVE ( 'NONE', #23827, #14659, #8655, .T. ) ;
#13047=ORIENTED_EDGE ( 'NONE', *, *, #22720, .T. ) ;
#13050=ORIENTED_EDGE ( 'NONE', *, *, #30024, .F. ) ;
#13051=DIRECTION ( 'NONE',  ( 1.000000000000000000, -1.219044193948983948E-29, 3.491481338843133355E-15 ) ) ;
#13053=CARTESIAN_POINT ( 'NONE',  ( -56.74999999999995737, 2.023778652682507474E-14, -3.400000000000201972 ) ) ;
#13056=ORIENTED_EDGE ( 'NONE', *, *, #3790, .T. ) ;
#13057=ORIENTED_EDGE ( 'NONE', *, *, #10812, .T. ) ;
#13066=CARTESIAN_POINT ( 'NONE',  ( -60.01905989232411542, 2.944486372867092250, 1.699999999999798339 ) ) ;
#13073=FACE_OUTER_BOUND ( 'NONE', #6485, .T. ) ;
#13076=CIRCLE ( 'NONE', #14601, 2.649999999999999911 ) ;
#13081=ADVANCED_FACE ( 'NONE', ( #25292 ), #20721, .T. ) ;
#13090=ORIENTED_EDGE ( 'NONE', *, *, #9527, .F. ) ;
#13106=ORIENTED_EDGE ( 'NONE', *, *, #8280, .T. ) ;
#13111=CARTESIAN_POINT ( 'NONE',  ( -58.39405989232412963, -2.016369211404101147E-14, 3.399999999999791633 ) ) ;
#13114=CARTESIAN_POINT ( 'NONE',  ( -57.94702994616203995, 4.156921938165313968, -1.791987581444107632E-13 ) ) ;
#13122=CARTESIAN_POINT ( 'NONE',  ( -59.19174289917960863, 2.538702292234776170, -0.9450962354860914516 ) ) ;
#13129=CARTESIAN_POINT ( 'NONE',  ( -56.07202994616204705, -4.156921938165296204, -2.141547992439359634E-13 ) ) ;
#13139=CARTESIAN_POINT ( 'NONE',  ( -60.50952994616203284, -3.117691453623963938, -1.800000000000225864 ) ) ;
#13142=CARTESIAN_POINT ( 'NONE',  ( -56.67306624327023457, -3.399999999999988365, -0.9110272542660329265 ) ) ;
#13152=DIRECTION ( 'NONE',  ( 0.000000000000000000, -1.000000000000000000, -4.336808689942015369E-15 ) ) ;
#13166=CYLINDRICAL_SURFACE ( 'NONE', #17513, 3.399999999999999911 ) ;
#13171=CARTESIAN_POINT ( 'NONE',  ( -60.69702994616205416, -2.078460969082657872, 3.599999999999776712 ) ) ;
#13177=CARTESIAN_POINT ( 'NONE',  ( -58.37499999999996447, -2.944486372867076707, -1.700000000000217781 ) ) ;
#13182=DIRECTION ( 'NONE',  ( 0.000000000000000000, 1.000000000000000000, 0.000000000000000000 ) ) ;
#13199=CARTESIAN_POINT ( 'NONE',  ( -58.68749999999998579, 1.962990915244722689, 3.399999999999799627 ) ) ;
#13204=AXIS2_PLACEMENT_3D ( 'NONE', #13883, #8825, #1879 ) ;
#13210=PLANE ( 'NONE',  #14676 ) ;
#13215=CARTESIAN_POINT ( 'NONE',  ( -59.20655989232412963, 1.962990915244722245, 3.399999999999796962 ) ) ;
#13224=EDGE_CURVE ( 'NONE', #11119, #16069, #6924, .T. ) ;
#13229=CARTESIAN_POINT ( 'NONE',  ( -59.45655989232410121, 1.962990915244762435, -3.400000000000193534 ) ) ;
#13230=VERTEX_POINT ( 'NONE', #2008 ) ;
#13233=CARTESIAN_POINT ( 'NONE',  ( -54.49999999999996447, -1.399999999999979039, -3.959797974644881258 ) ) ;
#13247=CARTESIAN_POINT ( 'NONE',  ( -55.07202994616204705, 2.078460969082674747, -3.600000000000187494 ) ) ;
#13260=PRODUCT_DEFINITION_CONTEXT ( 'detailed design', #16079, 'design' ) ;
#13261=DIRECTION ( 'NONE',  ( -1.499696682456116357E-15, 0.9030524935654929974, 0.4295302013422865883 ) ) ;
#13264=ADVANCED_FACE ( 'NONE', ( #9297 ), #8975, .T. ) ;
#13265=ORIENTED_EDGE ( 'NONE', *, *, #14201, .F. ) ;
#13269=CARTESIAN_POINT ( 'NONE',  ( -60.25952994616203284, 3.117691453623994580, -1.800000000000200329 ) ) ;
#13275=CARTESIAN_POINT ( 'NONE',  ( -59.38929772167340104, 2.352105592641139609, 1.259504355517284457 ) ) ;
#13279=CARTESIAN_POINT ( 'NONE',  ( -60.88452994616204705, 3.117691453623979481, 1.799999999999795985 ) ) ;
#13294=CARTESIAN_POINT ( 'NONE',  ( -59.19495429951913223, 2.548385458854359964, -0.9469503383365888149 ) ) ;
#13295=DIRECTION ( 'NONE',  ( 1.000000000000000000, -1.219044193948983948E-29, 3.491481338843133355E-15 ) ) ;
#13301=EDGE_CURVE ( 'NONE', #14560, #2157, #13324, .T. ) ;
#13309=CARTESIAN_POINT ( 'NONE',  ( -56.00952994616203995, -3.117691453623961273, -1.800000000000214762 ) ) ;
#13310=CARTESIAN_POINT ( 'NONE',  ( -59.20655989232412963, 1.962990915244722245, 3.399999999999796962 ) ) ;
#13311=VERTEX_POINT ( 'NONE', #20805 ) ;
#13313=ORIENTED_EDGE ( 'NONE', *, *, #29078, .F. ) ;
#13317=CARTESIAN_POINT ( 'NONE',  ( -55.68749999999999289, 1.962990915244722689, 3.399999999999809841 ) ) ;
#13321=CARTESIAN_POINT ( 'NONE',  ( -54.49999999999996447, 2.023778652682504319E-14, -3.400000000000193978 ) ) ;
#13324=LINE ( 'NONE', #5762, #16040 ) ;
#13336=LINE ( 'NONE', #1324, #7319 ) ;
#13340=CARTESIAN_POINT ( 'NONE',  ( -57.24999999999997158, 2.944486372867092250, 1.699999999999808109 ) ) ;
#13341=CARTESIAN_POINT ( 'NONE',  ( -59.40950473592805281, 2.424939707643913867, 1.246983968401823795 ) ) ;
#13352=FACE_OUTER_BOUND ( 'NONE', #17853, .T. ) ;
#13358=CARTESIAN_POINT ( 'NONE',  ( -57.39405989232411542, -2.944486372867076263, -1.700000000000214451 ) ) ;
#13365=CARTESIAN_POINT ( 'NONE',  ( -56.70655989232412963, -3.399999999999991029, -2.112596694108398230E-13 ) ) ;
#13378=DIRECTION ( 'NONE',  ( -1.000000000000000000, 1.219044193948983948E-29, -3.491481338843133355E-15 ) ) ;
#13379=CARTESIAN_POINT ( 'NONE',  ( -44.59999999999996589, -1.499999999999978906, -3.959797974644846619 ) ) ;
#13389=CARTESIAN_POINT ( 'NONE',  ( -54.49999999999997868, -3.188085654472696540, 1.181570928782897267 ) ) ;
#13393=CARTESIAN_POINT ( 'NONE',  ( -54.38452994616203995, 2.093608279459366986E-14, -3.600000000000193268 ) ) ;
#13395=CIRCLE ( 'NONE', #19519, 3.524999999999996358 ) ;
#13399=AXIS2_PLACEMENT_3D ( 'NONE', #14197, #26239, #18656 ) ;
#13403=CARTESIAN_POINT ( 'NONE',  ( -54.39999999999996305, 1.400000000000023670, -3.959797974644871044 ) ) ;
#13405=EDGE_CURVE ( 'NONE', #4631, #19660, #8990, .T. ) ;
#13406=CARTESIAN_POINT ( 'NONE',  ( -56.93749999999996447, -3.399999999999991473, -2.119568960425587465E-13 ) ) ;
#13411=EDGE_CURVE ( 'NONE', #7915, #23830, #9346, .T. ) ;
#13426=CIRCLE ( 'NONE', #10426, 0.09999999999999995004 ) ;
#13428=CARTESIAN_POINT ( 'NONE',  ( -59.39436078131932817, 2.362401244263863997, 1.255862057041944535 ) ) ;
#13429=VECTOR ( 'NONE', #19382, 1000.000000000000000 ) ;
#13436=CARTESIAN_POINT ( 'NONE',  ( -59.32267277260975646, 3.229247813185812888, 1.250136525132572451 ) ) ;
#13443=AXIS2_PLACEMENT_3D ( 'NONE', #7990, #17329, #15262 ) ;
#13462=B_SPLINE_CURVE_WITH_KNOTS ( 'NONE', 3,
 ( #17013, #26193, #2270, #12102, #2116, #19243, #28733, #29032, #28882, #2442 ),
 .UNSPECIFIED., .F., .F.,
 ( 4, 3, 3, 4 ),
 ( 1.252429503699613567E-17, 0.0001369029408772380434, 0.0002053557494648628661, 0.0002738089271645095064 ),
 .UNSPECIFIED. ) ;
#13469=ORIENTED_EDGE ( 'NONE', *, *, #24601, .F. ) ;
#13472=CARTESIAN_POINT ( 'NONE',  ( -54.94702994616205416, 4.156921938165313968, -1.801810997602979365E-13 ) ) ;
#13474=CARTESIAN_POINT ( 'NONE',  ( -58.89405989232411542, -2.944486372867076263, -1.700000000000219558 ) ) ;
#13481=CIRCLE ( 'NONE', #13982, 3.624999999999996447 ) ;
#13482=CARTESIAN_POINT ( 'NONE',  ( -57.87499999999997868, -3.920666489018319112E-15, 3.399999999999793854 ) ) ;
#13487=CARTESIAN_POINT ( 'NONE',  ( -56.56249999999997158, 3.400000000000008349, -1.863919195461975120E-13 ) ) ;
#13492=DIRECTION ( 'NONE',  ( -1.000000000000000000, -0.000000000000000000, 0.000000000000000000 ) ) ;
#13494=VECTOR ( 'NONE', #13378, 1000.000000000000000 ) ;
#13496=CARTESIAN_POINT ( 'NONE',  ( -59.60675767627765964, 2.338930541566064392, -1.245993773302328744 ) ) ;
#13507=TOROIDAL_SURFACE ( 'NONE', #14008, 3.525000000000025224, 0.1000000000000000056 ) ;
#13513=CARTESIAN_POINT ( 'NONE',  ( -57.81249999999998579, -1.962990915244731793, 3.399999999999786304 ) ) ;
#13524=CARTESIAN_POINT ( 'NONE',  ( -54.46614378277664059, -2.255560380866761250, -2.805788190199900889 ) ) ;
#13533=ADVANCED_FACE ( 'NONE', ( #21589 ), #2088, .F. ) ;
#13538=FACE_OUTER_BOUND ( 'NONE', #3119, .T. ) ;
#13539=CARTESIAN_POINT ( 'NONE',  ( -59.49861073854652460, -2.239724662550681700, 1.422539515414428024 ) ) ;
#13548=ORIENTED_EDGE ( 'NONE', *, *, #6577, .F. ) ;
#13549=( BOUNDED_CURVE ( )  B_SPLINE_CURVE ( 2, ( #31179, #1893, #11558, #16454, #4425, #23902, #2195, #13590, #14073 ),
 .UNSPECIFIED., .F., .T. ) 
 B_SPLINE_CURVE_WITH_KNOTS ( ( 3, 2, 2, 2, 3 ),
 ( 0.1388888888888888951, 0.1481481481481481399, 0.1666666666666666574, 0.1851851851851851749, 0.1944444444444444475 ),
 .UNSPECIFIED. ) 
 CURVE ( )  GEOMETRIC_REPRESENTATION_ITEM ( )  RATIONAL_B_SPLINE_CURVE ( ( 0.9330127018922192983, 0.9330127018922194093, 1.000000000000000000, 0.8660254037844387076, 1.000000000000000000, 0.8660254037844387076, 1.000000000000000000, 0.9330127018922191873, 0.9330127018922192983 ) ) 
 REPRESENTATION_ITEM ( '' )  );
#13564=CARTESIAN_POINT ( 'NONE',  ( -54.49999999999996447, -1.599999999999981215, -3.363870538531692489 ) ) ;
#13565=DIRECTION ( 'NONE',  ( 1.000000000000000000, -1.219044193948983948E-29, 3.491481338843133355E-15 ) ) ;
#13567=CARTESIAN_POINT ( 'NONE',  ( -56.00952994616203995, -3.117691453623963938, -1.800000000000210099 ) ) ;
#13570=EDGE_CURVE ( 'NONE', #3568, #1750, #30659, .T. ) ;
#13586=CARTESIAN_POINT ( 'NONE',  ( -60.07202994616204705, 2.078460969082646770, 3.599999999999794031 ) ) ;
#13588=ORIENTED_EDGE ( 'NONE', *, *, #19754, .F. ) ;
#13590=CARTESIAN_POINT ( 'NONE',  ( -55.54806624327024167, 3.400000000000003908, 0.9110272542656333572 ) ) ;
#13594=AXIS2_PLACEMENT_3D ( 'NONE', #15292, #11166, #11488 ) ;
#13595=ORIENTED_EDGE ( 'NONE', *, *, #26940, .T. ) ;
#13598=CIRCLE ( 'NONE', #31316, 0.1000000000000000472 ) ;
#13601=CARTESIAN_POINT ( 'NONE',  ( -54.39999999999999147, 1.399999999999995914, 3.959797974644419849 ) ) ;
#13614=CARTESIAN_POINT ( 'NONE',  ( -59.61639066107911589, -2.342446846742894717, -1.242019481833328776 ) ) ;
#13622=EDGE_CURVE ( 'NONE', #20056, #30092, #4539, .T. ) ;
#13625=CARTESIAN_POINT ( 'NONE',  ( -59.69999999999995310, -3.120538811013533032, -1.606221934090561687 ) ) ;
#13628=SURFACE_STYLE_FILL_AREA ( #6210 ) ;
#13631=CARTESIAN_POINT ( 'NONE',  ( -57.58155989232413674, -1.962990915244731571, 3.399999999999786748 ) ) ;
#13639=CARTESIAN_POINT ( 'NONE',  ( -56.56249999999997158, 3.925981830489463142, -1.866702293926226148E-13 ) ) ;
#13644=EDGE_CURVE ( 'NONE', #30441, #10060, #19215, .T. ) ;
#13649=CARTESIAN_POINT ( 'NONE',  ( -59.60063969940316753, 2.337287690019632880, -1.248834004845440715 ) ) ;
#13655=ORIENTED_EDGE ( 'NONE', *, *, #30536, .T. ) ;
#13662=CARTESIAN_POINT ( 'NONE',  ( -60.68749999999996447, -3.925981830489445379, -2.294491627273766911E-13 ) ) ;
#13664=ORIENTED_EDGE ( 'NONE', *, *, #10781, .T. ) ;
#13674=FACE_OUTER_BOUND ( 'NONE', #15641, .T. ) ;
#13677=ORIENTED_EDGE ( 'NONE', *, *, #9841, .T. ) ;
#13697=VERTEX_POINT ( 'NONE', #17601 ) ;
#13704=VERTEX_POINT ( 'NONE', #22501 ) ;
#13719=CARTESIAN_POINT ( 'NONE',  ( -57.94702994616203995, 4.156921938165313080, -1.906555437768272735E-13 ) ) ;
#13746=DIRECTION ( 'NONE',  ( 0.000000000000000000, -1.000000000000000000, 0.000000000000000000 ) ) ;
#13755=DIRECTION ( 'NONE',  ( -1.000000000000000000, 1.219044193948983948E-29, -3.491481338843133355E-15 ) ) ;
#13764=CARTESIAN_POINT ( 'NONE',  ( -59.69999999999997442, 8.366749974758454467E-15, -2.120534355533670266E-13 ) ) ;
#13776=VERTEX_POINT ( 'NONE', #2203 ) ;
#13778=CARTESIAN_POINT ( 'NONE',  ( -55.32202994616205416, -4.156921938165296204, -2.162464288268359870E-13 ) ) ;
#13779=CARTESIAN_POINT ( 'NONE',  ( -57.33155989232411542, -1.962990915244706924, -3.400000000000209521 ) ) ;
#13780=ORIENTED_EDGE ( 'NONE', *, *, #2713, .F. ) ;
#13781=ORIENTED_EDGE ( 'NONE', *, *, #9569, .F. ) ;
#13784=CARTESIAN_POINT ( 'NONE',  ( -55.13452994616203995, 2.093608279459367933E-14, -3.600000000000195932 ) ) ;
#13785=CARTESIAN_POINT ( 'NONE',  ( -55.14405989232412253, -2.944486372867075819, -1.700000000000207345 ) ) ;
#13787=VECTOR ( 'NONE', #24347, 1000.000000000000000 ) ;
#13807=CARTESIAN_POINT ( 'NONE',  ( -59.81249999999995026, -1.962990915244707368, -3.400000000000219291 ) ) ;
#13825=CYLINDRICAL_SURFACE ( 'NONE', #298, 3.399999999999999911 ) ;
#13832=EDGE_CURVE ( 'NONE', #826, #1451, #4946, .T. ) ;
#13863=CARTESIAN_POINT ( 'NONE',  ( -59.38452994616203995, 3.117691453623979481, 1.799999999999801092 ) ) ;
#13870=CARTESIAN_POINT ( 'NONE',  ( -55.64405989232412253, 2.944486372867106905, -1.700000000000184253 ) ) ;
#13873=VERTEX_POINT ( 'NONE', #25608 ) ;
#13883=CARTESIAN_POINT ( 'NONE',  ( -54.49999999999997868, -6.102218906431378987E-14, -2.216533082070118739E-13 ) ) ;
#13888=ORIENTED_EDGE ( 'NONE', *, *, #2095, .T. ) ;
#13922=CARTESIAN_POINT ( 'NONE',  ( -59.19999999999996732, -2.580747833305891970, -0.9498634748674686934 ) ) ;
#13934=ORIENTED_EDGE ( 'NONE', *, *, #6790, .T. ) ;
#13941=CARTESIAN_POINT ( 'NONE',  ( -60.26905989232410121, 2.023778652682511261E-14, -3.400000000000213518 ) ) ;
#13942=ORIENTED_EDGE ( 'NONE', *, *, #11013, .F. ) ;
#13946=CARTESIAN_POINT ( 'NONE',  ( -56.07202994616204705, -4.156921938165296204, -2.141547992439359634E-13 ) ) ;
#13950=CARTESIAN_POINT ( 'NONE',  ( -59.19495429951913223, -2.548385458854336871, -0.9469503383366065785 ) ) ;
#13971=AXIS2_PLACEMENT_3D ( 'NONE', #12958, #22327, #5842 ) ;
#13975=CARTESIAN_POINT ( 'NONE',  ( -54.69702994616206837, -2.078460969082657872, 3.599999999999797584 ) ) ;
#13981=ORIENTED_EDGE ( 'NONE', *, *, #7094, .T. ) ;
#13982=AXIS2_PLACEMENT_3D ( 'NONE', #9196, #16466, #1577 ) ;
#13993=CARTESIAN_POINT ( 'NONE',  ( -44.59999999999997300, -4.766731106216475591E-14, -1.489237264809750408E-13 ) ) ;
#14008=AXIS2_PLACEMENT_3D ( 'NONE', #14837, #24498, #12021 ) ;
#14012=EDGE_CURVE ( 'NONE', #23000, #16551, #16978, .T. ) ;
#14032=EDGE_CURVE ( 'NONE', #15811, #6214, #106, .T. ) ;
#14037=CARTESIAN_POINT ( 'NONE',  ( -57.19702994616204705, 4.156921938165313080, -1.880369327726949834E-13 ) ) ;
#14051=CARTESIAN_POINT ( 'NONE',  ( -44.49999999999997868, -3.524999999999988365, -1.993951146718866384E-13 ) ) ;
#14063=ORIENTED_EDGE ( 'NONE', *, *, #16676, .F. ) ;
#14064=CARTESIAN_POINT ( 'NONE',  ( -59.09665968485343512, -2.466443774698472424, -0.9691001528487745986 ) ) ;
#14073=CARTESIAN_POINT ( 'NONE',  ( -55.58155989232413674, 3.400000000000007461, -1.857527951337884861E-13 ) ) ;
#14105=EDGE_LOOP ( 'NONE', ( #12333, #8791, #92, #19357 ) ) ;
#14115=CARTESIAN_POINT ( 'NONE',  ( -59.76905989232412253, -2.944486372867088697, 1.699999999999776579 ) ) ;
#14122=CIRCLE ( 'NONE', #26287, 0.1000000000000001860 ) ;
#14123=CARTESIAN_POINT ( 'NONE',  ( -59.31249999999997868, -1.962990915244731793, 3.399999999999781419 ) ) ;
#14132=ORIENTED_EDGE ( 'NONE', *, *, #21725, .F. ) ;
#14142=AXIS2_PLACEMENT_3D ( 'NONE', #10901, #5848, #15674 ) ;
#14144=ORIENTED_EDGE ( 'NONE', *, *, #7501, .T. ) ;
#14147=CARTESIAN_POINT ( 'NONE',  ( -60.06249999999997868, -1.962990915244731793, 3.399999999999778755 ) ) ;
#14149=ORIENTED_EDGE ( 'NONE', *, *, #6459, .F. ) ;
#14155=CARTESIAN_POINT ( 'NONE',  ( -57.94702994616203995, 4.156921938165313080, -1.906555437768272735E-13 ) ) ;
#14162=ORIENTED_EDGE ( 'NONE', *, *, #30716, .T. ) ;
#14165=DIRECTION ( 'NONE',  ( 1.000000000000000000, -1.219044193948983948E-29, 3.491481338843133355E-15 ) ) ;
#14176=ORIENTED_EDGE ( 'NONE', *, *, #13044, .F. ) ;
#14178=CARTESIAN_POINT ( 'NONE',  ( -59.13776767298602977, -2.346568386202238177, 1.245686009234607150 ) ) ;
#14197=CARTESIAN_POINT ( 'NONE',  ( -54.39999999999996305, -1.399999999999979039, -3.959797974644881258 ) ) ;
#14199=CARTESIAN_POINT ( 'NONE',  ( -56.19702994616206837, -2.078460969082657872, 3.599999999999791811 ) ) ;
#14200=CARTESIAN_POINT ( 'NONE',  ( -59.10189254065529951, -2.466111651437300267, -0.9699939416073426468 ) ) ;
#14201=EDGE_CURVE ( 'NONE', #2157, #12035, #29859, .T. ) ;
#14206=DIRECTION ( 'NONE',  ( 0.000000000000000000, 1.000000000000000000, 3.491481338843130594E-15 ) ) ;
#14215=CARTESIAN_POINT ( 'NONE',  ( -57.43749999999995737, 1.962990915244761103, -3.400000000000188205 ) ) ;
#14221=DIRECTION ( 'NONE',  ( 0.000000000000000000, 1.000000000000000000, 8.673617379884030739E-15 ) ) ;
#14227=DIRECTION ( 'NONE',  ( -1.499696682456116357E-15, -0.9030524935654959950, 0.4295302013422802601 ) ) ;
#14246=LINE ( 'NONE', #6336, #18474 ) ;
#14251=DIRECTION ( 'NONE',  ( -0.000000000000000000, 1.000000000000000000, 3.491481338843133355E-15 ) ) ;
#14253=AXIS2_PLACEMENT_3D ( 'NONE', #27719, #8548, #15688 ) ;
#14279=CARTESIAN_POINT ( 'NONE',  ( -54.50952994616204705, -3.117691453623963938, -1.800000000000204770 ) ) ;
#14301=CARTESIAN_POINT ( 'NONE',  ( -60.12499999999997868, -3.920666489018291502E-15, 3.399999999999785860 ) ) ;
#14307=CARTESIAN_POINT ( 'NONE',  ( -58.32202994616204705, -4.156921938165296204, -2.220106322563329850E-13 ) ) ;
#14323=EDGE_CURVE ( 'NONE', #6036, #18483, #29168, .T. ) ;
#14350=CARTESIAN_POINT ( 'NONE',  ( -56.64405989232412253, -2.944486372867076263, -1.700000000000211786 ) ) ;
#14351=CARTESIAN_POINT ( 'NONE',  ( -59.15783187464324300, -2.494370574884575920, -0.9479319139174872122 ) ) ;
#14352=CARTESIAN_POINT ( 'NONE',  ( -58.62499999999998579, -2.016369211404101147E-14, 3.399999999999791189 ) ) ;
#14357=DIRECTION ( 'NONE',  ( -0.5000000000000029976, -3.023711536277451078E-15, 0.8660254037844369313 ) ) ;
#14360=DIRECTION ( 'NONE',  ( 0.000000000000000000, 1.000000000000000000, -1.030899290251718945E-13 ) ) ;
#14365=( NAMED_UNIT ( * ) SI_UNIT ( $, .STERADIAN. ) SOLID_ANGLE_UNIT ( ) );
#14366=VECTOR ( 'NONE', #7613, 1000.000000000000000 ) ;
#14379=CARTESIAN_POINT ( 'NONE',  ( -44.59999999999996589, -1.514093959731525496, -3.183260039818558873 ) ) ;
#14381=DIRECTION ( 'NONE',  ( 0.000000000000000000, -4.336808689942024836E-15, 1.000000000000000000 ) ) ;
#14387=ADVANCED_FACE ( 'NONE', ( #30801 ), #25737, .T. ) ;
#14404=PLANE ( 'NONE',  #22189 ) ;
#14413=VERTEX_POINT ( 'NONE', #20995 ) ;
#14420=CARTESIAN_POINT ( 'NONE',  ( -60.01905989232411542, 2.944486372867092250, 1.699999999999798339 ) ) ;
#14427=CARTESIAN_POINT ( 'NONE',  ( -54.82202994616206126, 2.078460969082646770, 3.599999999999812683 ) ) ;
#14431=CIRCLE ( 'NONE', #3800, 0.1000000000000000472 ) ;
#14437=EDGE_CURVE ( 'NONE', #30441, #18960, #7761, .T. ) ;
#14439=CARTESIAN_POINT ( 'NONE',  ( -55.43749999999997868, -3.399999999999991473, -2.094585006122325661E-13 ) ) ;
#14455=CARTESIAN_POINT ( 'NONE',  ( -56.57202994616203995, 2.078460969082674747, -3.600000000000191935 ) ) ;
#14456=ORIENTED_EDGE ( 'NONE', *, *, #1306, .T. ) ;
#14463=CARTESIAN_POINT ( 'NONE',  ( -56.82202994616205416, -4.156921938165296204, -2.167734102480683039E-13 ) ) ;
#14468=CIRCLE ( 'NONE', #807, 3.525000000000025224 ) ;
#14476=ADVANCED_FACE ( 'NONE', ( #19974 ), #29613, .T. ) ;
#14481=AXIS2_PLACEMENT_3D ( 'NONE', #6065, #10650, #22853 ) ;
#14484=EDGE_CURVE ( 'NONE', #17625, #19844, #3332, .T. ) ;
#14487=CARTESIAN_POINT ( 'NONE',  ( -54.49999999999997868, -4.766731106216463600E-14, -1.834893917355220926E-13 ) ) ;
#14494=CARTESIAN_POINT ( 'NONE',  ( -59.69999999999998153, 3.161828374300071687, 1.250136525132549581 ) ) ;
#14502=ORIENTED_EDGE ( 'NONE', *, *, #29487, .T. ) ;
#14504=ORIENTED_EDGE ( 'NONE', *, *, #11318, .F. ) ;
#14512=DIRECTION ( 'NONE',  ( 0.000000000000000000, 1.000000000000000000, 3.491481338843130594E-15 ) ) ;
#14513=CIRCLE ( 'NONE', #29665, 3.399999999999999911 ) ;
#14518=CARTESIAN_POINT ( 'NONE',  ( -55.58155989232412963, 3.925981830489463142, -1.832452953121496317E-13 ) ) ;
#14538=ORIENTED_EDGE ( 'NONE', *, *, #29078, .T. ) ;
#14560=VERTEX_POINT ( 'NONE', #2135 ) ;
#14563=VECTOR ( 'NONE', #24242, 1000.000000000000000 ) ;
#14573=ORIENTED_EDGE ( 'NONE', *, *, #8053, .T. ) ;
#14582=AXIS2_PLACEMENT_3D ( 'NONE', #19711, #27282, #12852 ) ;
#14589=ORIENTED_EDGE ( 'NONE', *, *, #13411, .T. ) ;
#14595=CARTESIAN_POINT ( 'NONE',  ( -59.38452994616203995, 3.117691453623979481, 1.799999999999801092 ) ) ;
#14601=AXIS2_PLACEMENT_3D ( 'NONE', #4704, #24199, #14360 ) ;
#14606=CYLINDRICAL_SURFACE ( 'NONE', #4356, 3.399999999999999911 ) ;
#14609=DIRECTION ( 'NONE',  ( 0.000000000000000000, -1.000000000000000000, -3.491481338843129805E-15 ) ) ;
#14615=ORIENTED_EDGE ( 'NONE', *, *, #18655, .F. ) ;
#14617=CARTESIAN_POINT ( 'NONE',  ( -56.75952994616203995, -3.117691453623963938, -1.800000000000212763 ) ) ;
#14625=CARTESIAN_POINT ( 'NONE',  ( -57.00952994616205416, -4.643455692769903542E-15, 3.599999999999796696 ) ) ;
#14633=CARTESIAN_POINT ( 'NONE',  ( -54.56249999999997158, -1.962990915244707368, -3.400000000000200640 ) ) ;
#14637=CARTESIAN_POINT ( 'NONE',  ( -59.65990137405635352, 2.396397731248872010, -2.649317374334408726 ) ) ;
#14648=AXIS2_PLACEMENT_3D ( 'NONE', #13601, #1425, #28016 ) ;
#14656=CARTESIAN_POINT ( 'NONE',  ( -54.49999999999996447, 2.023778652682504319E-14, -3.400000000000193978 ) ) ;
#14659=VERTEX_POINT ( 'NONE', #3648 ) ;
#14660=DIRECTION ( 'NONE',  ( 0.000000000000000000, 1.000000000000000000, 3.491481338843132961E-15 ) ) ;
#14663=EDGE_CURVE ( 'NONE', #17201, #21866, #23027, .T. ) ;
#14672=FACE_OUTER_BOUND ( 'NONE', #8425, .T. ) ;
#14674=CARTESIAN_POINT ( 'NONE',  ( -55.08155989232411542, -1.962990915244706924, -3.400000000000202416 ) ) ;
#14676=AXIS2_PLACEMENT_3D ( 'NONE', #11155, #22894, #27791 ) ;
#14681=EDGE_CURVE ( 'NONE', #16115, #19668, #28393, .T. ) ;
#14684=CARTESIAN_POINT ( 'NONE',  ( -59.69977646026288909, -2.446662296333478537, -1.238409548734900278 ) ) ;
#14697=DIRECTION ( 'NONE',  ( 0.000000000000000000, 1.000000000000000000, 4.336808689942015369E-15 ) ) ;
#14721=ORIENTED_EDGE ( 'NONE', *, *, #15635, .F. ) ;
#14727=DIRECTION ( 'NONE',  ( -1.000000000000000000, 1.219044193948983948E-29, -3.491481338843133355E-15 ) ) ;
#14733=CARTESIAN_POINT ( 'NONE',  ( -59.19999999999996732, 4.156921938165317520, -0.9498634748674451567 ) ) ;
#14743=CARTESIAN_POINT ( 'NONE',  ( -56.75952994616203995, -3.117691453623963938, -1.800000000000212763 ) ) ;
#14748=CARTESIAN_POINT ( 'NONE',  ( -58.83155989232410832, -1.962990915244687828, -3.400000000000225953 ) ) ;
#14753=CARTESIAN_POINT ( 'NONE',  ( -44.49999999999999289, -1.600000000000004530, 3.363870538531272381 ) ) ;
#14757=B_SPLINE_CURVE_WITH_KNOTS ( 'NONE', 3,
 ( #1311, #10816, #5929, #23189, #17957, #15736, #30436, #3228, #22555, #17812 ),
 .UNSPECIFIED., .F., .F.,
 ( 4, 3, 3, 4 ),
 ( 0.000000000000000000, 1.446898074592995643E-05, 3.359950008203892456E-05, 3.648946756727797501E-05 ),
 .UNSPECIFIED. ) ;
#14760=( BOUNDED_CURVE ( )  B_SPLINE_CURVE ( 2, ( #14889, #15059, #17761, #3177, #12817, #642, #7935, #13142, #22502 ),
 .UNSPECIFIED., .F., .T. ) 
 B_SPLINE_CURVE_WITH_KNOTS ( ( 3, 2, 2, 2, 3 ),
 ( 0.3055555555555555802, 0.3148148148148148251, 0.3333333333333333148, 0.3518518518518518601, 0.3611111111111111605 ),
 .UNSPECIFIED. ) 
 CURVE ( )  GEOMETRIC_REPRESENTATION_ITEM ( )  RATIONAL_B_SPLINE_CURVE ( ( 0.9330127018922194093, 0.9330127018922195203, 1.000000000000000000, 0.8660254037844387076, 1.000000000000000000, 0.8660254037844387076, 1.000000000000000000, 0.9330127018922189652, 0.9330127018922194093 ) ) 
 REPRESENTATION_ITEM ( '' )  );
#14764=CARTESIAN_POINT ( 'NONE',  ( -58.31249999999995737, -1.962990915244701151, -3.400000000000217515 ) ) ;
#14770=ORIENTED_EDGE ( 'NONE', *, *, #3145, .F. ) ;
#14773=LINE ( 'NONE', #16860, #4553 ) ;
#14774=ADVANCED_FACE ( 'NONE', ( #9348 ), #19015, .F. ) ;
#14775=CARTESIAN_POINT ( 'NONE',  ( -54.63452994616206126, -3.117691453623976816, 1.799999999999793765 ) ) ;
#14780=ORIENTED_EDGE ( 'NONE', *, *, #10356, .T. ) ;
#14781=CARTESIAN_POINT ( 'NONE',  ( -59.19999999999997442, -3.222669219888746550, 1.250136525132528931 ) ) ;
#14787=DIRECTION ( 'NONE',  ( -2.081668171172170028E-13, -0.4295302013422817033, -0.9030524935654953289 ) ) ;
#14791=PLANE ( 'NONE',  #30635 ) ;
#14792=EDGE_CURVE ( 'NONE', #3421, #9593, #13481, .T. ) ;
#14812=CARTESIAN_POINT ( 'NONE',  ( -54.83155989232412963, 3.925981830489463142, -1.806266843080172912E-13 ) ) ;
#14828=VERTEX_POINT ( 'NONE', #29284 ) ;
#14837=CARTESIAN_POINT ( 'NONE',  ( -44.59999999999997300, -6.102218906431391608E-14, -1.870876429524648473E-13 ) ) ;
#14846=CARTESIAN_POINT ( 'NONE',  ( -44.59999999999998721, 1.599999999999998090, 3.363870538531281706 ) ) ;
#14853=DIRECTION ( 'NONE',  ( 0.000000000000000000, -4.336808689942006692E-15, 1.000000000000000000 ) ) ;
#14874=( BOUNDED_CURVE ( )  B_SPLINE_CURVE ( 2, ( #20005, #2746, #7797, #5124, #19554, #9878, #527, #26673, #22241 ),
 .UNSPECIFIED., .F., .T. ) 
 B_SPLINE_CURVE_WITH_KNOTS ( ( 3, 2, 2, 2, 3 ),
 ( 0.2500000000000000000, 0.2592592592592592449, 0.2777777777777777901, 0.2962962962962962798, 0.3055555555555555802 ),
 .UNSPECIFIED. ) 
 CURVE ( )  GEOMETRIC_REPRESENTATION_ITEM ( )  RATIONAL_B_SPLINE_CURVE ( ( 0.9330127018922192983, 0.9330127018922194093, 1.000000000000000000, 0.8660254037844387076, 1.000000000000000000, 0.8660254037844387076, 1.000000000000000000, 0.9330127018922191873, 0.9330127018922194093 ) ) 
 REPRESENTATION_ITEM ( '' )  );
#14881=DIRECTION ( 'NONE',  ( 0.000000000000000000, -0.3333333333333282633, 0.9428090415820651327 ) ) ;
#14886=CARTESIAN_POINT ( 'NONE',  ( -57.75952994616205416, -4.643455692769894075E-15, 3.599999999999794031 ) ) ;
#14887=ADVANCED_FACE ( 'NONE', ( #12043 ), #27594, .T. ) ;
#14889=CARTESIAN_POINT ( 'NONE',  ( -56.33155989232412963, 3.400000000000008349, -1.856946929144785632E-13 ) ) ;
#14900=ADVANCED_FACE ( 'NONE', ( #19644 ), #10270, .T. ) ;
#14906=DIRECTION ( 'NONE',  ( -1.000000000000000000, 1.219044193948983948E-29, -3.491481338843133355E-15 ) ) ;
#14912=FACE_OUTER_BOUND ( 'NONE', #16977, .T. ) ;
#14918=CARTESIAN_POINT ( 'NONE',  ( -55.33155989232414385, -1.962990915244731571, 3.399999999999794742 ) ) ;
#14955=ORIENTED_EDGE ( 'NONE', *, *, #26257, .T. ) ;
#14958=ORIENTED_EDGE ( 'NONE', *, *, #15259, .F. ) ;
#14962=CARTESIAN_POINT ( 'NONE',  ( -57.45655989232412253, -3.399999999999991029, -2.148039047887444390E-13 ) ) ;
#14968=CARTESIAN_POINT ( 'NONE',  ( -61.00952994616203284, 3.117691453623994580, -1.800000000000202993 ) ) ;
#15002=ORIENTED_EDGE ( 'NONE', *, *, #13411, .F. ) ;
#15005=AXIS2_PLACEMENT_3D ( 'NONE', #9389, #19059, #7024 ) ;
#15010=CARTESIAN_POINT ( 'NONE',  ( -59.69999999999996021, 1.397030005794335672, -3.099726949734703751 ) ) ;
#15024=CARTESIAN_POINT ( 'NONE',  ( -57.63452994616205416, -3.117691453623982589, 1.799999999999773337 ) ) ;
#15043=ORIENTED_EDGE ( 'NONE', *, *, #12922, .T. ) ;
#15044=ADVANCED_FACE ( 'NONE', ( #11353 ), #17076, .T. ) ;
#15045=CARTESIAN_POINT ( 'NONE',  ( -59.19312575602410931, 2.408440864227364919, 1.250136525132548693 ) ) ;
#15051=CARTESIAN_POINT ( 'NONE',  ( -54.39999999999999147, -1.400000000000006795, 3.959797974644449603 ) ) ;
#15055=ORIENTED_EDGE ( 'NONE', *, *, #6148, .F. ) ;
#15057=CARTESIAN_POINT ( 'NONE',  ( -57.57202994616204705, -4.156921938165296204, -2.193920212522006445E-13 ) ) ;
#15059=CARTESIAN_POINT ( 'NONE',  ( -56.36505354137801049, 3.400000000000011902, -0.9110272542659988426 ) ) ;
#15063=CARTESIAN_POINT ( 'NONE',  ( -59.54784193156670113, -3.076428338433373710, 1.450963157958014449 ) ) ;
#15069=CARTESIAN_POINT ( 'NONE',  ( -54.49999999999996447, -1.399999999999981259, -3.300094695611242468 ) ) ;
#15071=( BOUNDED_CURVE ( )  B_SPLINE_CURVE ( 2, ( #29101, #6954, #2032, #14215, #19308, #16920, #4711, #7251, #25937 ),
 .UNSPECIFIED., .F., .T. ) 
 B_SPLINE_CURVE_WITH_KNOTS ( ( 3, 2, 2, 2, 3 ),
 ( 0.4166666666666666852, 0.4259259259259259300, 0.4444444444444444198, 0.4629629629629629650, 0.4722222222222222654 ),
 .UNSPECIFIED. ) 
 CURVE ( )  GEOMETRIC_REPRESENTATION_ITEM ( )  RATIONAL_B_SPLINE_CURVE ( ( 0.9330127018922194093, 0.9330127018922195203, 1.000000000000000000, 0.8660254037844387076, 1.000000000000000000, 0.8660254037844387076, 1.000000000000000000, 0.9330127018922189652, 0.9330127018922194093 ) ) 
 REPRESENTATION_ITEM ( '' )  );
#15083=EDGE_CURVE ( 'NONE', #21866, #30858, #11189, .T. ) ;
#15088=VERTEX_POINT ( 'NONE', #2648 ) ;
#15090=CARTESIAN_POINT ( 'NONE',  ( -54.51905989232412963, -2.944486372867088697, 1.699999999999795008 ) ) ;
#15093=DIRECTION ( 'NONE',  ( -2.095850865446309212E-30, -1.000000000000000000, -2.891205793294679411E-15 ) ) ;
#15096=ORIENTED_EDGE ( 'NONE', *, *, #17352, .T. ) ;
#15098=DIRECTION ( 'NONE',  ( -1.000000000000000000, 0.000000000000000000, -3.491481338843153471E-15 ) ) ;
#15115=EDGE_CURVE ( 'NONE', #17127, #7637, #7398, .T. ) ;
#15119=CARTESIAN_POINT ( 'NONE',  ( -59.32290219554960942, 2.336760081911408271, 1.249820915005386279 ) ) ;
#15132=ADVANCED_FACE ( 'NONE', ( #5799 ), #19146, .T. ) ;
#15134=CARTESIAN_POINT ( 'NONE',  ( -59.45655989232410832, 1.962990915244748891, -3.400000000000202416 ) ) ;
#15142=CARTESIAN_POINT ( 'NONE',  ( -59.14664939113121278, -2.420129821023009331, 1.219334536740721564 ) ) ;
#15143=CARTESIAN_POINT ( 'NONE',  ( -59.14665968485343228, 2.559517124687116230, -0.9190674295589398302 ) ) ;
#15155=CARTESIAN_POINT ( 'NONE',  ( -59.19376570361661294, -3.399999999999992362, 0.1704271383727704869 ) ) ;
#15170=CARTESIAN_POINT ( 'NONE',  ( -54.39999999999996305, 1.400000000000021450, -3.363870538531680499 ) ) ;
#15175=CARTESIAN_POINT ( 'NONE',  ( -54.50952994616204705, -3.117691453623963938, -1.800000000000204770 ) ) ;
#15183=CARTESIAN_POINT ( 'NONE',  ( -56.69702994616203284, -2.078460969082626342, -3.600000000000210587 ) ) ;
#15188=ADVANCED_FACE ( 'NONE', ( #902 ), #22547, .T. ) ;
#15195=EDGE_CURVE ( 'NONE', #11984, #16075, #789, .T. ) ;
#15198=CARTESIAN_POINT ( 'NONE',  ( -59.26905989232412253, 2.944486372867082480, 1.699999999999818101 ) ) ;
#15200=ORIENTED_EDGE ( 'NONE', *, *, #16045, .F. ) ;
#15201=CARTESIAN_POINT ( 'NONE',  ( -56.13452994616205416, -3.117691453623976816, 1.799999999999788436 ) ) ;
#15211=CARTESIAN_POINT ( 'NONE',  ( -56.19702994616206837, -2.078460969082657872, 3.599999999999791811 ) ) ;
#15218=CARTESIAN_POINT ( 'NONE',  ( -56.90400635094607651, -3.399999999999988809, -0.9110272542660338146 ) ) ;
#15232=CARTESIAN_POINT ( 'NONE',  ( -58.09599364905385244, 3.400000000000014122, -0.9110272542660006190 ) ) ;
#15233=ADVANCED_FACE ( 'NONE', ( #27178 ), #22941, .T. ) ;
#15237=ORIENTED_EDGE ( 'NONE', *, *, #10891, .T. ) ;
#15238=FACE_OUTER_BOUND ( 'NONE', #2703, .T. ) ;
#15245=CARTESIAN_POINT ( 'NONE',  ( -59.57202994616203995, 2.078460969082674747, -3.600000000000202593 ) ) ;
#15248=ORIENTED_EDGE ( 'NONE', *, *, #7228, .T. ) ;
#15257=CARTESIAN_POINT ( 'NONE',  ( -54.39999999999997016, -1.514093959731525274, -3.183260039818592624 ) ) ;
#15258=( BOUNDED_CURVE ( )  B_SPLINE_CURVE ( 2, ( #2808, #22305, #17546, #3128, #12461, #5816, #20088, #29726, #5332 ),
 .UNSPECIFIED., .F., .T. ) 
 B_SPLINE_CURVE_WITH_KNOTS ( ( 3, 2, 2, 2, 3 ),
 ( 0.4722222222222222654, 0.4814814814814814548, 0.5000000000000000000, 0.5185185185185184897, 0.5277777777777777901 ),
 .UNSPECIFIED. ) 
 CURVE ( )  GEOMETRIC_REPRESENTATION_ITEM ( )  RATIONAL_B_SPLINE_CURVE ( ( 0.9330127018922194093, 0.9330127018922197424, 1.000000000000000000, 0.8660254037844387076, 1.000000000000000000, 0.8660254037844387076, 1.000000000000000000, 0.9330127018922194093, 0.9330127018922194093 ) ) 
 REPRESENTATION_ITEM ( '' )  );
#15259=EDGE_CURVE ( 'NONE', #6022, #17883, #21040, .T. ) ;
#15262=DIRECTION ( 'NONE',  ( 0.000000000000000000, -1.000000000000000000, -3.491481338843134933E-15 ) ) ;
#15281=VERTEX_POINT ( 'NONE', #21331 ) ;
#15284=CARTESIAN_POINT ( 'NONE',  ( -58.84599364905385954, 3.400000000000015010, -0.9110272542660019512 ) ) ;
#15287=CARTESIAN_POINT ( 'NONE',  ( -60.83155989232411542, 3.925981830489463142, -2.015755723410760408E-13 ) ) ;
#15292=CARTESIAN_POINT ( 'NONE',  ( -59.09999999999997300, 8.366749974758448157E-15, -2.099585467500611340E-13 ) ) ;
#15296=DIRECTION ( 'NONE',  ( -2.095850865446309212E-30, -1.000000000000000000, -2.891205793294679411E-15 ) ) ;
#15315=ORIENTED_EDGE ( 'NONE', *, *, #19827, .T. ) ;
#15319=ORIENTED_EDGE ( 'NONE', *, *, #6941, .F. ) ;
#15331=LINE ( 'NONE', #30507, #4828 ) ;
#15332=CARTESIAN_POINT ( 'NONE',  ( -59.00952994616203284, -3.117691453623959053, -1.800000000000228750 ) ) ;
#15335=ORIENTED_EDGE ( 'NONE', *, *, #5679, .T. ) ;
#15349=CARTESIAN_POINT ( 'NONE',  ( -58.75952994616203284, 3.117691453623994580, -1.800000000000195000 ) ) ;
#15357=VERTEX_POINT ( 'NONE', #23058 ) ;
#15374=EDGE_CURVE ( 'NONE', #6165, #17785, #4341, .T. ) ;
#15383=AXIS2_PLACEMENT_3D ( 'NONE', #15170, #22631, #931 ) ;
#15384=ORIENTED_EDGE ( 'NONE', *, *, #30008, .T. ) ;
#15388=ORIENTED_EDGE ( 'NONE', *, *, #3145, .T. ) ;
#15391=ORIENTED_EDGE ( 'NONE', *, *, #25772, .F. ) ;
#15393=CARTESIAN_POINT ( 'NONE',  ( -59.32202994616204705, 2.078460969082646770, 3.599999999999797140 ) ) ;
#15401=CARTESIAN_POINT ( 'NONE',  ( -57.06249999999997868, -1.962990915244731793, 3.399999999999788969 ) ) ;
#15403=( BOUNDED_CURVE ( )  B_SPLINE_CURVE ( 2, ( #17511, #12591, #26997, #8012, #29849, #22420, #5303, #22583, #14962 ),
 .UNSPECIFIED., .F., .T. ) 
 B_SPLINE_CURVE_WITH_KNOTS ( ( 3, 2, 2, 2, 3 ),
 ( 0.4166666666666666852, 0.4259259259259259300, 0.4444444444444444198, 0.4629629629629629650, 0.4722222222222222654 ),
 .UNSPECIFIED. ) 
 CURVE ( )  GEOMETRIC_REPRESENTATION_ITEM ( )  RATIONAL_B_SPLINE_CURVE ( ( 0.9330127018922194093, 0.9330127018922195203, 1.000000000000000000, 0.8660254037844387076, 1.000000000000000000, 0.8660254037844387076, 1.000000000000000000, 0.9330127018922189652, 0.9330127018922194093 ) ) 
 REPRESENTATION_ITEM ( '' )  );
#15409=AXIS2_PLACEMENT_3D ( 'NONE', #30005, #27949, #30326 ) ;
#15410=CARTESIAN_POINT ( 'NONE',  ( -59.19999999999997442, 8.366749974758448157E-15, -2.103076948839454410E-13 ) ) ;
#15425=CARTESIAN_POINT ( 'NONE',  ( -56.49999999999997868, 2.944486372867092250, 1.699999999999810774 ) ) ;
#15445=CARTESIAN_POINT ( 'NONE',  ( -58.64405989232411542, 2.944486372867106461, -1.700000000000195577 ) ) ;
#15469=EDGE_LOOP ( 'NONE', ( #23380, #24428, #30571 ) ) ;
#15470=EDGE_CURVE ( 'NONE', #18483, #24201, #19052, .T. ) ;
#15475=ORIENTED_EDGE ( 'NONE', *, *, #11583, .T. ) ;
#15493=VECTOR ( 'NONE', #10848, 1000.000000000000000 ) ;
#15498=VECTOR ( 'NONE', #14251, 1000.000000000000000 ) ;
#15499=CARTESIAN_POINT ( 'NONE',  ( -56.32202994616206126, 2.078460969082643217, 3.599999999999808686 ) ) ;
#15504=CARTESIAN_POINT ( 'NONE',  ( -59.19999999999997442, 2.449420067797480893, 1.250136525132548693 ) ) ;
#15508=CARTESIAN_POINT ( 'NONE',  ( -59.10126175456193209, 2.465973215726302570, -0.9703132803711642662 ) ) ;
#15516=EDGE_CURVE ( 'NONE', #13230, #11849, #1329, .T. ) ;
#15520=CARTESIAN_POINT ( 'NONE',  ( -56.38452994616205416, 3.117691453623979481, 1.799999999999811751 ) ) ;
#15540=CIRCLE ( 'NONE', #28193, 0.09999999999999983902 ) ;
#15568=CARTESIAN_POINT ( 'NONE',  ( -59.50952994616202574, 3.117691453623994580, -1.800000000000197664 ) ) ;
#15569=ORIENTED_EDGE ( 'NONE', *, *, #14484, .T. ) ;
#15575=CARTESIAN_POINT ( 'NONE',  ( -56.37499999999998579, -3.920666489018338045E-15, 3.399999999999799183 ) ) ;
#15594=EDGE_CURVE ( 'NONE', #24984, #11667, #23095, .T. ) ;
#15598=CARTESIAN_POINT ( 'NONE',  ( -57.56249999999995737, -1.962990915244707368, -3.400000000000210854 ) ) ;
#15599=FACE_OUTER_BOUND ( 'NONE', #2480, .T. ) ;
#15614=ADVANCED_FACE ( 'NONE', ( #1769 ), #6227, .T. ) ;
#15617=CARTESIAN_POINT ( 'NONE',  ( -57.89405989232411542, 2.944486372867106461, -1.700000000000192912 ) ) ;
#15622=CARTESIAN_POINT ( 'NONE',  ( -59.18789508915042319, 2.395752775956333291, 1.250136525132548915 ) ) ;
#15633=CARTESIAN_POINT ( 'NONE',  ( -59.39405989232410832, 2.944486372867118451, -1.700000000000178035 ) ) ;
#15635=EDGE_CURVE ( 'NONE', #11459, #15281, #14468, .T. ) ;
#15638=CARTESIAN_POINT ( 'NONE',  ( -54.49999999999999289, 1.499999999999998002, 3.363870538531246623 ) ) ;
#15641=EDGE_LOOP ( 'NONE', ( #19803, #30303, #13888, #5603, #23165, #15475, #2109, #14162, #15237 ) ) ;
#15648=EDGE_LOOP ( 'NONE', ( #6602, #10041, #23360, #20720 ) ) ;
#15650=CARTESIAN_POINT ( 'NONE',  ( -54.58155989232413674, -1.962990915244731571, 3.399999999999796962 ) ) ;
#15651=MECHANICAL_DESIGN_GEOMETRIC_PRESENTATION_REPRESENTATION('',(#24744),#21226);
#15653=FACE_OUTER_BOUND ( 'NONE', #4597, .T. ) ;
#15660=AXIS2_PLACEMENT_3D ( 'NONE', #9502, #23747, #1560 ) ;
#15663=CARTESIAN_POINT ( 'NONE',  ( -58.82202994616202574, 2.078460969082688514, -3.600000000000191935 ) ) ;
#15672=CARTESIAN_POINT ( 'NONE',  ( -54.39999999999999147, -1.514093959731547701, 3.183260039818139653 ) ) ;
#15674=DIRECTION ( 'NONE',  ( 0.000000000000000000, -1.000000000000000000, -3.491481338843137694E-15 ) ) ;
#15688=DIRECTION ( 'NONE',  ( 1.344447539785323523E-44, -1.000000000000000000, -3.491481338843137300E-15 ) ) ;
#15694=B_SPLINE_CURVE_WITH_KNOTS ( 'NONE', 3,
 ( #27817, #20707, #30335, #31117, #28437, #4674, #7070, #14178, #19114, #2302, #11504, #31283, #16733, #21806, #18795, #9447 ),
 .UNSPECIFIED., .F., .F.,
 ( 4, 3, 3, 3, 3, 4 ),
 ( 0.000000000000000000, 3.448798496382319379E-05, 6.876885415380709437E-05, 0.0001064608974028143388, 0.0001221728072927708356, 0.0001243510251068951895 ),
 .UNSPECIFIED. ) ;
#15700=CARTESIAN_POINT ( 'NONE',  ( -59.50499785763158656, 3.022972365879558421, 1.564058272419715179 ) ) ;
#15705=DIRECTION ( 'NONE',  ( -1.000000000000000000, 1.219044193948983948E-29, -3.491481338843133355E-15 ) ) ;
#15709=VERTEX_POINT ( 'NONE', #14439 ) ;
#15720=CARTESIAN_POINT ( 'NONE',  ( -55.88452994616203995, 2.269957418536587429E-14, -3.600000000000198597 ) ) ;
#15721=CARTESIAN_POINT ( 'NONE',  ( -56.70655989232412253, -3.925981830489445379, -2.155497846303743205E-13 ) ) ;
#15726=CARTESIAN_POINT ( 'NONE',  ( -59.06249999999995737, -1.962990915244707368, -3.400000000000216627 ) ) ;
#15730=CARTESIAN_POINT ( 'NONE',  ( -54.49999999999997868, -1.697688561373014160, -3.084438062315841833 ) ) ;
#15736=CARTESIAN_POINT ( 'NONE',  ( -59.69985929041246209, 2.111923219456912193, 1.749892808977832726 ) ) ;
#15746=CARTESIAN_POINT ( 'NONE',  ( -55.24999999999996447, 2.023778652682505581E-14, -3.400000000000196643 ) ) ;
#15749=ORIENTED_EDGE ( 'NONE', *, *, #31318, .F. ) ;
#15750=DIRECTION ( 'NONE',  ( -1.499696682456171183E-15, -0.9030524935654884455, 0.4295302013422959697 ) ) ;
#15751=CIRCLE ( 'NONE', #13204, 3.525000000000025224 ) ;
#15752=ORIENTED_EDGE ( 'NONE', *, *, #3336, .F. ) ;
#15762=CARTESIAN_POINT ( 'NONE',  ( -60.45655989232412253, -3.925981830489445379, -2.286428396510360233E-13 ) ) ;
#15768=DIRECTION ( 'NONE',  ( -3.170125418975226039E-16, 0.9428090415820620240, 0.3333333333333372561 ) ) ;
#15772=LINE ( 'NONE', #7212, #21144 ) ;
#15777=ORIENTED_EDGE ( 'NONE', *, *, #29676, .T. ) ;
#15784=CARTESIAN_POINT ( 'NONE',  ( -44.49999999999997868, 8.366749974758269874E-15, -1.589829192029513996E-13 ) ) ;
#15790=CARTESIAN_POINT ( 'NONE',  ( -59.35358983848620795, 2.308634493194285486, 1.301040651491357503 ) ) ;
#15796=CARTESIAN_POINT ( 'NONE',  ( -44.59999999999998721, 1.557046979865768677, 3.273565289174733106 ) ) ;
#15797=FACE_OUTER_BOUND ( 'NONE', #14105, .T. ) ;
#15803=EDGE_CURVE ( 'NONE', #28731, #17704, #6934, .T. ) ;
#15811=VERTEX_POINT ( 'NONE', #11914 ) ;
#15829=CARTESIAN_POINT ( 'NONE',  ( -60.82202994616204705, 2.078460969082646770, 3.599999999999791367 ) ) ;
#15835=CARTESIAN_POINT ( 'NONE',  ( -54.68749999999998579, -3.399999999999991029, -2.060885718922576431E-13 ) ) ;
#15841=DIRECTION ( 'NONE',  ( 0.000000000000000000, -1.000000000000000000, -3.491481338843135722E-15 ) ) ;
#15842=ORIENTED_EDGE ( 'NONE', *, *, #15594, .F. ) ;
#15858=SURFACE_SIDE_STYLE ('',( #13628 ) ) ;
#15861=CARTESIAN_POINT ( 'NONE',  ( -55.83155989232411542, -1.962990915244706924, -3.400000000000204636 ) ) ;
#15868=CARTESIAN_POINT ( 'NONE',  ( -55.81249999999997158, 3.925981830489463142, -1.840516183884902743E-13 ) ) ;
#15871=CYLINDRICAL_SURFACE ( 'NONE', #9966, 0.1000000000000000472 ) ;
#15886=CARTESIAN_POINT ( 'NONE',  ( -54.93749999999998579, 1.962990915244722689, 3.399999999999812506 ) ) ;
#15899=DIRECTION ( 'NONE',  ( -1.000000000000000000, 1.219044193948983948E-29, -3.491481338843133355E-15 ) ) ;
#15902=VECTOR ( 'NONE', #5659, 1000.000000000000000 ) ;
#15915=ORIENTED_EDGE ( 'NONE', *, *, #45, .T. ) ;
#15934=DIRECTION ( 'NONE',  ( -1.000000000000000000, -0.000000000000000000, 0.000000000000000000 ) ) ;
#15942=CARTESIAN_POINT ( 'NONE',  ( -56.63452994616203284, 2.093608279459369510E-14, -3.600000000000201261 ) ) ;
#15957=CARTESIAN_POINT ( 'NONE',  ( -44.59999999999998010, -2.649999999999991918, -1.685844928847700321E-13 ) ) ;
#15960=DIRECTION ( 'NONE',  ( 1.000000000000000000, -1.219044193948983948E-29, 3.491481338843133355E-15 ) ) ;
#15973=AXIS2_PLACEMENT_3D ( 'NONE', #20385, #30173, #30007 ) ;
#15984=CARTESIAN_POINT ( 'NONE',  ( -54.49999999999999289, 1.499999999999995781, 4.029888335921750553 ) ) ;
#15986=CARTESIAN_POINT ( 'NONE',  ( -59.35162536475819905, 3.281785115337339409, 1.250136525132572451 ) ) ;
#15987=FACE_OUTER_BOUND ( 'NONE', #25007, .T. ) ;
#15992=DIRECTION ( 'NONE',  ( 1.000000000000000000, -1.219044193948983948E-29, 3.491481338843133355E-15 ) ) ;
#16014=AXIS2_PLACEMENT_3D ( 'NONE', #23586, #16626, #6638 ) ;
#16023=CARTESIAN_POINT ( 'NONE',  ( -58.08155989232410832, -1.962990915244706924, -3.400000000000212630 ) ) ;
#16031=CARTESIAN_POINT ( 'NONE',  ( -56.74999999999995737, 2.023778652682507474E-14, -3.400000000000201972 ) ) ;
#16040=VECTOR ( 'NONE', #16044, 1000.000000000000000 ) ;
#16044=DIRECTION ( 'NONE',  ( 3.491481338843133355E-15, 3.491481338843133355E-15, -1.000000000000000000 ) ) ;
#16045=EDGE_CURVE ( 'NONE', #30038, #2131, #22835, .T. ) ;
#16047=CARTESIAN_POINT ( 'NONE',  ( -59.67203891626250112, -2.203043321329347215, 1.525444001725758447 ) ) ;
#16049=CARTESIAN_POINT ( 'NONE',  ( -59.52340461522653925, 2.130728629699490284, 1.584472915547397776 ) ) ;
#16058=VECTOR ( 'NONE', #9280, 1000.000000000000000 ) ;
#16062=CARTESIAN_POINT ( 'NONE',  ( -57.99999999999997868, 2.944486372867092250, 1.699999999999805667 ) ) ;
#16069=VERTEX_POINT ( 'NONE', #8400 ) ;
#16075=VERTEX_POINT ( 'NONE', #27728 ) ;
#16079=APPLICATION_CONTEXT ( 'automotive_design' ) ;
#16115=VERTEX_POINT ( 'NONE', #25561 ) ;
#16120=CARTESIAN_POINT ( 'NONE',  ( -58.69702994616204705, 4.156921938165313080, -1.932741547809596393E-13 ) ) ;
#16127=CARTESIAN_POINT ( 'NONE',  ( -55.95655989232413674, -3.399999999999990585, -2.144552914728849520E-13 ) ) ;
#16135=CYLINDRICAL_SURFACE ( 'NONE', #25644, 3.399999999999999911 ) ;
#16136=CARTESIAN_POINT ( 'NONE',  ( -59.51024032614731851, 3.088598804228899652, 1.421463128792039843 ) ) ;
#16143=CARTESIAN_POINT ( 'NONE',  ( -59.94702994616205416, -2.078460969082657872, 3.599999999999778932 ) ) ;
#16151=TOROIDAL_SURFACE ( 'NONE', #2995, 3.525000000000025224, 0.1000000000000000056 ) ;
#16155=CARTESIAN_POINT ( 'NONE',  ( -59.34124040948578482, 3.262940601168114796, 1.250136525132572451 ) ) ;
#16180=PLANE ( 'NONE',  #7336 ) ;
#16184=( NAMED_UNIT ( * ) SI_UNIT ( $, .STERADIAN. ) SOLID_ANGLE_UNIT ( ) );
#16185=CARTESIAN_POINT ( 'NONE',  ( -55.07202994616204705, 2.078460969082675192, -3.600000000000186606 ) ) ;
#16187=CARTESIAN_POINT ( 'NONE',  ( -58.33155989232413674, -1.962990915244731571, 3.399999999999784528 ) ) ;
#16192=ORIENTED_EDGE ( 'NONE', *, *, #21764, .F. ) ;
#16194=CARTESIAN_POINT ( 'NONE',  ( -55.69702994616204705, 4.156921938165313080, -1.827997107644302771E-13 ) ) ;
#16195=CARTESIAN_POINT ( 'NONE',  ( -55.01905989232411542, 2.107054635024524725E-14, -3.400000000000195310 ) ) ;
#16201=CARTESIAN_POINT ( 'NONE',  ( -44.59999999999997300, 8.366749974758367693E-15, -1.870876429524646202E-13 ) ) ;
#16219=CARTESIAN_POINT ( 'NONE',  ( -55.38452994616205416, -3.117691453623976816, 1.799999999999791100 ) ) ;
#16227=DIRECTION ( 'NONE',  ( 1.000000000000000000, -1.219044193948983948E-29, 3.491481338843133355E-15 ) ) ;
#16235=CARTESIAN_POINT ( 'NONE',  ( -55.81249999999997868, 3.400000000000007905, -1.865662262041272555E-13 ) ) ;
#16245=EDGE_CURVE ( 'NONE', #14659, #2157, #28603, .T. ) ;
#16246=DIRECTION ( 'NONE',  ( 1.000000000000000000, -1.219044193948983948E-29, 3.491481338843133355E-15 ) ) ;
#16251=ORIENTED_EDGE ( 'NONE', *, *, #30024, .T. ) ;
#16253=ORIENTED_EDGE ( 'NONE', *, *, #18427, .F. ) ;
#16256=DIRECTION ( 'NONE',  ( -1.000000000000000000, 1.219044193948983948E-29, -3.491481338843133355E-15 ) ) ;
#16262=FACE_OUTER_BOUND ( 'NONE', #19212, .T. ) ;
#16273=CARTESIAN_POINT ( 'NONE',  ( -54.49999999999996447, 2.023778652682504319E-14, -3.400000000000193978 ) ) ;
#16274=ADVANCED_FACE ( 'NONE', ( #21636 ), #17481, .T. ) ;
#16275=CARTESIAN_POINT ( 'NONE',  ( -57.07202994616206126, 2.078460969082646770, 3.599999999999804690 ) ) ;
#16276=CARTESIAN_POINT ( 'NONE',  ( -59.17366934936939060, -2.509710670695419754, -0.9445351920416235059 ) ) ;
#16282=EDGE_CURVE ( 'NONE', #15709, #7802, #24155, .T. ) ;
#16283=( BOUNDED_CURVE ( )  B_SPLINE_CURVE ( 2, ( #13406, #6476, #4090, #23416, #21219, #30515, #1697, #11365, #18213 ),
 .UNSPECIFIED., .F., .T. ) 
 B_SPLINE_CURVE_WITH_KNOTS ( ( 3, 2, 2, 2, 3 ),
 ( 0.3611111111111111605, 0.3703703703703703498, 0.3888888888888888951, 0.4074074074074073848, 0.4166666666666666852 ),
 .UNSPECIFIED. ) 
 CURVE ( )  GEOMETRIC_REPRESENTATION_ITEM ( )  RATIONAL_B_SPLINE_CURVE ( ( 0.9330127018922194093, 0.9330127018922197424, 1.000000000000000000, 0.8660254037844387076, 1.000000000000000000, 0.8660254037844387076, 1.000000000000000000, 0.9330127018922191873, 0.9330127018922194093 ) ) 
 REPRESENTATION_ITEM ( '' )  );
#16287=CARTESIAN_POINT ( 'NONE',  ( -59.48573950359912743, 3.423031164920794289, -1.114835254188495162 ) ) ;
#16289=DIRECTION ( 'NONE',  ( 0.000000000000000000, -1.000000000000000000, 0.000000000000000000 ) ) ;
#16297=ORIENTED_EDGE ( 'NONE', *, *, #30915, .T. ) ;
#16308=SPHERICAL_SURFACE ( 'NONE', #2290, 0.1000000000000000056 ) ;
#16339=( LENGTH_UNIT ( ) NAMED_UNIT ( * ) SI_UNIT ( .MILLI., .METRE. ) );
#16341=CARTESIAN_POINT ( 'NONE',  ( -56.51905989232411542, 2.023778652682506843E-14, -3.400000000000200640 ) ) ;
#16345=CARTESIAN_POINT ( 'NONE',  ( -55.44702994616206126, -2.078460969082657872, 3.599999999999794920 ) ) ;
#16362=DIRECTION ( 'NONE',  ( 0.000000000000000000, -1.000000000000000000, 0.000000000000000000 ) ) ;
#16369=CARTESIAN_POINT ( 'NONE',  ( -60.18749999999998579, 1.962990915244722689, 3.399999999999794742 ) ) ;
#16373=ORIENTED_EDGE ( 'NONE', *, *, #5356, .F. ) ;
#16378=CARTESIAN_POINT ( 'NONE',  ( -59.69999999999997442, -3.399999999999991473, -2.235080921937235780E-13 ) ) ;
#16391=DIRECTION ( 'NONE',  ( 2.114027855662425118E-44, -1.000000000000000000, -3.491481338843139666E-15 ) ) ;
#16399=EDGE_CURVE ( 'NONE', #13704, #6992, #20019, .T. ) ;
#16414=EDGE_CURVE ( 'NONE', #556, #13873, #6352, .T. ) ;
#16416=AXIS2_PLACEMENT_3D ( 'NONE', #12137, #31127, #14660 ) ;
#16418=EDGE_CURVE ( 'NONE', #7185, #16500, #10844, .T. ) ;
#16422=CARTESIAN_POINT ( 'NONE',  ( -57.69702994616206126, -2.078460969082657872, 3.599999999999786926 ) ) ;
#16433=CARTESIAN_POINT ( 'NONE',  ( -54.39999999999999147, -1.557046979865776226, 3.273565289174688253 ) ) ;
#16438=CARTESIAN_POINT ( 'NONE',  ( -54.49999999999999289, -1.500000000000006661, 3.959797974644449603 ) ) ;
#16446=CARTESIAN_POINT ( 'NONE',  ( -59.33448904220814057, -2.516908228110002366, -1.027510759589413736 ) ) ;
#16454=CARTESIAN_POINT ( 'NONE',  ( -55.33155989232414385, -1.962990915244735790, 3.399999999999792522 ) ) ;
#16466=DIRECTION ( 'NONE',  ( 1.000000000000000000, -1.219044193948983948E-29, 3.491481338843133355E-15 ) ) ;
#16470=AXIS2_PLACEMENT_3D ( 'NONE', #1690, #6769, #4398 ) ;
#16475=AXIS2_PLACEMENT_3D ( 'NONE', #24372, #12042, #14853 ) ;
#16489=VERTEX_POINT ( 'NONE', #9430 ) ;
#16499=DIRECTION ( 'NONE',  ( 0.000000000000000000, -1.000000000000000000, -4.336808689942015369E-15 ) ) ;
#16500=VERTEX_POINT ( 'NONE', #7059 ) ;
#16502=ORIENTED_EDGE ( 'NONE', *, *, #4399, .F. ) ;
#16505=CARTESIAN_POINT ( 'NONE',  ( -60.24999999999997158, 2.944486372867092250, 1.699999999999797673 ) ) ;
#16510=DIRECTION ( 'NONE',  ( 1.163827112947710658E-15, 0.9428090415820645775, -0.3333333333333299286 ) ) ;
#16530=AXIS2_PLACEMENT_3D ( 'NONE', #13764, #1274, #25819 ) ;
#16535=CARTESIAN_POINT ( 'NONE',  ( -59.68749999999995737, 1.962990915244749557, -3.400000000000203304 ) ) ;
#16544=CARTESIAN_POINT ( 'NONE',  ( -57.69702994616206126, -2.078460969082657872, 3.599999999999786926 ) ) ;
#16551=VERTEX_POINT ( 'NONE', #9599 ) ;
#16553=B_SPLINE_CURVE_WITH_KNOTS ( 'NONE', 3,
 ( #8102, #17770, #27410, #25021, #3352, #13002, #30086, #6506, #6659, #6991, #4271, #4122, #26295, #31202, #16653, #7142 ),
 .UNSPECIFIED., .F., .F.,
 ( 4, 3, 3, 3, 3, 4 ),
 ( 0.000000000000000000, 3.350201058276301074E-05, 6.696995785605353631E-05, 0.0001009523001788503553, 0.0001220103457549332620, 0.0001251189910046208303 ),
 .UNSPECIFIED. ) ;
#16569=ADVANCED_FACE ( 'NONE', ( #28747 ), #19506, .T. ) ;
#16582=VECTOR ( 'NONE', #22158, 1000.000000000000000 ) ;
#16588=DIRECTION ( 'NONE',  ( 0.000000000000000000, -1.000000000000000000, -3.491481338843133355E-15 ) ) ;
#16596=FACE_OUTER_BOUND ( 'NONE', #4718, .T. ) ;
#16599=CARTESIAN_POINT ( 'NONE',  ( -58.94702994616203284, -2.078460969082631227, -3.600000000000215472 ) ) ;
#16626=DIRECTION ( 'NONE',  ( 3.491481338843133355E-15, 3.491481338843133355E-15, -1.000000000000000000 ) ) ;
#16631=CIRCLE ( 'NONE', #8022, 0.1000000000000001166 ) ;
#16640=EDGE_CURVE ( 'NONE', #27693, #18790, #11755, .T. ) ;
#16653=CARTESIAN_POINT ( 'NONE',  ( -59.60101405528192942, 2.022629942802355973, 1.712153077242869470 ) ) ;
#16655=VECTOR ( 'NONE', #31074, 1000.000000000000000 ) ;
#16673=ADVANCED_FACE ( 'NONE', ( #4187 ), #13825, .T. ) ;
#16676=EDGE_CURVE ( 'NONE', #1750, #13697, #17483, .T. ) ;
#16678=CARTESIAN_POINT ( 'NONE',  ( -55.07202994616204705, 2.078460969082674747, -3.600000000000187494 ) ) ;
#16692=DIRECTION ( 'NONE',  ( 1.000000000000000000, -1.219044193948983948E-29, 3.491481338843133355E-15 ) ) ;
#16702=CARTESIAN_POINT ( 'NONE',  ( -55.44702994616206126, -2.078460969082657872, 3.599999999999794920 ) ) ;
#16704=ORIENTED_EDGE ( 'NONE', *, *, #30959, .F. ) ;
#16709=CARTESIAN_POINT ( 'NONE',  ( -56.38452994616205416, 3.117691453623979481, 1.799999999999811751 ) ) ;
#16729=DIRECTION ( 'NONE',  ( 3.491481338843133355E-15, 3.491481338843133355E-15, -1.000000000000000000 ) ) ;
#16733=CARTESIAN_POINT ( 'NONE',  ( -59.10192033946857748, -2.331623134809623465, 1.259417044000318286 ) ) ;
#16740=ORIENTED_EDGE ( 'NONE', *, *, #5001, .F. ) ;
#16752=CARTESIAN_POINT ( 'NONE',  ( -59.51024032614731851, 3.088598804228899652, 1.421463128792039843 ) ) ;
#16753=CARTESIAN_POINT ( 'NONE',  ( -56.20655989232413674, 1.962990915244722245, 3.399999999999807621 ) ) ;
#16754=CARTESIAN_POINT ( 'NONE',  ( -59.17998499521433331, -2.518779524791931124, -0.9443209727575352375 ) ) ;
#16773=EDGE_LOOP ( 'NONE', ( #19349, #13664, #26952, #3051, #9763, #9253 ) ) ;
#16780=DIRECTION ( 'NONE',  ( 3.491481338843133355E-15, 3.491481338843133355E-15, -1.000000000000000000 ) ) ;
#16798=CARTESIAN_POINT ( 'NONE',  ( -59.13463329438567229, 2.488830503680618200, -0.9121239897849973133 ) ) ;
#16799=CARTESIAN_POINT ( 'NONE',  ( -59.46420457061498865, 3.387909745995675959, -1.102402054833139466 ) ) ;
#16802=CARTESIAN_POINT ( 'NONE',  ( -44.59999999999998721, 1.499999999999998002, 3.363870538531281262 ) ) ;
#16812=EDGE_CURVE ( 'NONE', #17785, #5500, #1112, .T. ) ;
#16815=CARTESIAN_POINT ( 'NONE',  ( -59.69999999999998153, 2.336591249775839430, 1.750136525132547360 ) ) ;
#16819=( BOUNDED_CURVE ( )  B_SPLINE_CURVE ( 2, ( #24218, #29274, #2676, #2530, #29113, #24505, #12179, #12314, #21999 ),
 .UNSPECIFIED., .F., .T. ) 
 B_SPLINE_CURVE_WITH_KNOTS ( ( 3, 2, 2, 2, 3 ),
 ( 0.08333333333333332871, 0.09259259259259258745, 0.1111111111111111049, 0.1296296296296296224, 0.1388888888888888951 ),
 .UNSPECIFIED. ) 
 CURVE ( )  GEOMETRIC_REPRESENTATION_ITEM ( )  RATIONAL_B_SPLINE_CURVE ( ( 0.9330127018922194093, 0.9330127018922194093, 1.000000000000000000, 0.8660254037844387076, 1.000000000000000000, 0.8660254037844387076, 1.000000000000000000, 0.9330127018922191873, 0.9330127018922192983 ) ) 
 REPRESENTATION_ITEM ( '' )  );
#16820=DIRECTION ( 'NONE',  ( 1.000000000000000000, -1.219044193948983948E-29, 3.491481338843133355E-15 ) ) ;
#16822=CARTESIAN_POINT ( 'NONE',  ( -59.69999999999997442, -3.237160264815294841, -1.238538609462289219 ) ) ;
#16824=CARTESIAN_POINT ( 'NONE',  ( -60.70655989232412963, 1.962990915244722245, 3.399999999999792077 ) ) ;
#16825=ORIENTED_EDGE ( 'NONE', *, *, #9634, .F. ) ;
#16830=CARTESIAN_POINT ( 'NONE',  ( -55.25952994616203995, -3.117691453623963938, -1.800000000000207434 ) ) ;
#16836=DIRECTION ( 'NONE',  ( 0.000000000000000000, 1.000000000000000000, 4.336808689942015369E-15 ) ) ;
#16855=CARTESIAN_POINT ( 'NONE',  ( -55.07202994616204705, 2.078460969082674747, -3.600000000000187494 ) ) ;
#16856=VERTEX_POINT ( 'NONE', #13487 ) ;
#16860=CARTESIAN_POINT ( 'NONE',  ( -54.49999999999996447, -1.499999999999981126, -3.363870538531692045 ) ) ;
#16861=CARTESIAN_POINT ( 'NONE',  ( -55.82202994616203995, 2.078460969082674747, -3.600000000000189715 ) ) ;
#16871=CARTESIAN_POINT ( 'NONE',  ( -59.19999999999996732, -3.264622394567714192, -0.9498634748674711359 ) ) ;
#16880=EDGE_CURVE ( 'NONE', #4682, #17943, #22577, .T. ) ;
#16882=DIRECTION ( 'NONE',  ( -1.000000000000000000, 1.219044193948983948E-29, -3.491481338843133355E-15 ) ) ;
#16901=CARTESIAN_POINT ( 'NONE',  ( -54.39405989232412253, -2.944486372867076263, -1.700000000000203793 ) ) ;
#16904=CARTESIAN_POINT ( 'NONE',  ( -44.59999999999998010, 2.750000000000007994, -1.493937157852515840E-13 ) ) ;
#16920=CARTESIAN_POINT ( 'NONE',  ( -57.56249999999995737, -1.962990915244702039, -3.400000000000213962 ) ) ;
#16927=ORIENTED_EDGE ( 'NONE', *, *, #25707, .F. ) ;
#16929=AXIS2_PLACEMENT_3D ( 'NONE', #20835, #14165, #26205 ) ;
#16934=CARTESIAN_POINT ( 'NONE',  ( -59.51260631243411581, 2.329131096718564553, 1.425561137250796362 ) ) ;
#16953=ORIENTED_EDGE ( 'NONE', *, *, #16245, .T. ) ;
#16955=DIRECTION ( 'NONE',  ( -1.000000000000000000, 1.219044193948984088E-29, -3.491481338843133750E-15 ) ) ;
#16957=DIRECTION ( 'NONE',  ( 1.000000000000000000, -1.219044193948983948E-29, 3.491481338843133355E-15 ) ) ;
#16962=ORIENTED_EDGE ( 'NONE', *, *, #25707, .T. ) ;
#16970=VERTEX_POINT ( 'NONE', #13950 ) ;
#16974=CARTESIAN_POINT ( 'NONE',  ( -59.95655989232412963, 1.962990915244722245, 3.399999999999794742 ) ) ;
#16977=EDGE_LOOP ( 'NONE', ( #30605, #4927, #11788, #27579 ) ) ;
#16978=B_SPLINE_CURVE_WITH_KNOTS ( 'NONE', 3,
 ( #28143, #2020, #11683, #21362 ),
 .UNSPECIFIED., .F., .F.,
 ( 4, 4 ),
 ( 1.045245121249583768E-16, 0.0009258403723363874561 ),
 .UNSPECIFIED. ) ;
#16980=CARTESIAN_POINT ( 'NONE',  ( -57.19702994616204705, 4.156921938165313080, -1.880369327726949834E-13 ) ) ;
#16998=TOROIDAL_SURFACE ( 'NONE', #27073, 2.750000000000000000, 0.1000000000000000056 ) ;
#17009=CARTESIAN_POINT ( 'NONE',  ( -56.94702994616206126, -2.078460969082657872, 3.599999999999789591 ) ) ;
#17013=CARTESIAN_POINT ( 'NONE',  ( -59.60604010435355349, 3.187076279294280390, -1.184290838417780600 ) ) ;
#17017=CARTESIAN_POINT ( 'NONE',  ( -55.94702994616203995, -2.078460969082631227, -3.600000000000205258 ) ) ;
#17033=ADVANCED_FACE ( 'NONE', ( #4473 ), #22056, .T. ) ;
#17056=ORIENTED_EDGE ( 'NONE', *, *, #15083, .T. ) ;
#17058=VERTEX_POINT ( 'NONE', #4622 ) ;
#17059=CARTESIAN_POINT ( 'NONE',  ( -44.59999999999999432, 1.433333333333330906, 4.054078878802660491 ) ) ;
#17061=DIRECTION ( 'NONE',  ( 0.000000000000000000, 1.000000000000000000, -8.673617379884030739E-15 ) ) ;
#17067=CARTESIAN_POINT ( 'NONE',  ( -60.38452994616202574, 2.093608279459374244E-14, -3.600000000000214140 ) ) ;
#17076=CYLINDRICAL_SURFACE ( 'NONE', #10423, 4.299999999999954525 ) ;
#17084=EDGE_LOOP ( 'NONE', ( #24883, #10242, #8616, #13677 ) ) ;
#17093=DIRECTION ( 'NONE',  ( 0.000000000000000000, -1.000000000000000000, -3.491481338843132961E-15 ) ) ;
#17108=ORIENTED_EDGE ( 'NONE', *, *, #25233, .T. ) ;
#17114=DIRECTION ( 'NONE',  ( -1.344447539785323523E-44, 1.000000000000000000, 3.491481338843137300E-15 ) ) ;
#17115=CARTESIAN_POINT ( 'NONE',  ( -59.44266919280509143, 3.352788690741696609, -1.089968598657499177 ) ) ;
#17124=DIRECTION ( 'NONE',  ( 0.000000000000000000, -1.000000000000000000, 0.000000000000000000 ) ) ;
#17127=VERTEX_POINT ( 'NONE', #3998 ) ;
#17132=ORIENTED_EDGE ( 'NONE', *, *, #20695, .T. ) ;
#17135=ORIENTED_EDGE ( 'NONE', *, *, #11497, .F. ) ;
#17142=CARTESIAN_POINT ( 'NONE',  ( -59.75952994616203284, -3.117691453623963938, -1.800000000000223199 ) ) ;
#17160=CARTESIAN_POINT ( 'NONE',  ( -58.06249999999996447, 3.400000000000007905, -1.844164440896605116E-13 ) ) ;
#17164=DIRECTION ( 'NONE',  ( 0.000000000000000000, 1.000000000000000000, 3.491481338843130594E-15 ) ) ;
#17171=DIRECTION ( 'NONE',  ( -1.000000000000000000, 1.219044193948983948E-29, -3.491481338843133355E-15 ) ) ;
#17173=CARTESIAN_POINT ( 'NONE',  ( -57.38452994616203284, 2.093608279459370457E-14, -3.600000000000203926 ) ) ;
#17174=ORIENTED_EDGE ( 'NONE', *, *, #14323, .T. ) ;
#17176=LINE ( 'NONE', #7347, #8121 ) ;
#17189=CARTESIAN_POINT ( 'NONE',  ( -59.66878239164782372, 3.173439364805089813, -1.220515114876693064 ) ) ;
#17201=VERTEX_POINT ( 'NONE', #495 ) ;
#17207=ORIENTED_EDGE ( 'NONE', *, *, #25272, .T. ) ;
#17214=AXIS2_PLACEMENT_3D ( 'NONE', #18452, #15899, #12109 ) ;
#17215=CARTESIAN_POINT ( 'NONE',  ( -55.26905989232413674, -2.944486372867088697, 1.699999999999792344 ) ) ;
#17230=CYLINDRICAL_SURFACE ( 'NONE', #11709, 3.399999999999999911 ) ;
#17242=EDGE_CURVE ( 'NONE', #29758, #30573, #1820, .T. ) ;
#17246=CARTESIAN_POINT ( 'NONE',  ( -55.81249999999997868, 3.400000000000007905, -1.865662262041272555E-13 ) ) ;
#17266=ORIENTED_EDGE ( 'NONE', *, *, #11136, .F. ) ;
#17273=ORIENTED_EDGE ( 'NONE', *, *, #2549, .F. ) ;
#17283=CARTESIAN_POINT ( 'NONE',  ( -58.75952994616203284, 3.117691453623994580, -1.800000000000195000 ) ) ;
#17290=CARTESIAN_POINT ( 'NONE',  ( -59.69999999999998153, -3.031840806488110385, 1.538811659727342906 ) ) ;
#17293=DIRECTION ( 'NONE',  ( 0.000000000000000000, -1.000000000000000000, -2.168404344971007685E-15 ) ) ;
#17303=EDGE_LOOP ( 'NONE', ( #6342, #13781, #30337, #13588 ) ) ;
#17305=ADVANCED_FACE ( 'NONE', ( #8393 ), #22503, .T. ) ;
#17314=CARTESIAN_POINT ( 'NONE',  ( -55.01905989232411542, 2.023778652682504950E-14, -3.400000000000195310 ) ) ;
#17325=DIRECTION ( 'NONE',  ( -1.404304041445553711E-15, -0.9030524935654961061, 0.4295302013422803711 ) ) ;
#17329=DIRECTION ( 'NONE',  ( -1.000000000000000000, 1.219044193948983948E-29, -3.491481338843133355E-15 ) ) ;
#17337=CARTESIAN_POINT ( 'NONE',  ( -59.13147575765562181, 2.328089616296125985, 1.276504352643064388 ) ) ;
#17351=DIRECTION ( 'NONE',  ( -1.000000000000000000, 1.219044193948983948E-29, -3.491481338843133355E-15 ) ) ;
#17352=EDGE_CURVE ( 'NONE', #5493, #20519, #21560, .T. ) ;
#17354=CARTESIAN_POINT ( 'NONE',  ( -60.19702994616203995, 4.156921938165313080, -1.985113767892243204E-13 ) ) ;
#17359=ADVANCED_FACE ( 'NONE', ( #8695 ), #17996, .T. ) ;
#17380=CARTESIAN_POINT ( 'NONE',  ( -58.01905989232410832, 3.648081215184778998E-14, -3.400000000000205969 ) ) ;
#17381=CARTESIAN_POINT ( 'NONE',  ( -59.09999999999997300, 8.366749974758448157E-15, -2.099585467500611340E-13 ) ) ;
#17385=CARTESIAN_POINT ( 'NONE',  ( -58.06249999999996447, 3.400000000000007905, -1.844164440896605116E-13 ) ) ;
#17395=B_SPLINE_CURVE_WITH_KNOTS ( 'NONE', 3,
 ( #16822, #13625, #1597, #20936, #30567, #6523 ),
 .UNSPECIFIED., .F., .F.,
 ( 4, 2, 4 ),
 ( 0.001078866813306119657, 0.002246630675358731073, 0.003414394537411343140 ),
 .UNSPECIFIED. ) ;
#17397=EDGE_CURVE ( 'NONE', #26101, #7915, #7960, .T. ) ;
#17402=FACE_OUTER_BOUND ( 'NONE', #21655, .T. ) ;
#17427=ORIENTED_EDGE ( 'NONE', *, *, #18504, .F. ) ;
#17428=CARTESIAN_POINT ( 'NONE',  ( -56.50952994616203995, 3.117691453623994580, -1.800000000000187006 ) ) ;
#17435=ADVANCED_FACE ( 'NONE', ( #15987 ), #11234, .T. ) ;
#17464=CARTESIAN_POINT ( 'NONE',  ( -60.07202994616204705, 2.078460969082646770, 3.599999999999794031 ) ) ;
#17474=DIRECTION ( 'NONE',  ( -1.000000000000000000, -0.000000000000000000, 0.000000000000000000 ) ) ;
#17481=TOROIDAL_SURFACE ( 'NONE', #30095, 4.199999999999954881, 0.1000000000000000056 ) ;
#17483=( BOUNDED_CURVE ( )  B_SPLINE_CURVE ( 3, ( #16871, #21795, #24444, #387 ),
 .UNSPECIFIED., .F., .T. ) 
 B_SPLINE_CURVE_WITH_KNOTS ( ( 4, 4 ),
 ( 1.853935925778139149, 1.936702241689763682 ),
 .UNSPECIFIED. ) 
 CURVE ( )  GEOMETRIC_REPRESENTATION_ITEM ( )  RATIONAL_B_SPLINE_CURVE ( ( 1.000000000000000000, 0.9994292262101478475, 0.9994292262101478475, 1.000000000000000000 ) ) 
 REPRESENTATION_ITEM ( '' )  );
#17487=DIRECTION ( 'NONE',  ( 1.000000000000000000, -1.219044193948983948E-29, 3.491481338843133355E-15 ) ) ;
#17511=CARTESIAN_POINT ( 'NONE',  ( -57.08155989232412963, 3.400000000000007905, -1.873796572744660248E-13 ) ) ;
#17512=CARTESIAN_POINT ( 'NONE',  ( -59.12499999999996447, -2.944486372867072266, -1.700000000000227995 ) ) ;
#17513=AXIS2_PLACEMENT_3D ( 'NONE', #22704, #20788, #20173 ) ;
#17515=CARTESIAN_POINT ( 'NONE',  ( -60.14405989232410832, 2.944486372867106461, -1.700000000000200684 ) ) ;
#17546=CARTESIAN_POINT ( 'NONE',  ( -57.51905989232412963, -2.944486372867094470, 1.699999999999774802 ) ) ;
#17556=CARTESIAN_POINT ( 'NONE',  ( -54.70655989232413674, 1.962990915244722467, 3.399999999999812950 ) ) ;
#17566=ADVANCED_FACE ( 'NONE', ( #13073 ), #28104, .T. ) ;
#17573=CARTESIAN_POINT ( 'NONE',  ( -59.32202994616204705, 2.078460969082640108, 3.599999999999799805 ) ) ;
#17581=CARTESIAN_POINT ( 'NONE',  ( -59.12208601139542452, 2.471957471229930370, -0.9603292137297660958 ) ) ;
#17582=CARTESIAN_POINT ( 'NONE',  ( -54.49999999999997158, -2.083909216633824890, -2.852996025551205683 ) ) ;
#17589=CARTESIAN_POINT ( 'NONE',  ( -57.50952994616203995, -3.117691453623963938, -1.800000000000215206 ) ) ;
#17597=CIRCLE ( 'NONE', #12039, 0.09999999999999982514 ) ;
#17598=ADVANCED_FACE ( 'NONE', ( #13538 ), #3722, .T. ) ;
#17600=CARTESIAN_POINT ( 'NONE',  ( -59.00952994616203284, -3.117691453623963938, -1.800000000000220757 ) ) ;
#17601=CARTESIAN_POINT ( 'NONE',  ( -59.66183546925923764, -3.174920041538525251, -1.216504307364950854 ) ) ;
#17620=CARTESIAN_POINT ( 'NONE',  ( -58.43749999999997158, -3.399999999999991029, -2.253785087031484148E-13 ) ) ;
#17622=DIRECTION ( 'NONE',  ( 0.000000000000000000, 1.000000000000000000, 3.491481338843130594E-15 ) ) ;
#17624=B_SPLINE_CURVE_WITH_KNOTS ( 'NONE', 3,
 ( #28065, #6383, #16047, #25700, #20958, #19811, #24251, #9694, #24541, #29304, #7303, #7756, #32 ),
 .UNSPECIFIED., .F., .F.,
 ( 4, 3, 3, 3, 4 ),
 ( 3.529906531158615134E-18, 3.856107938921464966E-05, 7.311388640164024157E-05, 0.0001107339254823213112, 0.0001129379781057718247 ),
 .UNSPECIFIED. ) ;
#17625=VERTEX_POINT ( 'NONE', #13365 ) ;
#17634=CARTESIAN_POINT ( 'NONE',  ( -55.20655989232412963, -3.925981830489445379, -2.103125626221096647E-13 ) ) ;
#17636=FACE_OUTER_BOUND ( 'NONE', #27157, .T. ) ;
#17658=CARTESIAN_POINT ( 'NONE',  ( -59.69999999999997442, -2.455304892039217091, -1.238538609462283446 ) ) ;
#17681=CARTESIAN_POINT ( 'NONE',  ( -59.51905989232410121, 2.023778652682510314E-14, -3.400000000000210854 ) ) ;
#17685=AXIS2_PLACEMENT_3D ( 'NONE', #11099, #23304, #1587 ) ;
#17690=CARTESIAN_POINT ( 'NONE',  ( -59.33507117675159748, -2.361427661686895885, 1.328119905389837152 ) ) ;
#17691=DIRECTION ( 'NONE',  ( -7.637891338979715149E-45, -1.000000000000000000, -3.491481338843131383E-15 ) ) ;
#17692=ORIENTED_EDGE ( 'NONE', *, *, #9300, .F. ) ;
#17704=VERTEX_POINT ( 'NONE', #21174 ) ;
#17716=CARTESIAN_POINT ( 'NONE',  ( -54.57202994616205416, -4.156921938165296204, -2.089175772356712570E-13 ) ) ;
#17717=CARTESIAN_POINT ( 'NONE',  ( -56.15400635094608361, -3.399999999999987477, -0.9110272542660342587 ) ) ;
#17730=CARTESIAN_POINT ( 'NONE',  ( -57.82202994616204705, 2.078460969082641885, 3.599999999999803801 ) ) ;
#17733=CYLINDRICAL_SURFACE ( 'NONE', #13971, 0.1000000000000000472 ) ;
#17747=CARTESIAN_POINT ( 'NONE',  ( -57.82202994616206126, 2.078460969082646770, 3.599999999999802025 ) ) ;
#17748=CARTESIAN_POINT ( 'NONE',  ( -59.19162505689493514, 2.404119360129248761, 1.250136525132548693 ) ) ;
#17759=DIRECTION ( 'NONE',  ( 0.000000000000000000, -1.000000000000000000, -3.491481338843133355E-15 ) ) ;
#17761=CARTESIAN_POINT ( 'NONE',  ( -56.39405989232412253, 2.944486372867110013, -1.700000000000180922 ) ) ;
#17770=CARTESIAN_POINT ( 'NONE',  ( -59.69104130886936588, 2.078408370926939863, 1.734619616925012986 ) ) ;
#17779=CYLINDRICAL_SURFACE ( 'NONE', #5384, 3.399999999999999911 ) ;
#17785=VERTEX_POINT ( 'NONE', #7810 ) ;
#17793=CARTESIAN_POINT ( 'NONE',  ( -59.94702994616205416, -2.078460969082657872, 3.599999999999778932 ) ) ;
#17810=DIRECTION ( 'NONE',  ( 1.000000000000000000, -1.219044193948983948E-29, 3.491481338843133355E-15 ) ) ;
#17812=CARTESIAN_POINT ( 'NONE',  ( -59.69999999999998153, 2.121207708687718352, 1.750136525132546472 ) ) ;
#17816=ORIENTED_EDGE ( 'NONE', *, *, #8253, .F. ) ;
#17818=ORIENTED_EDGE ( 'NONE', *, *, #8253, .T. ) ;
#17819=ORIENTED_EDGE ( 'NONE', *, *, #9349, .F. ) ;
#17822=CARTESIAN_POINT ( 'NONE',  ( -55.37499999999996447, -2.944486372867076707, -1.700000000000207345 ) ) ;
#17823=CARTESIAN_POINT ( 'NONE',  ( -59.60820241427157384, 2.215761459564569602, 1.591138442638788453 ) ) ;
#17824=VERTEX_POINT ( 'NONE', #86 ) ;
#17829=ORIENTED_EDGE ( 'NONE', *, *, #12706, .T. ) ;
#17831=( BOUNDED_SURFACE ( )  B_SPLINE_SURFACE ( 1, 2, ( 
 ( #13393, #27839, #15175, #25300, #3298, #8662, #20265, #29894, #24827, #12784, #18030, #13247, #22462, #758, #10421, #20414, #20104, #29738, #30036, #5831, #8055, #17873, #27364, #27507, #8351, #21506, #13567, #9307, #26241, #14199, #4225, #25920, #19139, #31141, #2165, #6293, #15942, #20874, #4552, #28307, #6464, #23874, #3925, #16275, #9473, #14037, #8807, #25602, #23724, #21030, #23254, #4079, #11828, #16422, #28617, #1541, #9154, #13719, #28460, #6933, #23402, #23553, #11201, #26076, #2016, #18815, #21359, #30501, #6763, #16120, #11681, #28139, #1684, #16599, #18496, #4388, #30985, #25770, #18970, #11345, #13863, #30670, #8985, #1854, #6613, #18658, #11527, #21203, #30836, #569, #12596, #4696, #421, #17354, #5307, #26723, #17067, #10227, #22281, #24637, #28778, #7091, #11993, #27000, #19435, #28925, #14968, #26396, #7389 ),
 ( #21678, #7237, #16901, #259, #31301, #22129, #29081, #29384, #2785, #14812, #7696, #19755, #5013, #14674, #5163, #26544, #17215, #24334, #4851, #2641, #12436, #14518, #12283, #21970, #9633, #26857, #9923, #19603, #2951, #29241, #2493, #16753, #24186, #7555, #2326, #24474, #10079, #19290, #14350, #24020, #12148, #21826, #114, #9770, #27324, #891, #29525, #20225, #29853, #8167, #13358, #24791, #17985, #5482, #17836, #27634, #20059, #22588, #15617, #1045, #25258, #25096, #27470, #3577, #5790, #12749, #19896, #22897, #23050, #1342, #15445, #22749, #30000, #24935, #10695, #8313, #30161, #5963, #6111, #13215, #1186, #22425, #10843, #15134, #17681, #3098, #20378, #20528, #5636, #10548, #7839, #3428, #13066, #8480, #17515, #717, #18161, #10377, #27798, #15762, #29696, #25412, #3715, #27170, #8016, #15287, #3257, #12899, #28265 ) ),
 .UNSPECIFIED., .F., .F., .F. ) 
 B_SPLINE_SURFACE_WITH_KNOTS ( ( 2, 2 ),
 ( 3, 2, 2, 2, 2, 2, 2, 2, 2, 2, 2, 2, 2, 2, 2, 2, 2, 2, 2, 2, 2, 2, 2, 2, 2, 2, 2, 2, 2, 2, 2, 2, 2, 2, 2, 2, 2, 2, 2, 2, 2, 2, 2, 2, 2, 2, 2, 2, 2, 2, 2, 2, 2, 2, 3 ),
 ( 0.000000000000000000, 1.000000000000000000 ),
 ( 0.000000000000000000, 0.01851851851851851749, 0.03703703703703703498, 0.05555555555555555247, 0.07407407407407406996, 0.09259259259259258745, 0.1111111111111111049, 0.1296296296296296224, 0.1481481481481481399, 0.1666666666666666574, 0.1851851851851851749, 0.2037037037037036924, 0.2222222222222222099, 0.2407407407407407274, 0.2592592592592592449, 0.2777777777777777901, 0.2962962962962962798, 0.3148148148148148251, 0.3333333333333333148, 0.3518518518518518601, 0.3703703703703703498, 0.3888888888888888951, 0.4074074074074073848, 0.4259259259259259300, 0.4444444444444444198, 0.4629629629629629650, 0.4814814814814814548, 0.5000000000000000000, 0.5185185185185184897, 0.5370370370370370905, 0.5555555555555555802, 0.5740740740740740700, 0.5925925925925925597, 0.6111111111111111605, 0.6296296296296296502, 0.6481481481481481399, 0.6666666666666666297, 0.6851851851851852304, 0.7037037037037037202, 0.7222222222222222099, 0.7407407407407406996, 0.7592592592592593004, 0.7777777777777777901, 0.7962962962962962798, 0.8148148148148147696, 0.8333333333333333703, 0.8518518518518518601, 0.8703703703703703498, 0.8888888888888888395, 0.9074074074074074403, 0.9259259259259259300, 0.9444444444444444198, 0.9629629629629629095, 0.9814814814814815103, 1.000000000000000000 ),
 .UNSPECIFIED. ) 
 GEOMETRIC_REPRESENTATION_ITEM ( )  RATIONAL_B_SPLINE_SURFACE ( (
 ( 1.000000000000000000, 0.8660254037844387076, 1.000000000000000000, 0.8660254037844387076, 1.000000000000000000, 0.8660254037844387076, 1.000000000000000000, 0.8660254037844387076, 1.000000000000000000, 0.8660254037844387076, 1.000000000000000000, 0.8660254037844387076, 1.000000000000000000, 0.8660254037844387076, 1.000000000000000000, 0.8660254037844387076, 1.000000000000000000, 0.8660254037844387076, 1.000000000000000000, 0.8660254037844387076, 1.000000000000000000, 0.8660254037844387076, 1.000000000000000000, 0.8660254037844387076, 1.000000000000000000, 0.8660254037844387076, 1.000000000000000000, 0.8660254037844387076, 1.000000000000000000, 0.8660254037844387076, 1.000000000000000000, 0.8660254037844387076, 1.000000000000000000, 0.8660254037844387076, 1.000000000000000000, 0.8660254037844387076, 1.000000000000000000, 0.8660254037844387076, 1.000000000000000000, 0.8660254037844387076, 1.000000000000000000, 0.8660254037844387076, 1.000000000000000000, 0.8660254037844387076, 1.000000000000000000, 0.8660254037844387076, 1.000000000000000000, 0.8660254037844387076, 1.000000000000000000, 0.8660254037844387076, 1.000000000000000000, 0.8660254037844387076, 1.000000000000000000, 0.8660254037844387076, 1.000000000000000000, 0.8660254037844387076, 1.000000000000000000, 0.8660254037844387076, 1.000000000000000000, 0.8660254037844387076, 1.000000000000000000, 0.8660254037844387076, 1.000000000000000000, 0.8660254037844387076, 1.000000000000000000, 0.8660254037844387076, 1.000000000000000000, 0.8660254037844387076, 1.000000000000000000, 0.8660254037844387076, 1.000000000000000000, 0.8660254037844387076, 1.000000000000000000, 0.8660254037844387076, 1.000000000000000000, 0.8660254037844387076, 1.000000000000000000, 0.8660254037844387076, 1.000000000000000000, 0.8660254037844387076, 1.000000000000000000, 0.8660254037844387076, 1.000000000000000000, 0.8660254037844387076, 1.000000000000000000, 0.8660254037844387076, 1.000000000000000000, 0.8660254037844387076, 1.000000000000000000, 0.8660254037844387076, 1.000000000000000000, 0.8660254037844387076, 1.000000000000000000, 0.8660254037844387076, 1.000000000000000000, 0.8660254037844387076, 1.000000000000000000, 0.8660254037844387076, 1.000000000000000000, 0.8660254037844387076, 1.000000000000000000, 0.8660254037844387076, 1.000000000000000000, 0.8660254037844387076, 1.000000000000000000, 0.8660254037844387076, 1.000000000000000000, 0.8660254037844387076, 1.000000000000000000),
 ( 1.000000000000000000, 0.8660254037844387076, 1.000000000000000000, 0.8660254037844387076, 1.000000000000000000, 0.8660254037844387076, 1.000000000000000000, 0.8660254037844387076, 1.000000000000000000, 0.8660254037844387076, 1.000000000000000000, 0.8660254037844387076, 1.000000000000000000, 0.8660254037844387076, 1.000000000000000000, 0.8660254037844387076, 1.000000000000000000, 0.8660254037844387076, 1.000000000000000000, 0.8660254037844387076, 1.000000000000000000, 0.8660254037844387076, 1.000000000000000000, 0.8660254037844387076, 1.000000000000000000, 0.8660254037844387076, 1.000000000000000000, 0.8660254037844387076, 1.000000000000000000, 0.8660254037844387076, 1.000000000000000000, 0.8660254037844387076, 1.000000000000000000, 0.8660254037844387076, 1.000000000000000000, 0.8660254037844387076, 1.000000000000000000, 0.8660254037844387076, 1.000000000000000000, 0.8660254037844387076, 1.000000000000000000, 0.8660254037844387076, 1.000000000000000000, 0.8660254037844387076, 1.000000000000000000, 0.8660254037844387076, 1.000000000000000000, 0.8660254037844387076, 1.000000000000000000, 0.8660254037844387076, 1.000000000000000000, 0.8660254037844387076, 1.000000000000000000, 0.8660254037844387076, 1.000000000000000000, 0.8660254037844387076, 1.000000000000000000, 0.8660254037844387076, 1.000000000000000000, 0.8660254037844387076, 1.000000000000000000, 0.8660254037844387076, 1.000000000000000000, 0.8660254037844387076, 1.000000000000000000, 0.8660254037844387076, 1.000000000000000000, 0.8660254037844387076, 1.000000000000000000, 0.8660254037844387076, 1.000000000000000000, 0.8660254037844387076, 1.000000000000000000, 0.8660254037844387076, 1.000000000000000000, 0.8660254037844387076, 1.000000000000000000, 0.8660254037844387076, 1.000000000000000000, 0.8660254037844387076, 1.000000000000000000, 0.8660254037844387076, 1.000000000000000000, 0.8660254037844387076, 1.000000000000000000, 0.8660254037844387076, 1.000000000000000000, 0.8660254037844387076, 1.000000000000000000, 0.8660254037844387076, 1.000000000000000000, 0.8660254037844387076, 1.000000000000000000, 0.8660254037844387076, 1.000000000000000000, 0.8660254037844387076, 1.000000000000000000, 0.8660254037844387076, 1.000000000000000000, 0.8660254037844387076, 1.000000000000000000, 0.8660254037844387076, 1.000000000000000000, 0.8660254037844387076, 1.000000000000000000, 0.8660254037844387076, 1.000000000000000000, 0.8660254037844387076, 1.000000000000000000) ) ) 
 REPRESENTATION_ITEM ( '' )  SURFACE ( )  );
#17836=CARTESIAN_POINT ( 'NONE',  ( -57.64405989232413674, -3.920666489018320690E-15, 3.399999999999794298 ) ) ;
#17839=CARTESIAN_POINT ( 'NONE',  ( -44.59999999999998010, 8.366749974758271452E-15, -1.593320673368357319E-13 ) ) ;
#17841=CARTESIAN_POINT ( 'NONE',  ( -59.43714858239737708, 3.292580442886323233, 1.294864515003326444 ) ) ;
#17853=EDGE_LOOP ( 'NONE', ( #4467, #7198, #19162, #5980 ) ) ;
#17855=CARTESIAN_POINT ( 'NONE',  ( -59.18749999999995737, -3.399999999999991029, -2.288065396424332102E-13 ) ) ;
#17857=CARTESIAN_POINT ( 'NONE',  ( -59.69999999999997442, 3.400000000000007905, -2.001823990013003858E-13 ) ) ;
#17869=CARTESIAN_POINT ( 'NONE',  ( -54.76905989232412963, 2.944486372867092250, 1.699999999999816769 ) ) ;
#17873=CARTESIAN_POINT ( 'NONE',  ( -55.69702994616204705, 4.156921938165313080, -1.827997107644302771E-13 ) ) ;
#17875=DIRECTION ( 'NONE',  ( -1.000000000000000000, 1.219044193948983948E-29, -3.491481338843133355E-15 ) ) ;
#17878=CARTESIAN_POINT ( 'NONE',  ( -58.20655989232411542, -3.399999999999991029, -2.246812820714294660E-13 ) ) ;
#17880=CARTESIAN_POINT ( 'NONE',  ( -57.07202994616206126, 2.078460969082642773, 3.599999999999806022 ) ) ;
#17883=VERTEX_POINT ( 'NONE', #5135 ) ;
#17887=VECTOR ( 'NONE', #16882, 1000.000000000000000 ) ;
#17891=ORIENTED_EDGE ( 'NONE', *, *, #2967, .T. ) ;
#17894=ORIENTED_EDGE ( 'NONE', *, *, #6956, .T. ) ;
#17895=CARTESIAN_POINT ( 'NONE',  ( -59.32202994616204705, 2.078460969082646770, 3.599999999999797140 ) ) ;
#17910=CARTESIAN_POINT ( 'NONE',  ( -56.74999999999995737, 2.273606599708567113E-14, -3.400000000000201972 ) ) ;
#17917=CARTESIAN_POINT ( 'NONE',  ( -59.23418654921033522, -3.153953023162030078, 1.269874138521803975 ) ) ;
#17919=EDGE_LOOP ( 'NONE', ( #7425, #6286, #3955, #20437 ) ) ;
#17921=CARTESIAN_POINT ( 'NONE',  ( -54.49999999999999289, 1.399999999999995914, 3.959797974644419849 ) ) ;
#17937=CARTESIAN_POINT ( 'NONE',  ( -59.38452994616203995, 3.117691453623979481, 1.799999999999801092 ) ) ;
#17939=DIRECTION ( 'NONE',  ( -1.000000000000000000, 0.000000000000000000, -3.491481338842906952E-15 ) ) ;
#17943=VERTEX_POINT ( 'NONE', #8135 ) ;
#17944=CARTESIAN_POINT ( 'NONE',  ( -58.24999999999995737, 2.023778652682509052E-14, -3.400000000000207301 ) ) ;
#17950=ADVANCED_FACE ( 'NONE', ( #1308 ), #30285, .T. ) ;
#17957=CARTESIAN_POINT ( 'NONE',  ( -59.69934827995219706, 2.105468426063201282, 1.749007712897468814 ) ) ;
#17967=CARTESIAN_POINT ( 'NONE',  ( -58.24999999999995737, 2.023778652682509052E-14, -3.400000000000207301 ) ) ;
#17969=ORIENTED_EDGE ( 'NONE', *, *, #15115, .T. ) ;
#17971=AXIS2_PLACEMENT_3D ( 'NONE', #26128, #18860, #4441 ) ;
#17977=FACE_OUTER_BOUND ( 'NONE', #22628, .T. ) ;
#17985=CARTESIAN_POINT ( 'NONE',  ( -57.51905989232412963, -2.944486372867088697, 1.699999999999784350 ) ) ;
#17995=CARTESIAN_POINT ( 'NONE',  ( -54.39999999999997726, -1.399999999999992806, -1.984366583318788002E-13 ) ) ;
#17996=TOROIDAL_SURFACE ( 'NONE', #4329, 0.2000000000000000111, 0.1000000000000000056 ) ;
#18011=DIRECTION ( 'NONE',  ( 1.000000000000000000, -1.219044193948983948E-29, 3.491481338843133355E-15 ) ) ;
#18017=CARTESIAN_POINT ( 'NONE',  ( -44.49999999999998579, 2.308634493194285486, 1.301040651491409239 ) ) ;
#18030=CARTESIAN_POINT ( 'NONE',  ( -55.00952994616204705, 3.117691453623994580, -1.800000000000181899 ) ) ;
#18044=CARTESIAN_POINT ( 'NONE',  ( -58.07202994616203995, 2.078460969082688070, -3.600000000000190603 ) ) ;
#18049=CARTESIAN_POINT ( 'NONE',  ( -54.65400635094608361, -3.399999999999987477, -0.9110272542660231565 ) ) ;
#18056=ORIENTED_EDGE ( 'NONE', *, *, #8536, .F. ) ;
#18065=CIRCLE ( 'NONE', #18580, 0.09999999999999992228 ) ;
#18069=EDGE_CURVE ( 'NONE', #26071, #1323, #19492, .T. ) ;
#18084=CARTESIAN_POINT ( 'NONE',  ( -44.59999999999998721, 1.599999999999998090, 3.363870538531281706 ) ) ;
#18087=DIRECTION ( 'NONE',  ( -3.491481338843133355E-15, -3.491481338843133355E-15, 1.000000000000000000 ) ) ;
#18093=FACE_OUTER_BOUND ( 'NONE', #30334, .T. ) ;
#18096=EDGE_LOOP ( 'NONE', ( #28362, #22795, #7009, #21497 ) ) ;
#18103=DIRECTION ( 'NONE',  ( 3.491481338843133355E-15, 3.491481338843133355E-15, -1.000000000000000000 ) ) ;
#18112=CARTESIAN_POINT ( 'NONE',  ( -58.70655989232410832, 1.962990915244748891, -3.400000000000199751 ) ) ;
#18115=ORIENTED_EDGE ( 'NONE', *, *, #24764, .F. ) ;
#18117=ORIENTED_EDGE ( 'NONE', *, *, #8633, .F. ) ;
#18118=CARTESIAN_POINT ( 'NONE',  ( -58.99999999999995737, 2.023778652682509683E-14, -3.400000000000209521 ) ) ;
#18122=DIRECTION ( 'NONE',  ( 0.000000000000000000, 1.000000000000000000, 8.673617379884030739E-15 ) ) ;
#18135=CARTESIAN_POINT ( 'NONE',  ( -54.49999999999997868, -3.188085654472696540, 1.181570928782897267 ) ) ;
#18142=CARTESIAN_POINT ( 'NONE',  ( -56.31249999999998579, -1.962990915244731793, 3.399999999999792077 ) ) ;
#18149=DIRECTION ( 'NONE',  ( 0.000000000000000000, 1.000000000000000000, 3.491481338843130594E-15 ) ) ;
#18153=CARTESIAN_POINT ( 'NONE',  ( -54.49999999999997868, 8.366749974758391359E-15, -1.938977325913827332E-13 ) ) ;
#18161=CARTESIAN_POINT ( 'NONE',  ( -60.26905989232410121, 2.023778652682511261E-14, -3.400000000000213518 ) ) ;
#18162=CARTESIAN_POINT ( 'NONE',  ( -54.49999999999996447, -1.599999999999981215, -3.363870538531692489 ) ) ;
#18173=ADVANCED_FACE ( 'NONE', ( #4306 ), #22507, .T. ) ;
#18176=CARTESIAN_POINT ( 'NONE',  ( -59.66183546925923764, -3.174920041538525251, -1.216504307364950854 ) ) ;
#18191=ORIENTED_EDGE ( 'NONE', *, *, #31282, .F. ) ;
#18194=CARTESIAN_POINT ( 'NONE',  ( -54.50990849663458704, -3.088199225670062997, 1.451082037244374900 ) ) ;
#18206=CARTESIAN_POINT ( 'NONE',  ( -57.13452994616205416, 3.117691453623977260, 1.799999999999813971 ) ) ;
#18213=CARTESIAN_POINT ( 'NONE',  ( -57.31249999999996447, 3.400000000000008349, -1.881930883448047941E-13 ) ) ;
#18216=CARTESIAN_POINT ( 'NONE',  ( -59.17529728802922051, 2.511751407530337765, -0.9443652579017279836 ) ) ;
#18232=FACE_OUTER_BOUND ( 'NONE', #21702, .T. ) ;
#18237=CARTESIAN_POINT ( 'NONE',  ( -55.06249999999997158, 3.400000000000007905, -1.826733775103631524E-13 ) ) ;
#18248=CARTESIAN_POINT ( 'NONE',  ( -59.67318048135356179, -2.383480368854686393, -1.229362881338657454 ) ) ;
#18260=CARTESIAN_POINT ( 'NONE',  ( -56.25952994616206126, -1.280183170538300192E-14, 3.599999999999798916 ) ) ;
#18261=EDGE_CURVE ( 'NONE', #27932, #826, #1764, .T. ) ;
#18262=CARTESIAN_POINT ( 'NONE',  ( -59.45655989232410832, 1.962990915244748891, -3.400000000000202416 ) ) ;
#18267=CARTESIAN_POINT ( 'NONE',  ( -56.24999999999997868, -2.944486372867089141, 1.699999999999789235 ) ) ;
#18271=DIRECTION ( 'NONE',  ( 3.491481338843133355E-15, 3.491481338843133355E-15, -1.000000000000000000 ) ) ;
#18287=CARTESIAN_POINT ( 'NONE',  ( -56.24999999999997868, -2.944486372867089141, 1.699999999999789235 ) ) ;
#18291=DIRECTION ( 'NONE',  ( 0.000000000000000000, 0.4295302013422958032, 0.9030524935654886676 ) ) ;
#18306=DIRECTION ( 'NONE',  ( -1.000000000000000000, 1.219044193948983948E-29, -3.491481338843133355E-15 ) ) ;
#18310=CARTESIAN_POINT ( 'NONE',  ( -44.49999999999997868, -4.766731106216475591E-14, -1.485745783470907590E-13 ) ) ;
#18322=( BOUNDED_SURFACE ( )  B_SPLINE_SURFACE ( 1, 2, ( 
 ( #14656, #405, #4998, #24319, #10065, #19739, #23198, #15886, #25244, #1486, #3861, #8750, #15746, #10681, #17822, #27458, #29988, #8299, #20513, #8610, #20674, #5773, #20209, #8151, #20365, #30447, #22736, #3413, #18287, #18142, #25712, #10830, #15425, #25396, #30301, #25077, #13053, #3700, #22569, #10996, #27781, #11142, #29839, #30140, #13340, #28075, #8464, #6096, #6397, #15598, #1032, #1174, #6242, #13513, #23032, #25543, #16062, #20817, #18440, #10535, #17967, #27616, #1326, #12881, #5944, #27927, #3565, #13199, #22883, #876, #11287, #6867, #11628, #4019, #23671, #4646, #28404, #26343, #4493, #30779, #9406, #21146, #1627, #16535, #1962, #13807, #26190, #31256, #9090, #14147, #14301, #16369, #2112, #21307, #6706, #23972, #18761, #23823, #9579, #13662, #23344, #18606, #30936, #20970, #11776, #28879, #4323, #19240, #28248 ),
 ( #7187, #9252, #21451, #18913, #23491, #13975, #2266, #19075, #31081, #6558, #28730, #16855, #26015, #30603, #8916, #7040, #16219, #16702, #28556, #25866, #11929, #21617, #4168, #1784, #11462, #8082, #10455, #13129, #15201, #961, #19959, #26492, #15520, #27389, #20134, #14455, #3165, #4797, #14617, #24131, #3324, #17009, #10611, #4964, #2439, #65, #24849, #20438, #12975, #12099, #17589, #29765, #24285, #25174, #10756, #17747, #20289, #27236, #29918, #30063, #7338, #22664, #5549, #12658, #12807, #21778, #9726, #1106, #19385, #5698, #15349, #29594, #24996, #8378, #3015, #629, #22488, #22341, #8228, #17895, #29029, #26662, #7917, #10291, #786, #27531, #5857, #3491, #22818, #16143, #1707, #13586, #23276, #6175, #13269, #11221, #20601, #11375, #25326, #1562, #18683, #6029, #4100, #22958, #10909, #20895, #27706, #25792, #30525 ) ),
 .UNSPECIFIED., .F., .F., .F. ) 
 B_SPLINE_SURFACE_WITH_KNOTS ( ( 2, 2 ),
 ( 3, 2, 2, 2, 2, 2, 2, 2, 2, 2, 2, 2, 2, 2, 2, 2, 2, 2, 2, 2, 2, 2, 2, 2, 2, 2, 2, 2, 2, 2, 2, 2, 2, 2, 2, 2, 2, 2, 2, 2, 2, 2, 2, 2, 2, 2, 2, 2, 2, 2, 2, 2, 2, 2, 3 ),
 ( 0.000000000000000000, 1.000000000000000000 ),
 ( 0.000000000000000000, 0.01851851851851851749, 0.03703703703703703498, 0.05555555555555555247, 0.07407407407407406996, 0.09259259259259258745, 0.1111111111111111049, 0.1296296296296296224, 0.1481481481481481399, 0.1666666666666666574, 0.1851851851851851749, 0.2037037037037036924, 0.2222222222222222099, 0.2407407407407407274, 0.2592592592592592449, 0.2777777777777777901, 0.2962962962962962798, 0.3148148148148148251, 0.3333333333333333148, 0.3518518518518518601, 0.3703703703703703498, 0.3888888888888888951, 0.4074074074074073848, 0.4259259259259259300, 0.4444444444444444198, 0.4629629629629629650, 0.4814814814814814548, 0.5000000000000000000, 0.5185185185185184897, 0.5370370370370370905, 0.5555555555555555802, 0.5740740740740740700, 0.5925925925925925597, 0.6111111111111111605, 0.6296296296296296502, 0.6481481481481481399, 0.6666666666666666297, 0.6851851851851852304, 0.7037037037037037202, 0.7222222222222222099, 0.7407407407407406996, 0.7592592592592593004, 0.7777777777777777901, 0.7962962962962962798, 0.8148148148148147696, 0.8333333333333333703, 0.8518518518518518601, 0.8703703703703703498, 0.8888888888888888395, 0.9074074074074074403, 0.9259259259259259300, 0.9444444444444444198, 0.9629629629629629095, 0.9814814814814815103, 1.000000000000000000 ),
 .UNSPECIFIED. ) 
 GEOMETRIC_REPRESENTATION_ITEM ( )  RATIONAL_B_SPLINE_SURFACE ( (
 ( 1.000000000000000000, 0.8660254037844387076, 1.000000000000000000, 0.8660254037844387076, 1.000000000000000000, 0.8660254037844387076, 1.000000000000000000, 0.8660254037844387076, 1.000000000000000000, 0.8660254037844387076, 1.000000000000000000, 0.8660254037844387076, 1.000000000000000000, 0.8660254037844387076, 1.000000000000000000, 0.8660254037844387076, 1.000000000000000000, 0.8660254037844387076, 1.000000000000000000, 0.8660254037844387076, 1.000000000000000000, 0.8660254037844387076, 1.000000000000000000, 0.8660254037844387076, 1.000000000000000000, 0.8660254037844387076, 1.000000000000000000, 0.8660254037844387076, 1.000000000000000000, 0.8660254037844387076, 1.000000000000000000, 0.8660254037844387076, 1.000000000000000000, 0.8660254037844387076, 1.000000000000000000, 0.8660254037844387076, 1.000000000000000000, 0.8660254037844387076, 1.000000000000000000, 0.8660254037844387076, 1.000000000000000000, 0.8660254037844387076, 1.000000000000000000, 0.8660254037844387076, 1.000000000000000000, 0.8660254037844387076, 1.000000000000000000, 0.8660254037844387076, 1.000000000000000000, 0.8660254037844387076, 1.000000000000000000, 0.8660254037844387076, 1.000000000000000000, 0.8660254037844387076, 1.000000000000000000, 0.8660254037844387076, 1.000000000000000000, 0.8660254037844387076, 1.000000000000000000, 0.8660254037844387076, 1.000000000000000000, 0.8660254037844387076, 1.000000000000000000, 0.8660254037844387076, 1.000000000000000000, 0.8660254037844387076, 1.000000000000000000, 0.8660254037844387076, 1.000000000000000000, 0.8660254037844387076, 1.000000000000000000, 0.8660254037844387076, 1.000000000000000000, 0.8660254037844387076, 1.000000000000000000, 0.8660254037844387076, 1.000000000000000000, 0.8660254037844387076, 1.000000000000000000, 0.8660254037844387076, 1.000000000000000000, 0.8660254037844387076, 1.000000000000000000, 0.8660254037844387076, 1.000000000000000000, 0.8660254037844387076, 1.000000000000000000, 0.8660254037844387076, 1.000000000000000000, 0.8660254037844387076, 1.000000000000000000, 0.8660254037844387076, 1.000000000000000000, 0.8660254037844387076, 1.000000000000000000, 0.8660254037844387076, 1.000000000000000000, 0.8660254037844387076, 1.000000000000000000, 0.8660254037844387076, 1.000000000000000000, 0.8660254037844387076, 1.000000000000000000, 0.8660254037844387076, 1.000000000000000000, 0.8660254037844387076, 1.000000000000000000, 0.8660254037844387076, 1.000000000000000000),
 ( 1.000000000000000000, 0.8660254037844387076, 1.000000000000000000, 0.8660254037844387076, 1.000000000000000000, 0.8660254037844387076, 1.000000000000000000, 0.8660254037844387076, 1.000000000000000000, 0.8660254037844387076, 1.000000000000000000, 0.8660254037844387076, 1.000000000000000000, 0.8660254037844387076, 1.000000000000000000, 0.8660254037844387076, 1.000000000000000000, 0.8660254037844387076, 1.000000000000000000, 0.8660254037844387076, 1.000000000000000000, 0.8660254037844387076, 1.000000000000000000, 0.8660254037844387076, 1.000000000000000000, 0.8660254037844387076, 1.000000000000000000, 0.8660254037844387076, 1.000000000000000000, 0.8660254037844387076, 1.000000000000000000, 0.8660254037844387076, 1.000000000000000000, 0.8660254037844387076, 1.000000000000000000, 0.8660254037844387076, 1.000000000000000000, 0.8660254037844387076, 1.000000000000000000, 0.8660254037844387076, 1.000000000000000000, 0.8660254037844387076, 1.000000000000000000, 0.8660254037844387076, 1.000000000000000000, 0.8660254037844387076, 1.000000000000000000, 0.8660254037844387076, 1.000000000000000000, 0.8660254037844387076, 1.000000000000000000, 0.8660254037844387076, 1.000000000000000000, 0.8660254037844387076, 1.000000000000000000, 0.8660254037844387076, 1.000000000000000000, 0.8660254037844387076, 1.000000000000000000, 0.8660254037844387076, 1.000000000000000000, 0.8660254037844387076, 1.000000000000000000, 0.8660254037844387076, 1.000000000000000000, 0.8660254037844387076, 1.000000000000000000, 0.8660254037844387076, 1.000000000000000000, 0.8660254037844387076, 1.000000000000000000, 0.8660254037844387076, 1.000000000000000000, 0.8660254037844387076, 1.000000000000000000, 0.8660254037844387076, 1.000000000000000000, 0.8660254037844387076, 1.000000000000000000, 0.8660254037844387076, 1.000000000000000000, 0.8660254037844387076, 1.000000000000000000, 0.8660254037844387076, 1.000000000000000000, 0.8660254037844387076, 1.000000000000000000, 0.8660254037844387076, 1.000000000000000000, 0.8660254037844387076, 1.000000000000000000, 0.8660254037844387076, 1.000000000000000000, 0.8660254037844387076, 1.000000000000000000, 0.8660254037844387076, 1.000000000000000000, 0.8660254037844387076, 1.000000000000000000, 0.8660254037844387076, 1.000000000000000000, 0.8660254037844387076, 1.000000000000000000, 0.8660254037844387076, 1.000000000000000000, 0.8660254037844387076, 1.000000000000000000, 0.8660254037844387076, 1.000000000000000000) ) ) 
 REPRESENTATION_ITEM ( '' )  SURFACE ( )  );
#18336=CARTESIAN_POINT ( 'NONE',  ( -56.14405989232413674, -1.162579938981959285E-14, 3.399999999999799627 ) ) ;
#18350=EDGE_CURVE ( 'NONE', #30038, #18483, #14431, .T. ) ;
#18353=DIRECTION ( 'NONE',  ( 0.000000000000000000, -4.336808689942024836E-15, 1.000000000000000000 ) ) ;
#18362=CARTESIAN_POINT ( 'NONE',  ( -59.28448904087068883, -2.425384292835011557, -1.073600088316542411 ) ) ;
#18373=EDGE_CURVE ( 'NONE', #8368, #20255, #780, .T. ) ;
#18381=CARTESIAN_POINT ( 'NONE',  ( -59.69999999999998153, -2.279157448682842091, 1.538811659727345349 ) ) ;
#18389=EDGE_LOOP ( 'NONE', ( #1488, #30849, #18117, #11591 ) ) ;
#18401=ORIENTED_EDGE ( 'NONE', *, *, #16282, .T. ) ;
#18407=CARTESIAN_POINT ( 'NONE',  ( -58.45655989232412963, 1.962990915244722245, 3.399999999999800071 ) ) ;
#18415=CARTESIAN_POINT ( 'NONE',  ( -56.87499999999996447, -2.944486372867076707, -1.700000000000212674 ) ) ;
#18427=EDGE_CURVE ( 'NONE', #10413, #13311, #14246, .T. ) ;
#18434=CARTESIAN_POINT ( 'NONE',  ( -54.50000000000001421, -3.416259366980110901, 0.5361331873031048856 ) ) ;
#18440=CARTESIAN_POINT ( 'NONE',  ( -58.12499999999996447, 2.944486372867106905, -1.700000000000193801 ) ) ;
#18450=CARTESIAN_POINT ( 'NONE',  ( -59.69999999999997442, -3.237160264815294841, -1.238538609462289219 ) ) ;
#18452=CARTESIAN_POINT ( 'NONE',  ( -44.59999999999997300, 8.366749974758271452E-15, -1.593320673368357066E-13 ) ) ;
#18454=ORIENTED_EDGE ( 'NONE', *, *, #13224, .T. ) ;
#18464=AXIS2_PLACEMENT_3D ( 'NONE', #25509, #11254, #8717 ) ;
#18474=VECTOR ( 'NONE', #15992, 1000.000000000000000 ) ;
#18483=VERTEX_POINT ( 'NONE', #160 ) ;
#18484=EDGE_LOOP ( 'NONE', ( #23631, #24132, #1286, #5587 ) ) ;
#18496=CARTESIAN_POINT ( 'NONE',  ( -59.00952994616203284, -3.117691453623963938, -1.800000000000220757 ) ) ;
#18504=EDGE_CURVE ( 'NONE', #11045, #23968, #20068, .T. ) ;
#18506=CARTESIAN_POINT ( 'NONE',  ( -55.83155989232411542, -1.962990915244703372, -3.400000000000206413 ) ) ;
#18516=ADVANCED_FACE ( 'NONE', ( #5208 ), #12486, .F. ) ;
#18520=FACE_OUTER_BOUND ( 'NONE', #6087, .T. ) ;
#18541=CARTESIAN_POINT ( 'NONE',  ( -59.30412500704678536, 3.195544065279134038, 1.250136525132556242 ) ) ;
#18542=DIRECTION ( 'NONE',  ( -2.095850865446309212E-30, -1.000000000000000000, -2.891205793294679411E-15 ) ) ;
#18553=CARTESIAN_POINT ( 'NONE',  ( -54.39999999999997726, 8.366749974758487600E-15, -2.213041600731273397E-13 ) ) ;
#18571=CARTESIAN_POINT ( 'NONE',  ( -57.89405989232411542, 2.944486372867106461, -1.700000000000192912 ) ) ;
#18578=CARTESIAN_POINT ( 'NONE',  ( -55.57202994616207548, 2.078460969082646770, 3.599999999999810019 ) ) ;
#18580=AXIS2_PLACEMENT_3D ( 'NONE', #15257, #17325, #14787 ) ;
#18583=CYLINDRICAL_SURFACE ( 'NONE', #5918, 3.399999999999999911 ) ;
#18591=AXIS2_PLACEMENT_3D ( 'NONE', #28472, #11060, #16289 ) ;
#18599=AXIS2_PLACEMENT_3D ( 'NONE', #1840, #4213, #11333 ) ;
#18606=CARTESIAN_POINT ( 'NONE',  ( -60.81249999999997868, -1.962990915244731793, 3.399999999999776090 ) ) ;
#18616=CARTESIAN_POINT ( 'NONE',  ( -54.49821982711414847, -3.342839925777855381, -1.196915030700223426 ) ) ;
#18623=CARTESIAN_POINT ( 'NONE',  ( -55.77900635094609783, 3.400000000000004352, 0.9110272542656325800 ) ) ;
#18631=DIRECTION ( 'NONE',  ( 0.000000000000000000, -1.000000000000000000, -4.379659758543257010E-15 ) ) ;
#18632=CARTESIAN_POINT ( 'NONE',  ( -44.59999999999999432, 1.499999999999995781, 4.029888335921785192 ) ) ;
#18635=ORIENTED_EDGE ( 'NONE', *, *, #19827, .F. ) ;
#18647=CARTESIAN_POINT ( 'NONE',  ( -44.49999999999999289, 1.399999999999995914, 3.959797974644454044 ) ) ;
#18648=EDGE_LOOP ( 'NONE', ( #11661, #5112, #7867, #18678 ) ) ;
#18655=EDGE_CURVE ( 'NONE', #24129, #30441, #12216, .T. ) ;
#18656=DIRECTION ( 'NONE',  ( 0.000000000000000000, -1.000000000000000000, 0.000000000000000000 ) ) ;
#18658=CARTESIAN_POINT ( 'NONE',  ( -59.69702994616202574, -2.078460969082631227, -3.600000000000218137 ) ) ;
#18659=CARTESIAN_POINT ( 'NONE',  ( -59.41132486540516311, 3.161828374300071687, 1.250136525132550691 ) ) ;
#18666=CARTESIAN_POINT ( 'NONE',  ( -54.39999999999996305, 1.500000000000021316, -3.300094695611233142 ) ) ;
#18670=ORIENTED_EDGE ( 'NONE', *, *, #1087, .T. ) ;
#18678=ORIENTED_EDGE ( 'NONE', *, *, #26940, .F. ) ;
#18683=CARTESIAN_POINT ( 'NONE',  ( -60.63452994616204705, -3.117691453623976816, 1.799999999999772671 ) ) ;
#18691=DIRECTION ( 'NONE',  ( -1.000000000000000000, 1.219044193948983948E-29, -3.491481338843133355E-15 ) ) ;
#18711=CARTESIAN_POINT ( 'NONE',  ( -59.69999999999997442, 3.264622394567738617, -1.238538609462263240 ) ) ;
#18724=CARTESIAN_POINT ( 'NONE',  ( -59.69999999999997442, 8.366749974758454467E-15, -2.120534355533670266E-13 ) ) ;
#18727=EDGE_LOOP ( 'NONE', ( #22006, #888, #26706, #1096 ) ) ;
#18728=CARTESIAN_POINT ( 'NONE',  ( -55.57202994616207548, 2.078460969082644105, 3.599999999999811351 ) ) ;
#18731=CARTESIAN_POINT ( 'NONE',  ( -56.08155989232413674, -1.962990915244731571, 3.399999999999792077 ) ) ;
#18735=TOROIDAL_SURFACE ( 'NONE', #17214, 4.200000000000016165, 0.1000000000000000056 ) ;
#18738=CARTESIAN_POINT ( 'NONE',  ( -61.12499999999995737, 2.944486372867106905, -1.700000000000204459 ) ) ;
#18744=EDGE_CURVE ( 'NONE', #2592, #17201, #20031, .T. ) ;
#18747=DIRECTION ( 'NONE',  ( 0.000000000000000000, 1.000000000000000000, 3.491481338843132961E-15 ) ) ;
#18752=EDGE_CURVE ( 'NONE', #30275, #24434, #15331, .T. ) ;
#18761=CARTESIAN_POINT ( 'NONE',  ( -60.49999999999995737, 2.023778652682511576E-14, -3.400000000000214850 ) ) ;
#18764=DIRECTION ( 'NONE',  ( 1.000000000000000000, -1.219044193948983948E-29, 3.491481338843133355E-15 ) ) ;
#18765=ORIENTED_EDGE ( 'NONE', *, *, #9349, .T. ) ;
#18779=EDGE_CURVE ( 'NONE', #24434, #3601, #1788, .T. ) ;
#18781=EDGE_CURVE ( 'NONE', #3236, #30643, #5733, .T. ) ;
#18790=VERTEX_POINT ( 'NONE', #25776 ) ;
#18793=B_SPLINE_CURVE_WITH_KNOTS ( 'NONE', 3,
 ( #7248, #21982, #19155, #9319 ),
 .UNSPECIFIED., .F., .F.,
 ( 4, 4 ),
 ( 2.928550287019058723E-17, 7.626196476045024651E-05 ),
 .UNSPECIFIED. ) ;
#18795=CARTESIAN_POINT ( 'NONE',  ( -59.10064013560211293, -2.331281186115777615, 1.260011170057584451 ) ) ;
#18815=CARTESIAN_POINT ( 'NONE',  ( -58.44702994616205416, -2.078460969082657872, 3.599999999999784261 ) ) ;
#18825=DIRECTION ( 'NONE',  ( -3.491481338843133355E-15, -3.491481338843133355E-15, 1.000000000000000000 ) ) ;
#18826=CARTESIAN_POINT ( 'NONE',  ( -59.69999999999996732, -1.873569517744609447, -3.074042495181142698 ) ) ;
#18832=ORIENTED_EDGE ( 'NONE', *, *, #22250, .F. ) ;
#18847=DIRECTION ( 'NONE',  ( -1.000000000000000000, -0.000000000000000000, 0.000000000000000000 ) ) ;
#18848=CARTESIAN_POINT ( 'NONE',  ( -54.39999999999999147, -1.500000000000004441, 3.300094695610789941 ) ) ;
#18860=DIRECTION ( 'NONE',  ( 1.000000000000000000, -1.219044193948983948E-29, 3.491481338843133355E-15 ) ) ;
#18880=ORIENTED_EDGE ( 'NONE', *, *, #18655, .T. ) ;
#18881=CARTESIAN_POINT ( 'NONE',  ( -60.64405989232412253, -3.920666489018283614E-15, 3.399999999999783640 ) ) ;
#18886=CARTESIAN_POINT ( 'NONE',  ( -59.43749999999997868, 1.962990915244722689, 3.399999999999796962 ) ) ;
#18888=CARTESIAN_POINT ( 'NONE',  ( -59.19999999999996732, 4.156921938165317520, -0.9498634748674451567 ) ) ;
#18902=DIRECTION ( 'NONE',  ( -1.000000000000000000, 1.219044193948983948E-29, -3.491481338843133355E-15 ) ) ;
#18906=CARTESIAN_POINT ( 'NONE',  ( -54.39999999999997726, -4.766731106216463600E-14, -1.831402436016377855E-13 ) ) ;
#18913=CARTESIAN_POINT ( 'NONE',  ( -54.57202994616205416, -4.156921938165296204, -2.089175772356712570E-13 ) ) ;
#18921=CARTESIAN_POINT ( 'NONE',  ( -57.07202994616206126, 2.078460969082646770, 3.599999999999804690 ) ) ;
#18922=EDGE_LOOP ( 'NONE', ( #22610, #13265, #7708, #14176 ) ) ;
#18939=CARTESIAN_POINT ( 'NONE',  ( -56.76905989232412963, -2.944486372867094026, 1.699999999999778133 ) ) ;
#18943=DIRECTION ( 'NONE',  ( 0.000000000000000000, -1.000000000000000000, -3.491481338843132566E-15 ) ) ;
#18956=B_SPLINE_CURVE_WITH_KNOTS ( 'NONE', 3,
 ( #13524, #4180, #1639, #23359, #30460, #28090, #1975, #18616, #28260, #8621 ),
 .UNSPECIFIED., .F., .F.,
 ( 4, 2, 2, 2, 4 ),
 ( 1.563658610346375379E-18, 0.0005941303177189510886, 0.001188260635437900659, 0.001782390953156850122, 0.002376521270875800017 ),
 .UNSPECIFIED. ) ;
#18960=VERTEX_POINT ( 'NONE', #9934 ) ;
#18968=DIRECTION ( 'NONE',  ( -1.000000000000000000, -0.000000000000000000, 0.000000000000000000 ) ) ;
#18970=CARTESIAN_POINT ( 'NONE',  ( -59.25952994616205416, -4.643455692769875931E-15, 3.599999999999788702 ) ) ;
#18971=CARTESIAN_POINT ( 'NONE',  ( -59.11085193857230280, -2.468077931648963386, -0.9654581933252147641 ) ) ;
#18983=VERTEX_POINT ( 'NONE', #21835 ) ;
#18994=ADVANCED_FACE ( 'NONE', ( #26863 ), #4701, .T. ) ;
#19015=PLANE ( 'NONE',  #23614 ) ;
#19021=EDGE_LOOP ( 'NONE', ( #16740, #25029, #18115, #19268 ) ) ;
#19038=ORIENTED_EDGE ( 'NONE', *, *, #2549, .T. ) ;
#19046=B_SPLINE_CURVE_WITH_KNOTS ( 'NONE', 3,
 ( #3952, #8689, #3640, #13428, #13275, #9019, #25477, #22824, #30387, #1419, #8544, #23130, #6323 ),
 .UNSPECIFIED., .F., .F.,
 ( 4, 3, 3, 3, 4 ),
 ( 0.000000000000000000, 3.627661428711262821E-05, 7.228648945962581657E-05, 0.0001163236820996669683, 0.0001184416086866318864 ),
 .UNSPECIFIED. ) ;
#19048=CARTESIAN_POINT ( 'NONE',  ( -61.06249999999995737, 3.925981830489463142, -2.023818954174166834E-13 ) ) ;
#19052=CIRCLE ( 'NONE', #13443, 4.200000000000016165 ) ;
#19059=DIRECTION ( 'NONE',  ( 1.163827112947767259E-15, 0.9428090415820590264, -0.3333333333333461379 ) ) ;
#19066=LINE ( 'NONE', #26009, #16655 ) ;
#19070=ADVANCED_FACE ( 'NONE', ( #267 ), #4559, .T. ) ;
#19075=CARTESIAN_POINT ( 'NONE',  ( -54.82202994616206126, 2.078460969082646770, 3.599999999999812683 ) ) ;
#19083=CARTESIAN_POINT ( 'NONE',  ( -57.82202994616206126, 2.078460969082646770, 3.599999999999802025 ) ) ;
#19093=CARTESIAN_POINT ( 'NONE',  ( -54.39999999999996305, -1.399999999999979261, -3.959797974644882146 ) ) ;
#19099=CIRCLE ( 'NONE', #9486, 0.2000000000000000944 ) ;
#19114=CARTESIAN_POINT ( 'NONE',  ( -59.12687546363279267, -2.340603034507739100, 1.249089021148755752 ) ) ;
#19115=EDGE_LOOP ( 'NONE', ( #11366, #19450, #5626, #24082 ) ) ;
#19117=CARTESIAN_POINT ( 'NONE',  ( -54.39999999999997726, 8.366749974758389781E-15, -1.935485844574984262E-13 ) ) ;
#19138=CARTESIAN_POINT ( 'NONE',  ( -59.19999999999997442, 8.366749974758448157E-15, -2.103076948839454410E-13 ) ) ;
#19139=CARTESIAN_POINT ( 'NONE',  ( -56.38452994616205416, 3.117691453623979481, 1.799999999999811751 ) ) ;
#19140=CARTESIAN_POINT ( 'NONE',  ( -59.10126175476050037, -2.465973215592141887, -0.9703132807041499053 ) ) ;
#19146=CYLINDRICAL_SURFACE ( 'NONE', #26581, 0.1000000000000000472 ) ;
#19152=LINE ( 'NONE', #6303, #24718 ) ;
#19155=CARTESIAN_POINT ( 'NONE',  ( -59.68727869885009341, -3.216413352772560685, -1.231193962818940113 ) ) ;
#19162=ORIENTED_EDGE ( 'NONE', *, *, #4583, .F. ) ;
#19163=ORIENTED_EDGE ( 'NONE', *, *, #14012, .T. ) ;
#19191=CARTESIAN_POINT ( 'NONE',  ( -54.49999999999997868, 3.400000000000007905, -1.910919895035100347E-13 ) ) ;
#19212=EDGE_LOOP ( 'NONE', ( #22293, #1458, #18401, #25552 ) ) ;
#19213=AXIS2_PLACEMENT_3D ( 'NONE', #3660, #13295, #27736 ) ;
#19214=CARTESIAN_POINT ( 'NONE',  ( -54.38452994616203995, 2.093608279459366986E-14, -3.600000000000193268 ) ) ;
#19215=LINE ( 'NONE', #12669, #11531 ) ;
#19230=CARTESIAN_POINT ( 'NONE',  ( -54.39999999999996305, -1.599999999999981215, -3.363870538531692045 ) ) ;
#19240=CARTESIAN_POINT ( 'NONE',  ( -61.18749999999995737, 1.962990915244749557, -3.400000000000207745 ) ) ;
#19242=VERTEX_POINT ( 'NONE', #23225 ) ;
#19243=CARTESIAN_POINT ( 'NONE',  ( -59.52606392228539534, 3.344530751152334780, -1.138116568171968046 ) ) ;
#19247=CARTESIAN_POINT ( 'NONE',  ( -58.57202994616204705, 2.078460969082646770, 3.599999999999799805 ) ) ;
#19254=CARTESIAN_POINT ( 'NONE',  ( -54.39999999999999147, -1.400000000000004574, 3.363870538531238630 ) ) ;
#19259=DIRECTION ( 'NONE',  ( -1.499696682456171775E-15, 0.9030524935654854479, 0.4295302013423024645 ) ) ;
#19265=AXIS2_PLACEMENT_3D ( 'NONE', #12894, #10075, #29381 ) ;
#19268=ORIENTED_EDGE ( 'NONE', *, *, #22283, .F. ) ;
#19280=EDGE_LOOP ( 'NONE', ( #30241, #19996, #12666, #24090 ) ) ;
#19289=CARTESIAN_POINT ( 'NONE',  ( -59.57529047491064489, 3.036744713703804166, 1.534133291490011430 ) ) ;
#19290=CARTESIAN_POINT ( 'NONE',  ( -56.58155989232411542, -1.962990915244706924, -3.400000000000206857 ) ) ;
#19295=CARTESIAN_POINT ( 'NONE',  ( -54.49999999999999289, 1.399999999999995914, 3.959797974644418961 ) ) ;
#19300=CARTESIAN_POINT ( 'NONE',  ( -59.19999999999997442, -3.399999999999991473, -2.218921219761684346E-13 ) ) ;
#19308=CARTESIAN_POINT ( 'NONE',  ( -57.49999999999995737, 2.356882582050588150E-14, -3.400000000000204636 ) ) ;
#19334=CYLINDRICAL_SURFACE ( 'NONE', #9503, 0.1000000000000000472 ) ;
#19335=CARTESIAN_POINT ( 'NONE',  ( -59.40411988557205092, 3.289922720809018930, -1.067712145749284858 ) ) ;
#19349=ORIENTED_EDGE ( 'NONE', *, *, #21802, .F. ) ;
#19351=EDGE_LOOP ( 'NONE', ( #21453, #6864, #20977, #19997, #6403, #26508, #21569, #9723, #23701, #23781, #7335, #25290, #29537 ) ) ;
#19357=ORIENTED_EDGE ( 'NONE', *, *, #2449, .F. ) ;
#19360=CARTESIAN_POINT ( 'NONE',  ( -59.70655989232412253, -3.925981830489445379, -2.260242286469037332E-13 ) ) ;
#19365=CARTESIAN_POINT ( 'NONE',  ( -56.63452994616203284, 2.093608279459369510E-14, -3.600000000000201261 ) ) ;
#19370=CARTESIAN_POINT ( 'NONE',  ( -59.09999999999998010, -2.331118226142294247, 1.260312586522342349 ) ) ;
#19382=DIRECTION ( 'NONE',  ( 1.000000000000000000, -1.219044193948983948E-29, 3.491481338843133355E-15 ) ) ;
#19385=CARTESIAN_POINT ( 'NONE',  ( -58.63452994616204705, 3.117691453623979481, 1.799999999999803757 ) ) ;
#19386=ORIENTED_EDGE ( 'NONE', *, *, #7255, .T. ) ;
#19393=CARTESIAN_POINT ( 'NONE',  ( -56.32202994616206126, 2.078460969082646770, 3.599999999999807354 ) ) ;
#19396=EDGE_CURVE ( 'NONE', #24201, #13873, #5575, .T. ) ;
#19409=CARTESIAN_POINT ( 'NONE',  ( -44.49999999999997868, 8.366749974758269874E-15, -1.589829192029513996E-13 ) ) ;
#19435=CARTESIAN_POINT ( 'NONE',  ( -60.88452994616204705, 3.117691453623979481, 1.799999999999795985 ) ) ;
#19450=ORIENTED_EDGE ( 'NONE', *, *, #16045, .T. ) ;
#19451=DIRECTION ( 'NONE',  ( -1.000000000000000000, 1.219044193948983948E-29, -3.491481338843133355E-15 ) ) ;
#19457=ORIENTED_EDGE ( 'NONE', *, *, #7840, .F. ) ;
#19481=EDGE_CURVE ( 'NONE', #17058, #15357, #26100, .T. ) ;
#19485=EDGE_LOOP ( 'NONE', ( #29725, #4285, #11404, #9174 ) ) ;
#19487=DIRECTION ( 'NONE',  ( 1.000000000000000000, -1.219044193948983948E-29, 3.491481338843133355E-15 ) ) ;
#19492=CIRCLE ( 'NONE', #7348, 0.1000000000000000472 ) ;
#19496=EDGE_CURVE ( 'NONE', #16069, #6234, #30163, .T. ) ;
#19506=TOROIDAL_SURFACE ( 'NONE', #1281, 2.750000000000000000, 0.1000000000000000056 ) ;
#19512=CARTESIAN_POINT ( 'NONE',  ( -59.25952994616205416, -4.643455692769875931E-15, 3.599999999999788702 ) ) ;
#19519=AXIS2_PLACEMENT_3D ( 'NONE', #21295, #18902, #28544 ) ;
#19520=CARTESIAN_POINT ( 'NONE',  ( -59.23418654921033522, -3.153953023162030078, 1.269874138521803975 ) ) ;
#19542=FACE_OUTER_BOUND ( 'NONE', #24279, .T. ) ;
#19548=ORIENTED_EDGE ( 'NONE', *, *, #25772, .T. ) ;
#19551=CARTESIAN_POINT ( 'NONE',  ( -55.07202994616204705, 2.078460969082674747, -3.600000000000187494 ) ) ;
#19554=CARTESIAN_POINT ( 'NONE',  ( -56.37499999999998579, -1.162579938981958969E-14, 3.399999999999799183 ) ) ;
#19559=AXIS2_PLACEMENT_3D ( 'NONE', #29011, #29460, #22215 ) ;
#19560=DIRECTION ( 'NONE',  ( 0.000000000000000000, -4.336808689942006692E-15, 1.000000000000000000 ) ) ;
#19570=EDGE_CURVE ( 'NONE', #31281, #24820, #16553, .T. ) ;
#19596=ORIENTED_EDGE ( 'NONE', *, *, #18069, .T. ) ;
#19601=CIRCLE ( 'NONE', #18591, 0.1000000000000000472 ) ;
#19603=CARTESIAN_POINT ( 'NONE',  ( -55.95655989232412963, -3.925981830489445379, -2.129311736262419800E-13 ) ) ;
#19618=ORIENTED_EDGE ( 'NONE', *, *, #22283, .T. ) ;
#19639=ORIENTED_EDGE ( 'NONE', *, *, #14663, .F. ) ;
#19644=FACE_OUTER_BOUND ( 'NONE', #6250, .T. ) ;
#19645=EDGE_CURVE ( 'NONE', #18983, #6165, #28354, .T. ) ;
#19648=LINE ( 'NONE', #26596, #12081 ) ;
#19655=CARTESIAN_POINT ( 'NONE',  ( -54.48922267869908609, -2.367328842898039021, -2.672487423992893074 ) ) ;
#19660=VERTEX_POINT ( 'NONE', #19191 ) ;
#19662=CIRCLE ( 'NONE', #8023, 0.1000000000000028644 ) ;
#19668=VERTEX_POINT ( 'NONE', #2215 ) ;
#19673=CARTESIAN_POINT ( 'NONE',  ( -56.94702994616206126, -2.078460969082657872, 3.599999999999789591 ) ) ;
#19675=DIRECTION ( 'NONE',  ( 1.000000000000000000, -1.219044193948983948E-29, 3.491481338843133355E-15 ) ) ;
#19693=CIRCLE ( 'NONE', #13594, 2.649999999999999911 ) ;
#19701=DIRECTION ( 'NONE',  ( 1.000000000000000000, -1.219044193948983948E-29, 3.491481338843133355E-15 ) ) ;
#19708=CIRCLE ( 'NONE', #19213, 3.524999999999996358 ) ;
#19709=CARTESIAN_POINT ( 'NONE',  ( -60.25952994616203284, 3.117691453623994580, -1.800000000000200329 ) ) ;
#19711=CARTESIAN_POINT ( 'NONE',  ( -59.59999999999998010, 8.366749974758452890E-15, -2.117042874194827196E-13 ) ) ;
#19715=VERTEX_POINT ( 'NONE', #2065 ) ;
#19733=ORIENTED_EDGE ( 'NONE', *, *, #1798, .T. ) ;
#19737=CARTESIAN_POINT ( 'NONE',  ( -44.49999999999997868, 8.366749974758269874E-15, -1.589829192029513996E-13 ) ) ;
#19739=CARTESIAN_POINT ( 'NONE',  ( -54.81249999999998579, -1.962990915244731793, 3.399999999999796962 ) ) ;
#19749=CARTESIAN_POINT ( 'NONE',  ( -54.39999999999997726, -6.102218906431378987E-14, -2.213041600731275921E-13 ) ) ;
#19754=EDGE_CURVE ( 'NONE', #12035, #22982, #28974, .T. ) ;
#19755=CARTESIAN_POINT ( 'NONE',  ( -54.95655989232411542, 1.962990915244748891, -3.400000000000186429 ) ) ;
#19768=( NAMED_UNIT ( * ) PLANE_ANGLE_UNIT ( ) SI_UNIT ( $, .RADIAN. ) );
#19774=AXIS2_PLACEMENT_3D ( 'NONE', #30712, #18691, #3378 ) ;
#19782=DIRECTION ( 'NONE',  ( -1.000000000000000000, 1.219044193948983948E-29, -3.491481338843133355E-15 ) ) ;
#19784=EDGE_CURVE ( 'NONE', #16970, #15088, #29375, .T. ) ;
#19803=ORIENTED_EDGE ( 'NONE', *, *, #45, .F. ) ;
#19806=AXIS2_PLACEMENT_3D ( 'NONE', #25919, #11051, #6001 ) ;
#19809=DIRECTION ( 'NONE',  ( 0.000000000000000000, -1.000000000000000000, -3.491481338843133355E-15 ) ) ;
#19810=CARTESIAN_POINT ( 'NONE',  ( -59.19495429951913223, 2.548385458854359964, -0.9469503383365888149 ) ) ;
#19811=CARTESIAN_POINT ( 'NONE',  ( -59.64490075983744788, -2.179131191433543169, 1.525521932368567590 ) ) ;
#19818=CARTESIAN_POINT ( 'NONE',  ( -58.88452994616202574, 2.093608279459372350E-14, -3.600000000000208811 ) ) ;
#19824=CARTESIAN_POINT ( 'NONE',  ( -56.83155989232414385, -1.962990915244743562, 3.399999999999782752 ) ) ;
#19827=EDGE_CURVE ( 'NONE', #23968, #13230, #2511, .T. ) ;
#19843=ORIENTED_EDGE ( 'NONE', *, *, #9451, .T. ) ;
#19844=VERTEX_POINT ( 'NONE', #31302 ) ;
#19850=CARTESIAN_POINT ( 'NONE',  ( -59.19702994616205416, -2.078460969082657872, 3.599999999999782041 ) ) ;
#19854=CARTESIAN_POINT ( 'NONE',  ( -44.59999999999996589, 1.600000000000021627, -3.363870538531645416 ) ) ;
#19871=CARTESIAN_POINT ( 'NONE',  ( -59.19999999999997442, 4.156921938165309527, 1.250136525132554910 ) ) ;
#19873=EDGE_CURVE ( 'NONE', #18790, #11223, #11829, .T. ) ;
#19890=ORIENTED_EDGE ( 'NONE', *, *, #22832, .F. ) ;
#19896=CARTESIAN_POINT ( 'NONE',  ( -58.39405989232412963, -3.920666489018312013E-15, 3.399999999999791633 ) ) ;
#19905=CARTESIAN_POINT ( 'NONE',  ( -59.33448904220819742, 2.516908228110276369, -1.027510759589427058 ) ) ;
#19912=ORIENTED_EDGE ( 'NONE', *, *, #2468, .F. ) ;
#19937=ORIENTED_EDGE ( 'NONE', *, *, #19645, .T. ) ;
#19940=CARTESIAN_POINT ( 'NONE',  ( -58.58155989232410832, 3.400000000000007905, -1.908076882137507950E-13 ) ) ;
#19943=CARTESIAN_POINT ( 'NONE',  ( -56.63452994616203284, 2.358131988075197809E-14, -3.600000000000201261 ) ) ;
#19959=CARTESIAN_POINT ( 'NONE',  ( -56.25952994616206126, -4.643455692769913008E-15, 3.599999999999798916 ) ) ;
#19960=CARTESIAN_POINT ( 'NONE',  ( -59.19999999999997442, 2.435569474727625305, 1.250136525132548693 ) ) ;
#19961=CARTESIAN_POINT ( 'NONE',  ( -54.39999999999996305, 1.557046979865791769, -3.273565289175131010 ) ) ;
#19968=CARTESIAN_POINT ( 'NONE',  ( -56.57202994616203995, 2.078460969082674747, -3.600000000000191935 ) ) ;
#19974=FACE_OUTER_BOUND ( 'NONE', #7505, .T. ) ;
#19990=FACE_OUTER_BOUND ( 'NONE', #16773, .T. ) ;
#19996=ORIENTED_EDGE ( 'NONE', *, *, #2713, .T. ) ;
#19997=ORIENTED_EDGE ( 'NONE', *, *, #11276, .T. ) ;
#20003=CARTESIAN_POINT ( 'NONE',  ( -60.88452994616204705, 3.117691453623979481, 1.799999999999795985 ) ) ;
#20005=CARTESIAN_POINT ( 'NONE',  ( -56.18749999999997868, -3.399999999999991029, -2.152687225432237971E-13 ) ) ;
#20008=AXIS2_PLACEMENT_3D ( 'NONE', #16201, #23475, #11443 ) ;
#20017=EDGE_CURVE ( 'NONE', #5117, #15357, #13395, .T. ) ;
#20019=CIRCLE ( 'NONE', #12917, 0.1000000000000028644 ) ;
#20023=DIRECTION ( 'NONE',  ( 0.000000000000000000, -1.000000000000000000, -4.336808689942015369E-15 ) ) ;
#20024=FACE_OUTER_BOUND ( 'NONE', #19351, .T. ) ;
#20029=EDGE_LOOP ( 'NONE', ( #4460, #23628, #27655, #5996 ) ) ;
#20031=CIRCLE ( 'NONE', #30109, 2.750000000000000000 ) ;
#20036=CARTESIAN_POINT ( 'NONE',  ( -59.18207606663301590, 2.383656014762451036, 1.250136525132548693 ) ) ;
#20039=CARTESIAN_POINT ( 'NONE',  ( -59.42527672090727009, 2.245369935805367589, 1.420690871442056080 ) ) ;
#20056=VERTEX_POINT ( 'NONE', #23809 ) ;
#20059=CARTESIAN_POINT ( 'NONE',  ( -57.76905989232412963, 2.944486372867092250, 1.699999999999806111 ) ) ;
#20064=CARTESIAN_POINT ( 'NONE',  ( -59.19926633714428732, -2.436054758973382750, 1.249712944685305471 ) ) ;
#20068=B_SPLINE_CURVE_WITH_KNOTS ( 'NONE', 3,
 ( #29285, #26762, #16799, #27045, #17115, #7598, #5063, #19335, #9812, #462 ),
 .UNSPECIFIED., .F., .F.,
 ( 4, 3, 3, 4 ),
 ( 8.940560153363745023E-19, 6.454972243978038357E-05, 0.0001290994448803190853, 0.0002310882096523268108 ),
 .UNSPECIFIED. ) ;
#20071=FACE_OUTER_BOUND ( 'NONE', #17303, .T. ) ;
#20080=DIRECTION ( 'NONE',  ( -1.000000000000000000, 1.219044193948983948E-29, -3.491481338843133355E-15 ) ) ;
#20088=CARTESIAN_POINT ( 'NONE',  ( -57.76905989232412963, 2.944486372867089141, 1.699999999999811218 ) ) ;
#20091=EDGE_CURVE ( 'NONE', #24434, #2131, #3804, .T. ) ;
#20097=EDGE_LOOP ( 'NONE', ( #3667, #915, #17266, #29716 ) ) ;
#20104=CARTESIAN_POINT ( 'NONE',  ( -55.38452994616205416, -3.117691453623976816, 1.799999999999791100 ) ) ;
#20114=CARTESIAN_POINT ( 'NONE',  ( -59.69999999999997442, 8.366749974758454467E-15, -2.120534355533670266E-13 ) ) ;
#20115=EDGE_CURVE ( 'NONE', #24820, #30654, #8765, .T. ) ;
#20126=CARTESIAN_POINT ( 'NONE',  ( -59.14182443247880627, 2.482031228406460954, -0.9525887483575969927 ) ) ;
#20134=CARTESIAN_POINT ( 'NONE',  ( -56.50952994616203995, 3.117691453623994580, -1.800000000000187006 ) ) ;
#20146=CARTESIAN_POINT ( 'NONE',  ( -60.69702994616205416, -2.078460969082657872, 3.599999999999776712 ) ) ;
#20159=ORIENTED_EDGE ( 'NONE', *, *, #10257, .T. ) ;
#20173=DIRECTION ( 'NONE',  ( 0.000000000000000000, 1.000000000000000000, 3.491481338843130594E-15 ) ) ;
#20178=CARTESIAN_POINT ( 'NONE',  ( -58.75952994616203284, 3.117691453623994580, -1.800000000000195000 ) ) ;
#20185=AXIS2_PLACEMENT_3D ( 'NONE', #25046, #25217, #25518 ) ;
#20189=SPHERICAL_SURFACE ( 'NONE', #28928, 0.1000000000000000056 ) ;
#20192=CARTESIAN_POINT ( 'NONE',  ( -44.59999999999996589, 1.400000000000023892, -3.959797974644837293 ) ) ;
#20201=VERTEX_POINT ( 'NONE', #9857 ) ;
#20203=ORIENTED_EDGE ( 'NONE', *, *, #14792, .F. ) ;
#20209=CARTESIAN_POINT ( 'NONE',  ( -55.87499999999996447, 2.944486372867106905, -1.700000000000186029 ) ) ;
#20210=CARTESIAN_POINT ( 'NONE',  ( -59.67491082927361390, 2.027450992888311543, 1.706680806714727883 ) ) ;
#20218=ORIENTED_EDGE ( 'NONE', *, *, #27216, .T. ) ;
#20225=CARTESIAN_POINT ( 'NONE',  ( -57.20655989232410832, 1.962990915244748891, -3.400000000000194422 ) ) ;
#20236=ORIENTED_EDGE ( 'NONE', *, *, #17397, .T. ) ;
#20242=( BOUNDED_CURVE ( )  B_SPLINE_CURVE ( 2, ( #16287, #21215, #28317, #8817, #6624, #9165, #18826 ),
 .UNSPECIFIED., .F., .T. ) 
 B_SPLINE_CURVE_WITH_KNOTS ( ( 3, 2, 2, 3 ),
 ( 0.7554854200587094448, 0.7592592592592593004, 0.7777777777777777901, 0.7874476280263653649 ),
 .UNSPECIFIED. ) 
 CURVE ( )  GEOMETRIC_REPRESENTATION_ITEM ( )  RATIONAL_B_SPLINE_CURVE ( ( 0.9565230875206803818, 0.9726976765138894976, 1.000000000000000000, 0.8660254037844387076, 1.000000000000000000, 0.9300422287439487068, 0.9331444240391612022 ) ) 
 REPRESENTATION_ITEM ( '' )  );
#20255=VERTEX_POINT ( 'NONE', #26801 ) ;
#20265=CARTESIAN_POINT ( 'NONE',  ( -54.75952994616206837, -4.643455692769931152E-15, 3.599999999999804245 ) ) ;
#20268=DIRECTION ( 'NONE',  ( 0.000000000000000000, -1.000000000000000000, -3.491481338843132961E-15 ) ) ;
#20272=CARTESIAN_POINT ( 'NONE',  ( -56.88452994616205416, -3.117691453623982145, 1.799999999999776890 ) ) ;
#20289=CARTESIAN_POINT ( 'NONE',  ( -57.88452994616205416, 3.117691453623979481, 1.799999999999806422 ) ) ;
#20311=CARTESIAN_POINT ( 'NONE',  ( -59.49999999999997158, 2.944486372867082924, 1.699999999999817435 ) ) ;
#20329=ORIENTED_EDGE ( 'NONE', *, *, #6148, .T. ) ;
#20333=CARTESIAN_POINT ( 'NONE',  ( -59.44702994616203995, 4.156921938165313080, -1.958927657850919798E-13 ) ) ;
#20340=CIRCLE ( 'NONE', #20825, 2.750000000000000000 ) ;
#20341=CARTESIAN_POINT ( 'NONE',  ( -55.24999999999996447, 2.023778652682505581E-14, -3.400000000000196643 ) ) ;
#20345=DIRECTION ( 'NONE',  ( 1.000000000000000000, -1.219044193948983948E-29, 3.491481338843133355E-15 ) ) ;
#20349=CARTESIAN_POINT ( 'NONE',  ( -59.60191903105513234, 2.337626997591227163, -1.248237806062581168 ) ) ;
#20354=B_SPLINE_CURVE_WITH_KNOTS ( 'NONE', 3,
 ( #21994, #5191, #29411, #24819, #10256, #26570, #5336 ),
 .UNSPECIFIED., .F., .F.,
 ( 4, 3, 4 ),
 ( 0.000000000000000000, 3.138403403613116213E-05, 4.417314921333021443E-05 ),
 .UNSPECIFIED. ) ;
#20360=ORIENTED_EDGE ( 'NONE', *, *, #10592, .T. ) ;
#20365=CARTESIAN_POINT ( 'NONE',  ( -55.99999999999995737, 2.023778652682506212E-14, -3.400000000000199307 ) ) ;
#20368=VERTEX_POINT ( 'NONE', #3190 ) ;
#20377=CARTESIAN_POINT ( 'NONE',  ( -44.59999999999998721, -1.500000000000006661, 3.959797974644484242 ) ) ;
#20378=CARTESIAN_POINT ( 'NONE',  ( -59.64405989232410832, -2.944486372867076263, -1.700000000000222222 ) ) ;
#20385=CARTESIAN_POINT ( 'NONE',  ( -44.49999999999997868, 8.366749974758269874E-15, -1.589829192029513996E-13 ) ) ;
#20401=DIRECTION ( 'NONE',  ( 0.000000000000000000, 1.000000000000000000, 0.000000000000000000 ) ) ;
#20414=CARTESIAN_POINT ( 'NONE',  ( -55.32202994616205416, -4.156921938165296204, -2.115361882398036228E-13 ) ) ;
#20422=CARTESIAN_POINT ( 'NONE',  ( -56.38452994616205416, 3.117691453623977260, 1.799999999999815747 ) ) ;
#20429=CARTESIAN_POINT ( 'NONE',  ( -59.13174955718955772, 2.476889386167965945, -0.9565396329281473653 ) ) ;
#20433=ORIENTED_EDGE ( 'NONE', *, *, #1043, .T. ) ;
#20435=CARTESIAN_POINT ( 'NONE',  ( -58.95655989232411542, -3.399999999999991029, -2.281093130107142867E-13 ) ) ;
#20437=ORIENTED_EDGE ( 'NONE', *, *, #5908, .F. ) ;
#20438=CARTESIAN_POINT ( 'NONE',  ( -57.32202994616202574, 2.078460969082674747, -3.600000000000194600 ) ) ;
#20442=PRODUCT_CONTEXT ( 'NONE', #9144, 'mechanical' ) ;
#20464=ADVANCED_FACE ( 'NONE', ( #8862 ), #28591, .T. ) ;
#20482=CARTESIAN_POINT ( 'NONE',  ( -56.39405989232412253, 2.944486372867106461, -1.700000000000187583 ) ) ;
#20487=CARTESIAN_POINT ( 'NONE',  ( -58.49999999999997868, -2.944486372867089141, 1.699999999999781242 ) ) ;
#20489=CARTESIAN_POINT ( 'NONE',  ( -44.49999999999997868, -2.649999999999991918, -1.682353447508856999E-13 ) ) ;
#20498=DIRECTION ( 'NONE',  ( 1.000000000000000000, -1.219044193948983948E-29, 3.491481338843133355E-15 ) ) ;
#20513=CARTESIAN_POINT ( 'NONE',  ( -55.62499999999998579, -3.920666489018346722E-15, 3.399999999999801403 ) ) ;
#20514=CARTESIAN_POINT ( 'NONE',  ( -59.60960479401909851, 2.008809929642550784, 1.728346801590697757 ) ) ;
#20518=DIRECTION ( 'NONE',  ( 1.000000000000000000, -1.219044193948983948E-29, 3.491481338843133355E-15 ) ) ;
#20519=VERTEX_POINT ( 'NONE', #13922 ) ;
#20528=CARTESIAN_POINT ( 'NONE',  ( -59.70655989232412253, -3.925981830489445379, -2.260242286469037332E-13 ) ) ;
#20549=CARTESIAN_POINT ( 'NONE',  ( -59.65261300033996150, -3.078803759524879613, -1.467355461969038100 ) ) ;
#20562=DIRECTION ( 'NONE',  ( -1.000000000000000000, 1.219044193948983948E-29, -3.491481338843133355E-15 ) ) ;
#20567=CARTESIAN_POINT ( 'NONE',  ( -54.64405989232413674, -3.920666489018357767E-15, 3.399999999999804512 ) ) ;
#20576=CIRCLE ( 'NONE', #7400, 0.2000000000000000944 ) ;
#20580=AXIS2_PLACEMENT_3D ( 'NONE', #22268, #24170, #2937 ) ;
#20582=CARTESIAN_POINT ( 'NONE',  ( -57.88452994616205416, 3.117691453623976816, 1.799999999999811973 ) ) ;
#20591=CARTESIAN_POINT ( 'NONE',  ( -59.19495429951913223, 2.548385458854359964, -0.9469503383365888149 ) ) ;
#20601=CARTESIAN_POINT ( 'NONE',  ( -60.38452994616202574, 2.093608279459374244E-14, -3.600000000000214140 ) ) ;
#20625=EDGE_LOOP ( 'NONE', ( #12106, #15043, #13934, #10635, #22912, #18635, #17427, #19890, #6170 ) ) ;
#20627=CARTESIAN_POINT ( 'NONE',  ( -44.59999999999998721, 1.499999999999996003, 3.959797974644454488 ) ) ;
#20630=CARTESIAN_POINT ( 'NONE',  ( -59.65728261716281366, -2.366782727822243526, -1.230152085140890916 ) ) ;
#20644=CARTESIAN_POINT ( 'NONE',  ( -56.19702994616206837, -2.078460969082662757, 3.599999999999788702 ) ) ;
#20646=CARTESIAN_POINT ( 'NONE',  ( -57.51905989232412963, -2.944486372867088697, 1.699999999999784350 ) ) ;
#20651=CARTESIAN_POINT ( 'NONE',  ( -58.12499999999996447, 2.944486372867106905, -1.700000000000193801 ) ) ;
#20657=CARTESIAN_POINT ( 'NONE',  ( -59.69999999999997442, 8.366749974758454467E-15, -2.120534355533670266E-13 ) ) ;
#20658=AXIS2_PLACEMENT_3D ( 'NONE', #18153, #1040, #8308 ) ;
#20665=ADVANCED_FACE ( 'NONE', ( #31204 ), #2388, .T. ) ;
#20669=CARTESIAN_POINT ( 'NONE',  ( -54.49999999999999289, -3.325675108906214206, 0.8689164811911511688 ) ) ;
#20674=CARTESIAN_POINT ( 'NONE',  ( -55.74999999999997868, 2.944486372867092250, 1.699999999999813438 ) ) ;
#20680=CYLINDRICAL_SURFACE ( 'NONE', #12893, 3.625000000000024869 ) ;
#20695=EDGE_CURVE ( 'NONE', #8146, #16115, #20734, .T. ) ;
#20703=( BOUNDED_CURVE ( )  B_SPLINE_CURVE ( 3, ( #30282, #28229, #30431, #6079 ),
 .UNSPECIFIED., .F., .T. ) 
 B_SPLINE_CURVE_WITH_KNOTS ( ( 4, 4 ),
 ( 5.208023207023585677, 5.331808265806120772 ),
 .UNSPECIFIED. ) 
 CURVE ( )  GEOMETRIC_REPRESENTATION_ITEM ( )  RATIONAL_B_SPLINE_CURVE ( ( 1.000000000000000000, 0.9987235124983906420, 0.9987235124983906420, 1.000000000000000000 ) ) 
 REPRESENTATION_ITEM ( '' )  );
#20707=CARTESIAN_POINT ( 'NONE',  ( -59.18666126818025930, -2.395858435315754154, 1.242435404725767523 ) ) ;
#20708=VERTEX_POINT ( 'NONE', #15504 ) ;
#20712=DIRECTION ( 'NONE',  ( -1.000000000000000000, 1.219044193948984088E-29, -3.491481338843133750E-15 ) ) ;
#20720=ORIENTED_EDGE ( 'NONE', *, *, #12866, .F. ) ;
#20721=SPHERICAL_SURFACE ( 'NONE', #2917, 0.1000000000000000056 ) ;
#20726=DIRECTION ( 'NONE',  ( 1.000000000000000000, -1.219044193948983948E-29, 3.491481338843133355E-15 ) ) ;
#20734=( BOUNDED_CURVE ( )  B_SPLINE_CURVE ( 2, ( #22475, #24985, #1095, #18049, #25162 ),
 .UNSPECIFIED., .F., .T. ) 
 B_SPLINE_CURVE_WITH_KNOTS ( ( 3, 2, 3 ),
 ( 0.000000000000000000, 0.01851851851851851749, 0.02777777777777778317 ),
 .UNSPECIFIED. ) 
 CURVE ( )  GEOMETRIC_REPRESENTATION_ITEM ( )  RATIONAL_B_SPLINE_CURVE ( ( 1.000000000000000000, 0.8660254037844387076, 1.000000000000000000, 0.9330127018922192983, 0.9330127018922194093 ) ) 
 REPRESENTATION_ITEM ( '' )  );
#20741=VECTOR ( 'NONE', #5401, 1000.000000000000000 ) ;
#20766=CARTESIAN_POINT ( 'NONE',  ( -59.36201654190949029, 3.300626201927056247, 1.250136525132569787 ) ) ;
#20773=CARTESIAN_POINT ( 'NONE',  ( -59.24999999999997158, -2.944486372867095803, 1.699999999999767919 ) ) ;
#20784=ORIENTED_EDGE ( 'NONE', *, *, #21026, .F. ) ;
#20785=FACE_OUTER_BOUND ( 'NONE', #27349, .T. ) ;
#20788=DIRECTION ( 'NONE',  ( 1.000000000000000000, -1.219044193948983948E-29, 3.491481338843133355E-15 ) ) ;
#20789=ORIENTED_EDGE ( 'NONE', *, *, #20911, .T. ) ;
#20790=SHAPE_REPRESENTATION_RELATIONSHIP ( 'NONE' , 'NONE' ,  #25673, #12322 ) ;
#20793=CARTESIAN_POINT ( 'NONE',  ( -56.33155989232412253, 3.925981830489463142, -1.858639063162819723E-13 ) ) ;
#20798=CARTESIAN_POINT ( 'NONE',  ( -55.99999999999995737, 2.023778652682506212E-14, -3.400000000000199307 ) ) ;
#20801=FACE_OUTER_BOUND ( 'NONE', #3982, .T. ) ;
#20805=CARTESIAN_POINT ( 'NONE',  ( -44.59999999999996589, -1.557046979865753356, -3.273565289175108362 ) ) ;
#20810=ORIENTED_EDGE ( 'NONE', *, *, #20017, .T. ) ;
#20811=CARTESIAN_POINT ( 'NONE',  ( -54.49999999999999289, -3.459683327251550811, -0.6431504214706185163 ) ) ;
#20817=CARTESIAN_POINT ( 'NONE',  ( -58.06249999999997158, 3.925981830489463142, -1.919074514008873212E-13 ) ) ;
#20825=AXIS2_PLACEMENT_3D ( 'NONE', #3752, #23092, #11200 ) ;
#20835=CARTESIAN_POINT ( 'NONE',  ( -44.49999999999999289, 1.599999999999998090, 3.363870538531282151 ) ) ;
#20839=FACE_OUTER_BOUND ( 'NONE', #2764, .T. ) ;
#20843=EDGE_CURVE ( 'NONE', #7637, #13776, #16283, .T. ) ;
#20874=CARTESIAN_POINT ( 'NONE',  ( -56.69702994616203284, -2.078460969082631227, -3.600000000000207923 ) ) ;
#20894=CARTESIAN_POINT ( 'NONE',  ( -59.69999999999996021, 1.397030005794335672, -3.099726949734703751 ) ) ;
#20895=CARTESIAN_POINT ( 'NONE',  ( -60.94702994616203995, 4.156921938165313080, -2.011299877933566609E-13 ) ) ;
#20897=ORIENTED_EDGE ( 'NONE', *, *, #20843, .F. ) ;
#20901=SHAPE_DEFINITION_REPRESENTATION ( #37, #25673 ) ;
#20905=VERTEX_POINT ( 'NONE', #15957 ) ;
#20911=EDGE_CURVE ( 'NONE', #23157, #1451, #25620, .T. ) ;
#20920=CARTESIAN_POINT ( 'NONE',  ( -44.59999999999996589, -1.599999999999981215, -3.363870538531657850 ) ) ;
#20925=CARTESIAN_POINT ( 'NONE',  ( -59.19999999999996732, 2.580747833305914618, -0.9498634748674507078 ) ) ;
#20931=EDGE_CURVE ( 'NONE', #13697, #7185, #18793, .T. ) ;
#20936=CARTESIAN_POINT ( 'NONE',  ( -59.69999999999995310, -2.472655081704904223, -2.581384084800625978 ) ) ;
#20939=CARTESIAN_POINT ( 'NONE',  ( -54.69702994616206837, -2.078460969082657872, 3.599999999999797584 ) ) ;
#20940=CARTESIAN_POINT ( 'NONE',  ( -55.70655989232410832, 1.962990915244748891, -3.400000000000189093 ) ) ;
#20945=EDGE_LOOP ( 'NONE', ( #8846, #13057, #25933, #16192 ) ) ;
#20946=CARTESIAN_POINT ( 'NONE',  ( -58.18749999999995737, 1.962990915244749557, -3.400000000000197531 ) ) ;
#20956=CARTESIAN_POINT ( 'NONE',  ( -59.68687113065863059, 2.402179451507872709, -1.230958653213889198 ) ) ;
#20958=CARTESIAN_POINT ( 'NONE',  ( -59.65432904196666186, -2.186231771939587620, 1.524642732528142197 ) ) ;
#20965=EDGE_CURVE ( 'NONE', #8534, #7227, #12298, .T. ) ;
#20970=CARTESIAN_POINT ( 'NONE',  ( -60.93749999999997868, 1.962990915244722689, 3.399999999999791633 ) ) ;
#20977=ORIENTED_EDGE ( 'NONE', *, *, #10257, .F. ) ;
#20979=DIRECTION ( 'NONE',  ( -1.404304041445553711E-15, 0.9030524935654929974, 0.4295302013422866994 ) ) ;
#20987=CARTESIAN_POINT ( 'NONE',  ( -55.74999999999997868, 2.944486372867090473, 1.699999999999816547 ) ) ;
#20993=DIRECTION ( 'NONE',  ( -1.000000000000000000, 1.219044193948983948E-29, -3.491481338843133355E-15 ) ) ;
#20994=AXIS2_PLACEMENT_3D ( 'NONE', #24427, #19701, #17164 ) ;
#20995=CARTESIAN_POINT ( 'NONE',  ( -59.23418654921033522, -3.153953023162030078, 1.269874138521803975 ) ) ;
#21012=DIRECTION ( 'NONE',  ( 0.000000000000000000, -1.000000000000000000, -3.491481338843137694E-15 ) ) ;
#21024=VERTEX_POINT ( 'NONE', #435 ) ;
#21026=EDGE_CURVE ( 'NONE', #3612, #950, #9282, .T. ) ;
#21030=CARTESIAN_POINT ( 'NONE',  ( -57.44702994616203284, -2.078460969082631227, -3.600000000000210587 ) ) ;
#21039=EDGE_CURVE ( 'NONE', #20519, #16970, #5950, .T. ) ;
#21040=CIRCLE ( 'NONE', #11411, 4.199999999999954881 ) ;
#21061=CARTESIAN_POINT ( 'NONE',  ( -44.59999999999997300, -6.102218906431391608E-14, -1.870876429524648473E-13 ) ) ;
#21062=ORIENTED_EDGE ( 'NONE', *, *, #3470, .T. ) ;
#21074=VERTEX_POINT ( 'NONE', #10397 ) ;
#21079=CARTESIAN_POINT ( 'NONE',  ( -59.37241364122699849, 3.319464018575120967, 1.250136525132569787 ) ) ;
#21102=ORIENTED_EDGE ( 'NONE', *, *, #12567, .F. ) ;
#21108=EDGE_LOOP ( 'NONE', ( #8041, #8519, #12253, #27618, #26737, #12012, #18765 ) ) ;
#21113=CARTESIAN_POINT ( 'NONE',  ( -55.63452994616205416, 3.117691453623977704, 1.799999999999817524 ) ) ;
#21114=CARTESIAN_POINT ( 'NONE',  ( -57.26905989232410832, 2.023778652682507790E-14, -3.400000000000203304 ) ) ;
#21115=ORIENTED_EDGE ( 'NONE', *, *, #331, .T. ) ;
#21122=CARTESIAN_POINT ( 'NONE',  ( -59.81249999999995026, -1.962990915244707368, -3.400000000000219291 ) ) ;
#21125=DIRECTION ( 'NONE',  ( 0.000000000000000000, 1.000000000000000000, 3.491481338843133355E-15 ) ) ;
#21129=DIRECTION ( 'NONE',  ( -3.491481338843133355E-15, -3.491481338843133355E-15, 1.000000000000000000 ) ) ;
#21144=VECTOR ( 'NONE', #23997, 1000.000000000000000 ) ;
#21146=CARTESIAN_POINT ( 'NONE',  ( -59.56249999999996447, 3.925981830489463142, -1.971446734091520023E-13 ) ) ;
#21167=DIRECTION ( 'NONE',  ( 0.000000000000000000, 1.000000000000000000, 3.491481338843130594E-15 ) ) ;
#21174=CARTESIAN_POINT ( 'NONE',  ( -54.39999999999999147, 1.433333333333330906, 4.054078878802625852 ) ) ;
#21175=CARTESIAN_POINT ( 'NONE',  ( -59.63966108275621281, -2.141766704520198239, 1.560556113508256182 ) ) ;
#21182=EDGE_LOOP ( 'NONE', ( #28290, #10249, #9216, #23854, #10098, #4613, #27960, #19457, #26672, #20897, #31009, #828, #11031, #23086, #28289, #840, #24611, #19843, #12378, #28992, #28841, #19548 ) ) ;
#21203=CARTESIAN_POINT ( 'NONE',  ( -59.82202994616204705, -4.156921938165296204, -2.272478542645976661E-13 ) ) ;
#21207=AXIS2_PLACEMENT_3D ( 'NONE', #18906, #11923, #23666 ) ;
#21212=CARTESIAN_POINT ( 'NONE',  ( -55.61505354137802470, 3.400000000000011902, -0.9110272542660020623 ) ) ;
#21215=CARTESIAN_POINT ( 'NONE',  ( -59.49819002796308354, 3.306248072576822405, -1.473410355870489630 ) ) ;
#21217=FACE_OUTER_BOUND ( 'NONE', #31126, .T. ) ;
#21219=CARTESIAN_POINT ( 'NONE',  ( -57.12499999999997868, -6.418945959278930492E-15, 3.399999999999796518 ) ) ;
#21226=( GEOMETRIC_REPRESENTATION_CONTEXT ( 3 ) GLOBAL_UNCERTAINTY_ASSIGNED_CONTEXT ( ( #27224 ) ) GLOBAL_UNIT_ASSIGNED_CONTEXT ( ( #21276, #8878, #11110 ) ) REPRESENTATION_CONTEXT ( 'NONE', 'WORKASPACE' ) );
#21235=EDGE_CURVE ( 'NONE', #23968, #13697, #23959, .T. ) ;
#21241=EDGE_CURVE ( 'NONE', #30858, #26147, #15694, .T. ) ;
#21243=CIRCLE ( 'NONE', #15660, 0.1000000000000000472 ) ;
#21246=DIRECTION ( 'NONE',  ( -1.000000000000000000, 1.219044193948983948E-29, -3.491481338843133355E-15 ) ) ;
#21261=LINE ( 'NONE', #2219, #5906 ) ;
#21276=( LENGTH_UNIT ( ) NAMED_UNIT ( * ) SI_UNIT ( .MILLI., .METRE. ) );
#21279=ORIENTED_EDGE ( 'NONE', *, *, #26257, .F. ) ;
#21282=AXIS2_PLACEMENT_3D ( 'NONE', #19749, #10372, #9918 ) ;
#21283=CARTESIAN_POINT ( 'NONE',  ( -59.12499999999996447, -2.944486372867076707, -1.700000000000220446 ) ) ;
#21289=CARTESIAN_POINT ( 'NONE',  ( -44.59999999999996589, 1.400000000000021450, -3.363870538531645860 ) ) ;
#21295=CARTESIAN_POINT ( 'NONE',  ( -54.49999999999997868, 8.366749974758489177E-15, -2.216533082070116467E-13 ) ) ;
#21296=EDGE_CURVE ( 'NONE', #9375, #10212, #9752, .T. ) ;
#21307=CARTESIAN_POINT ( 'NONE',  ( -60.31249999999996447, 3.925981830489463142, -1.997632844132843428E-13 ) ) ;
#21313=CARTESIAN_POINT ( 'NONE',  ( -54.50952994616204705, -3.117691453623963938, -1.800000000000204770 ) ) ;
#21331=CARTESIAN_POINT ( 'NONE',  ( -44.49999999999999289, 1.514093959731539263, 3.183260039818184506 ) ) ;
#21347=ORIENTED_EDGE ( 'NONE', *, *, #11625, .T. ) ;
#21350=ORIENTED_EDGE ( 'NONE', *, *, #11625, .F. ) ;
#21359=CARTESIAN_POINT ( 'NONE',  ( -58.50952994616205416, -4.643455692769885398E-15, 3.599999999999791367 ) ) ;
#21362=CARTESIAN_POINT ( 'NONE',  ( -59.19999999999997442, -3.222669219888746550, 1.250136525132528931 ) ) ;
#21424=ORIENTED_EDGE ( 'NONE', *, *, #10812, .F. ) ;
#21425=CARTESIAN_POINT ( 'NONE',  ( -60.31249999999996447, 3.925981830489463142, -1.997632844132843428E-13 ) ) ;
#21428=CARTESIAN_POINT ( 'NONE',  ( -44.59999999999998721, -1.600000000000004530, 3.363870538531271936 ) ) ;
#21451=CARTESIAN_POINT ( 'NONE',  ( -54.50952994616204705, -3.117691453623963938, -1.800000000000204770 ) ) ;
#21453=ORIENTED_EDGE ( 'NONE', *, *, #15259, .T. ) ;
#21455=ORIENTED_EDGE ( 'NONE', *, *, #1043, .F. ) ;
#21457=CARTESIAN_POINT ( 'NONE',  ( -58.07202994616203995, 2.078460969082674747, -3.600000000000197709 ) ) ;
#21476=EDGE_CURVE ( 'NONE', #17704, #28363, #24452, .T. ) ;
#21497=ORIENTED_EDGE ( 'NONE', *, *, #30915, .F. ) ;
#21506=CARTESIAN_POINT ( 'NONE',  ( -55.94702994616203995, -2.078460969082631227, -3.600000000000205258 ) ) ;
#21560=CIRCLE ( 'NONE', #10418, 2.750000000000000000 ) ;
#21569=ORIENTED_EDGE ( 'NONE', *, *, #9569, .T. ) ;
#21572=( BOUNDED_CURVE ( )  B_SPLINE_CURVE ( 2, ( #27499, #24668, #7581, #29410, #17380, #5664, #5819, #5335, #12773 ),
 .UNSPECIFIED., .F., .T. ) 
 B_SPLINE_CURVE_WITH_KNOTS ( ( 3, 2, 2, 2, 3 ),
 ( 0.5277777777777777901, 0.5370370370370370905, 0.5555555555555555802, 0.5740740740740740700, 0.5833333333333333703 ),
 .UNSPECIFIED. ) 
 CURVE ( )  GEOMETRIC_REPRESENTATION_ITEM ( )  RATIONAL_B_SPLINE_CURVE ( ( 0.9330127018922194093, 0.9330127018922194093, 1.000000000000000000, 0.8660254037844387076, 1.000000000000000000, 0.8660254037844387076, 1.000000000000000000, 0.9330127018922189652, 0.9330127018922194093 ) ) 
 REPRESENTATION_ITEM ( '' )  );
#21583=CARTESIAN_POINT ( 'NONE',  ( -60.20655989232410832, 1.962990915244748891, -3.400000000000205969 ) ) ;
#21587=CARTESIAN_POINT ( 'NONE',  ( -60.62499999999995737, -2.944486372867076707, -1.700000000000225775 ) ) ;
#21589=FACE_OUTER_BOUND ( 'NONE', #2103, .T. ) ;
#21594=AXIS2_PLACEMENT_3D ( 'NONE', #10847, #18306, #6262 ) ;
#21614=AXIS2_PLACEMENT_3D ( 'NONE', #11239, #30884, #23615 ) ;
#21617=CARTESIAN_POINT ( 'NONE',  ( -55.69702994616204705, 4.156921938165313080, -1.827997107644302771E-13 ) ) ;
#21623=AXIS2_PLACEMENT_3D ( 'NONE', #3031, #5406, #24409 ) ;
#21626=CARTESIAN_POINT ( 'NONE',  ( -55.19702994616203284, -2.078460969082631227, -3.600000000000202593 ) ) ;
#21628=LINE ( 'NONE', #16378, #29230 ) ;
#21631=CARTESIAN_POINT ( 'NONE',  ( -59.19495429951913223, -2.548385458854336871, -0.9469503383366065785 ) ) ;
#21636=FACE_OUTER_BOUND ( 'NONE', #29645, .T. ) ;
#21649=CIRCLE ( 'NONE', #11496, 0.1000000000000000472 ) ;
#21653=ORIENTED_EDGE ( 'NONE', *, *, #5952, .T. ) ;
#21655=EDGE_LOOP ( 'NONE', ( #26988, #30976, #14144, #2072 ) ) ;
#21674=CARTESIAN_POINT ( 'NONE',  ( -59.19495429951913223, 2.548385458854359964, -0.9469503383365888149 ) ) ;
#21678=CARTESIAN_POINT ( 'NONE',  ( -54.26905989232411542, 2.023778652682504003E-14, -3.400000000000192646 ) ) ;
#21685=ORIENTED_EDGE ( 'NONE', *, *, #27605, .T. ) ;
#21702=EDGE_LOOP ( 'NONE', ( #9314, #12491, #12594, #19639, #30299, #12708 ) ) ;
#21711=CARTESIAN_POINT ( 'NONE',  ( -59.59999999999998721, -2.157671697750204842, 1.538490443495526216 ) ) ;
#21712=ORIENTED_EDGE ( 'NONE', *, *, #17352, .F. ) ;
#21725=EDGE_CURVE ( 'NONE', #2222, #2592, #22029, .T. ) ;
#21729=DIRECTION ( 'NONE',  ( 1.000000000000000000, -1.219044193948983948E-29, 3.491481338843133355E-15 ) ) ;
#21732=LINE ( 'NONE', #22024, #14563 ) ;
#21733=ORIENTED_EDGE ( 'NONE', *, *, #12866, .T. ) ;
#21734=ORIENTED_EDGE ( 'NONE', *, *, #8086, .F. ) ;
#21739=CIRCLE ( 'NONE', #30286, 2.649999999999999911 ) ;
#21744=CARTESIAN_POINT ( 'NONE',  ( -60.45655989232412253, -3.925981830489445379, -2.286428396510360233E-13 ) ) ;
#21751=CARTESIAN_POINT ( 'NONE',  ( -55.00952994616204705, 3.117691453623994580, -1.800000000000181899 ) ) ;
#21764=EDGE_CURVE ( 'NONE', #19844, #16856, #24845, .T. ) ;
#21777=CARTESIAN_POINT ( 'NONE',  ( -54.49999999999997868, -6.102218906431378987E-14, -2.216533082070118739E-13 ) ) ;
#21778=CARTESIAN_POINT ( 'NONE',  ( -58.44702994616205416, -2.078460969082657872, 3.599999999999784261 ) ) ;
#21786=CARTESIAN_POINT ( 'NONE',  ( -55.57202994616207548, 2.078460969082646770, 3.599999999999810019 ) ) ;
#21793=DIRECTION ( 'NONE',  ( -3.491481338843133355E-15, -3.491481338843133355E-15, 1.000000000000000000 ) ) ;
#21795=CARTESIAN_POINT ( 'NONE',  ( -59.35604502977157182, -3.238409345187212907, -1.039956114811810606 ) ) ;
#21802=EDGE_CURVE ( 'NONE', #18960, #10212, #22771, .T. ) ;
#21806=CARTESIAN_POINT ( 'NONE',  ( -59.10128028972211212, -2.331449503985936200, 1.259712628313877980 ) ) ;
#21826=CARTESIAN_POINT ( 'NONE',  ( -56.83155989232414385, -1.962990915244731571, 3.399999999999789413 ) ) ;
#21832=CARTESIAN_POINT ( 'NONE',  ( -59.36275712389306847, -2.351251615786114524, 1.344104394424739723 ) ) ;
#21835=CARTESIAN_POINT ( 'NONE',  ( -59.69999999999997442, 2.455304892039244180, -1.238538609462265905 ) ) ;
#21855=CARTESIAN_POINT ( 'NONE',  ( -59.09999999999997300, -2.649999999999991918, -1.947706029260935638E-13 ) ) ;
#21862=DIRECTION ( 'NONE',  ( 1.000000000000000000, -1.219044193948983948E-29, 3.491481338843133355E-15 ) ) ;
#21863=CARTESIAN_POINT ( 'NONE',  ( -44.49999999999997868, 8.366749974758366115E-15, -1.867384948185803131E-13 ) ) ;
#21866=VERTEX_POINT ( 'NONE', #22484 ) ;
#21871=CARTESIAN_POINT ( 'NONE',  ( -59.31908585006429036, 2.449738638601857588, -1.018617722459514763 ) ) ;
#21873=AXIS2_PLACEMENT_3D ( 'NONE', #29239, #17351, #7551 ) ;
#21890=VERTEX_POINT ( 'NONE', #27385 ) ;
#21898=ADVANCED_FACE ( 'NONE', ( #3319 ), #6752, .T. ) ;
#21901=CARTESIAN_POINT ( 'NONE',  ( -58.19702994616203284, -2.078460969082631227, -3.600000000000212363 ) ) ;
#21904=CARTESIAN_POINT ( 'NONE',  ( -54.39999999999997726, 8.366749974758487600E-15, -2.213041600731273397E-13 ) ) ;
#21923=DIRECTION ( 'NONE',  ( -1.000000000000000000, 1.219044193948983948E-29, -3.491481338843133355E-15 ) ) ;
#21931=CARTESIAN_POINT ( 'NONE',  ( -57.19702994616204705, 4.156921938165313080, -1.880369327726949834E-13 ) ) ;
#21939=CARTESIAN_POINT ( 'NONE',  ( -54.93749999999998579, 1.962990915244722689, 3.399999999999812506 ) ) ;
#21969=AXIS2_PLACEMENT_3D ( 'NONE', #12171, #7114, #17093 ) ;
#21970=CARTESIAN_POINT ( 'NONE',  ( -55.70655989232410832, 1.962990915244748891, -3.400000000000189093 ) ) ;
#21982=CARTESIAN_POINT ( 'NONE',  ( -59.67455719258389735, -3.195666608421381838, -1.223849197751685436 ) ) ;
#21985=CIRCLE ( 'NONE', #16416, 2.750000000000000000 ) ;
#21988=CARTESIAN_POINT ( 'NONE',  ( -59.19999999999997442, 3.400000000000007905, -1.910919895035100347E-13 ) ) ;
#21994=CARTESIAN_POINT ( 'NONE',  ( -59.69999999999997442, 2.455304892039244180, -1.238538609462265905 ) ) ;
#21999=CARTESIAN_POINT ( 'NONE',  ( -55.43749999999997868, -3.399999999999991473, -2.094585006122325661E-13 ) ) ;
#22006=ORIENTED_EDGE ( 'NONE', *, *, #19754, .T. ) ;
#22010=CARTESIAN_POINT ( 'NONE',  ( -59.09999999999997300, 8.366749974758448157E-15, -2.099585467500611340E-13 ) ) ;
#22024=CARTESIAN_POINT ( 'NONE',  ( -54.49999999999999289, 1.433333333333330906, 4.054078878802625852 ) ) ;
#22025=ADVANCED_FACE ( 'NONE', ( #18520 ), #29265, .T. ) ;
#22029=LINE ( 'NONE', #16815, #14366 ) ;
#22031=EDGE_LOOP ( 'NONE', ( #38, #14149, #10871, #15200 ) ) ;
#22039=ADVANCED_FACE ( 'NONE', ( #6959 ), #9840, .T. ) ;
#22042=CARTESIAN_POINT ( 'NONE',  ( -57.25952994616203995, 3.117691453623994580, -1.800000000000189671 ) ) ;
#22056=TOROIDAL_SURFACE ( 'NONE', #28623, 0.2000000000000000111, 0.1000000000000000056 ) ;
#22080=CARTESIAN_POINT ( 'NONE',  ( -56.57202994616203995, 2.078460969082674747, -3.600000000000191935 ) ) ;
#22084=CARTESIAN_POINT ( 'NONE',  ( -44.59999999999998010, -2.749999999999991562, -1.689336410186543392E-13 ) ) ;
#22091=( BOUNDED_CURVE ( )  B_SPLINE_CURVE ( 2, ( #17246, #10112, #12778, #7723, #12312, #10415, #22459, #17717, #29733 ),
 .UNSPECIFIED., .F., .T. ) 
 B_SPLINE_CURVE_WITH_KNOTS ( ( 3, 2, 2, 2, 3 ),
 ( 0.1944444444444444475, 0.2037037037037036924, 0.2222222222222222099, 0.2407407407407407274, 0.2500000000000000000 ),
 .UNSPECIFIED. ) 
 CURVE ( )  GEOMETRIC_REPRESENTATION_ITEM ( )  RATIONAL_B_SPLINE_CURVE ( ( 0.9330127018922192983, 0.9330127018922194093, 1.000000000000000000, 0.8660254037844387076, 1.000000000000000000, 0.8660254037844387076, 1.000000000000000000, 0.9330127018922191873, 0.9330127018922192983 ) ) 
 REPRESENTATION_ITEM ( '' )  );
#22096=AXIS2_PLACEMENT_3D ( 'NONE', #18888, #30912, #21125 ) ;
#22129=CARTESIAN_POINT ( 'NONE',  ( -54.58155989232414385, -1.962990915244731571, 3.399999999999797851 ) ) ;
#22149=CARTESIAN_POINT ( 'NONE',  ( -59.69999999999997442, 8.366749974758454467E-15, -2.120534355533670266E-13 ) ) ;
#22158=DIRECTION ( 'NONE',  ( -3.491481338843133355E-15, -3.491481338843133355E-15, 1.000000000000000000 ) ) ;
#22169=AXIS2_PLACEMENT_3D ( 'NONE', #11982, #28606, #17061 ) ;
#22185=DIRECTION ( 'NONE',  ( 0.000000000000000000, 0.3333333333333307058, 0.9428090415820643555 ) ) ;
#22189=AXIS2_PLACEMENT_3D ( 'NONE', #22332, #27054, #7145 ) ;
#22203=CARTESIAN_POINT ( 'NONE',  ( -57.63452994616205416, -3.117691453623976816, 1.799999999999783329 ) ) ;
#22215=DIRECTION ( 'NONE',  ( 0.000000000000000000, -1.000000000000000000, -3.491481338843129805E-15 ) ) ;
#22222=AXIS2_PLACEMENT_3D ( 'NONE', #27475, #1189, #721 ) ;
#22225=CARTESIAN_POINT ( 'NONE',  ( -58.37499999999996447, -2.944486372867072710, -1.700000000000224443 ) ) ;
#22238=AXIS2_PLACEMENT_3D ( 'NONE', #26772, #14727, #24388 ) ;
#22239=CARTESIAN_POINT ( 'NONE',  ( -55.58155989232412963, 3.925981830489463142, -1.832452953121496317E-13 ) ) ;
#22241=CARTESIAN_POINT ( 'NONE',  ( -56.56249999999997158, 3.400000000000008349, -1.863919195461974867E-13 ) ) ;
#22250=EDGE_CURVE ( 'NONE', #17127, #10254, #15258, .T. ) ;
#22253=EDGE_CURVE ( 'NONE', #6234, #4064, #3761, .T. ) ;
#22268=CARTESIAN_POINT ( 'NONE',  ( -54.39999999999997726, -1.399999999999992806, -1.984366583318788002E-13 ) ) ;
#22275=ORIENTED_EDGE ( 'NONE', *, *, #23659, .T. ) ;
#22278=CARTESIAN_POINT ( 'NONE',  ( -59.19999999999997442, 2.750000000000007994, -2.007061212021268338E-13 ) ) ;
#22281=CARTESIAN_POINT ( 'NONE',  ( -60.50952994616203284, -3.117691453623963938, -1.800000000000225864 ) ) ;
#22283=EDGE_CURVE ( 'NONE', #25749, #27693, #591, .T. ) ;
#22293=ORIENTED_EDGE ( 'NONE', *, *, #208, .F. ) ;
#22302=CARTESIAN_POINT ( 'NONE',  ( -44.59999999999998721, -1.500000000000004663, 3.363870538531272381 ) ) ;
#22305=CARTESIAN_POINT ( 'NONE',  ( -57.49005354137802470, -3.399999999999994138, 0.9110272542655952766 ) ) ;
#22307=DIRECTION ( 'NONE',  ( -3.491481338843133355E-15, -3.491481338843133355E-15, 1.000000000000000000 ) ) ;
#22316=CARTESIAN_POINT ( 'NONE',  ( -59.69999999999996732, -1.873569517744609447, -3.074042495181142698 ) ) ;
#22327=DIRECTION ( 'NONE',  ( 1.000000000000000000, -1.219044193948983948E-29, 3.491481338843133355E-15 ) ) ;
#22332=CARTESIAN_POINT ( 'NONE',  ( -54.49999999999996447, 1.500000000000023981, -4.029888335922182208 ) ) ;
#22333=CARTESIAN_POINT ( 'NONE',  ( -54.47257281981953270, -2.332729758745841764, -2.735898203255155980 ) ) ;
#22335=ORIENTED_EDGE ( 'NONE', *, *, #4072, .T. ) ;
#22337=CARTESIAN_POINT ( 'NONE',  ( -59.01905989232412253, -2.944486372867095358, 1.699999999999768363 ) ) ;
#22341=CARTESIAN_POINT ( 'NONE',  ( -59.19702994616205416, -2.078460969082657872, 3.599999999999782041 ) ) ;
#22349=CARTESIAN_POINT ( 'NONE',  ( -58.94702994616203284, -2.078460969082631227, -3.600000000000215472 ) ) ;
#22356=AXIS2_PLACEMENT_3D ( 'NONE', #19254, #4660, #7203 ) ;
#22381=CARTESIAN_POINT ( 'NONE',  ( -55.08155989232411542, -1.962990915244706924, -3.400000000000202416 ) ) ;
#22388=( BOUNDED_SURFACE ( )  B_SPLINE_SURFACE ( 1, 2, ( 
 ( #1970, #11634, #21313, #17716, #14775, #2120, #2273, #24292, #24433, #24138, #2744, #19551, #12248, #21626, #29196, #214, #5122, #12105, #7048, #21786, #71, #29035, #12390, #16861, #4971, #17017, #23829, #2446, #9876, #9732, #26671, #19393, #16709, #26498, #26351, #22080, #7197, #4501, #7344, #14463, #31261, #4803, #14625, #18921, #2602, #21931, #7510, #26196, #17173, #26817, #9259, #28563, #6875, #16544, #9414, #19083, #28885, #14155, #11782, #21457, #31088, #28736, #4654, #14307, #23978, #11938, #9588, #19247, #1002, #24749, #20178, #27116, #10181, #525, #22532, #25215, #8123, #19850, #836, #15393, #17937, #20333, #15568, #15245, #5743, #671, #25044, #3535, #12550, #17793, #10331, #17464, #7971, #26957, #19709, #5909, #29343, #10505, #3207, #3059, #29811, #13171, #29479, #5437, #20003, #12701, #7795, #2904, #3374 ),
 ( #29644, #375, #10040, #13025, #15090, #7653, #10655, #22707, #29962, #27432, #8269, #27578, #17314, #22381, #5267, #17634, #27280, #14918, #24583, #5598, #12850, #22239, #24891, #20940, #30420, #15861, #11424, #6211, #3987, #18731, #22858, #1146, #6070, #20793, #20482, #1600, #16341, #23171, #28373, #15721, #25516, #6527, #6676, #6361, #25985, #1755, #25835, #3827, #21114, #13779, #4293, #25684, #20646, #13631, #23317, #11261, #10798, #8723, #18571, #30570, #25368, #16023, #23463, #8881, #28221, #16187, #30273, #18407, #8580, #30105, #28046, #18112, #4143, #30752, #13474, #9058, #8428, #27749, #3674, #13310, #23002, #1292, #10957, #18262, #27900, #1454, #11114, #19360, #14115, #23793, #2233, #16974, #14420, #7162, #1934, #21583, #13941, #2083, #11594, #21744, #26784, #28847, #18881, #16824, #28525, #11897, #7470, #34, #11747 ) ),
 .UNSPECIFIED., .F., .F., .F. ) 
 B_SPLINE_SURFACE_WITH_KNOTS ( ( 2, 2 ),
 ( 3, 2, 2, 2, 2, 2, 2, 2, 2, 2, 2, 2, 2, 2, 2, 2, 2, 2, 2, 2, 2, 2, 2, 2, 2, 2, 2, 2, 2, 2, 2, 2, 2, 2, 2, 2, 2, 2, 2, 2, 2, 2, 2, 2, 2, 2, 2, 2, 2, 2, 2, 2, 2, 2, 3 ),
 ( 0.000000000000000000, 1.000000000000000000 ),
 ( 0.000000000000000000, 0.01851851851851851749, 0.03703703703703703498, 0.05555555555555555247, 0.07407407407407406996, 0.09259259259259258745, 0.1111111111111111049, 0.1296296296296296224, 0.1481481481481481399, 0.1666666666666666574, 0.1851851851851851749, 0.2037037037037036924, 0.2222222222222222099, 0.2407407407407407274, 0.2592592592592592449, 0.2777777777777777901, 0.2962962962962962798, 0.3148148148148148251, 0.3333333333333333148, 0.3518518518518518601, 0.3703703703703703498, 0.3888888888888888951, 0.4074074074074073848, 0.4259259259259259300, 0.4444444444444444198, 0.4629629629629629650, 0.4814814814814814548, 0.5000000000000000000, 0.5185185185185184897, 0.5370370370370370905, 0.5555555555555555802, 0.5740740740740740700, 0.5925925925925925597, 0.6111111111111111605, 0.6296296296296296502, 0.6481481481481481399, 0.6666666666666666297, 0.6851851851851852304, 0.7037037037037037202, 0.7222222222222222099, 0.7407407407407406996, 0.7592592592592593004, 0.7777777777777777901, 0.7962962962962962798, 0.8148148148148147696, 0.8333333333333333703, 0.8518518518518518601, 0.8703703703703703498, 0.8888888888888888395, 0.9074074074074074403, 0.9259259259259259300, 0.9444444444444444198, 0.9629629629629629095, 0.9814814814814815103, 1.000000000000000000 ),
 .UNSPECIFIED. ) 
 GEOMETRIC_REPRESENTATION_ITEM ( )  RATIONAL_B_SPLINE_SURFACE ( (
 ( 1.000000000000000000, 0.8660254037844387076, 1.000000000000000000, 0.8660254037844387076, 1.000000000000000000, 0.8660254037844387076, 1.000000000000000000, 0.8660254037844387076, 1.000000000000000000, 0.8660254037844387076, 1.000000000000000000, 0.8660254037844387076, 1.000000000000000000, 0.8660254037844387076, 1.000000000000000000, 0.8660254037844387076, 1.000000000000000000, 0.8660254037844387076, 1.000000000000000000, 0.8660254037844387076, 1.000000000000000000, 0.8660254037844387076, 1.000000000000000000, 0.8660254037844387076, 1.000000000000000000, 0.8660254037844387076, 1.000000000000000000, 0.8660254037844387076, 1.000000000000000000, 0.8660254037844387076, 1.000000000000000000, 0.8660254037844387076, 1.000000000000000000, 0.8660254037844387076, 1.000000000000000000, 0.8660254037844387076, 1.000000000000000000, 0.8660254037844387076, 1.000000000000000000, 0.8660254037844387076, 1.000000000000000000, 0.8660254037844387076, 1.000000000000000000, 0.8660254037844387076, 1.000000000000000000, 0.8660254037844387076, 1.000000000000000000, 0.8660254037844387076, 1.000000000000000000, 0.8660254037844387076, 1.000000000000000000, 0.8660254037844387076, 1.000000000000000000, 0.8660254037844387076, 1.000000000000000000, 0.8660254037844387076, 1.000000000000000000, 0.8660254037844387076, 1.000000000000000000, 0.8660254037844387076, 1.000000000000000000, 0.8660254037844387076, 1.000000000000000000, 0.8660254037844387076, 1.000000000000000000, 0.8660254037844387076, 1.000000000000000000, 0.8660254037844387076, 1.000000000000000000, 0.8660254037844387076, 1.000000000000000000, 0.8660254037844387076, 1.000000000000000000, 0.8660254037844387076, 1.000000000000000000, 0.8660254037844387076, 1.000000000000000000, 0.8660254037844387076, 1.000000000000000000, 0.8660254037844387076, 1.000000000000000000, 0.8660254037844387076, 1.000000000000000000, 0.8660254037844387076, 1.000000000000000000, 0.8660254037844387076, 1.000000000000000000, 0.8660254037844387076, 1.000000000000000000, 0.8660254037844387076, 1.000000000000000000, 0.8660254037844387076, 1.000000000000000000, 0.8660254037844387076, 1.000000000000000000, 0.8660254037844387076, 1.000000000000000000, 0.8660254037844387076, 1.000000000000000000, 0.8660254037844387076, 1.000000000000000000, 0.8660254037844387076, 1.000000000000000000, 0.8660254037844387076, 1.000000000000000000, 0.8660254037844387076, 1.000000000000000000, 0.8660254037844387076, 1.000000000000000000),
 ( 1.000000000000000000, 0.8660254037844387076, 1.000000000000000000, 0.8660254037844387076, 1.000000000000000000, 0.8660254037844387076, 1.000000000000000000, 0.8660254037844387076, 1.000000000000000000, 0.8660254037844387076, 1.000000000000000000, 0.8660254037844387076, 1.000000000000000000, 0.8660254037844387076, 1.000000000000000000, 0.8660254037844387076, 1.000000000000000000, 0.8660254037844387076, 1.000000000000000000, 0.8660254037844387076, 1.000000000000000000, 0.8660254037844387076, 1.000000000000000000, 0.8660254037844387076, 1.000000000000000000, 0.8660254037844387076, 1.000000000000000000, 0.8660254037844387076, 1.000000000000000000, 0.8660254037844387076, 1.000000000000000000, 0.8660254037844387076, 1.000000000000000000, 0.8660254037844387076, 1.000000000000000000, 0.8660254037844387076, 1.000000000000000000, 0.8660254037844387076, 1.000000000000000000, 0.8660254037844387076, 1.000000000000000000, 0.8660254037844387076, 1.000000000000000000, 0.8660254037844387076, 1.000000000000000000, 0.8660254037844387076, 1.000000000000000000, 0.8660254037844387076, 1.000000000000000000, 0.8660254037844387076, 1.000000000000000000, 0.8660254037844387076, 1.000000000000000000, 0.8660254037844387076, 1.000000000000000000, 0.8660254037844387076, 1.000000000000000000, 0.8660254037844387076, 1.000000000000000000, 0.8660254037844387076, 1.000000000000000000, 0.8660254037844387076, 1.000000000000000000, 0.8660254037844387076, 1.000000000000000000, 0.8660254037844387076, 1.000000000000000000, 0.8660254037844387076, 1.000000000000000000, 0.8660254037844387076, 1.000000000000000000, 0.8660254037844387076, 1.000000000000000000, 0.8660254037844387076, 1.000000000000000000, 0.8660254037844387076, 1.000000000000000000, 0.8660254037844387076, 1.000000000000000000, 0.8660254037844387076, 1.000000000000000000, 0.8660254037844387076, 1.000000000000000000, 0.8660254037844387076, 1.000000000000000000, 0.8660254037844387076, 1.000000000000000000, 0.8660254037844387076, 1.000000000000000000, 0.8660254037844387076, 1.000000000000000000, 0.8660254037844387076, 1.000000000000000000, 0.8660254037844387076, 1.000000000000000000, 0.8660254037844387076, 1.000000000000000000, 0.8660254037844387076, 1.000000000000000000, 0.8660254037844387076, 1.000000000000000000, 0.8660254037844387076, 1.000000000000000000, 0.8660254037844387076, 1.000000000000000000, 0.8660254037844387076, 1.000000000000000000, 0.8660254037844387076, 1.000000000000000000) ) ) 
 REPRESENTATION_ITEM ( '' )  SURFACE ( )  );
#22416=CARTESIAN_POINT ( 'NONE',  ( -59.69999999999997442, 8.366749974758454467E-15, -2.120534355533670266E-13 ) ) ;
#22420=CARTESIAN_POINT ( 'NONE',  ( -57.33155989232411542, -1.962990915244702039, -3.400000000000212630 ) ) ;
#22421=CARTESIAN_POINT ( 'NONE',  ( -58.93749999999996447, 1.962990915244761991, -3.400000000000193534 ) ) ;
#22425=CARTESIAN_POINT ( 'NONE',  ( -59.33155989232412253, 3.925981830489463142, -1.963383503328113345E-13 ) ) ;
#22442=ORIENTED_EDGE ( 'NONE', *, *, #9417, .F. ) ;
#22448=EDGE_LOOP ( 'NONE', ( #15749, #20203, #23241, #30973 ) ) ;
#22459=CARTESIAN_POINT ( 'NONE',  ( -56.12499999999996447, -2.944486372867074042, -1.700000000000214673 ) ) ;
#22460=CARTESIAN_POINT ( 'NONE',  ( -54.83155989232413674, 3.400000000000008349, -1.845326485282803322E-13 ) ) ;
#22462=CARTESIAN_POINT ( 'NONE',  ( -55.13452994616203995, 2.093608279459367933E-14, -3.600000000000195932 ) ) ;
#22471=CARTESIAN_POINT ( 'NONE',  ( -57.75952994616205416, -2.096020771799606953E-14, 3.599999999999794031 ) ) ;
#22475=CARTESIAN_POINT ( 'NONE',  ( -54.49999999999996447, 2.023778652682504319E-14, -3.400000000000193978 ) ) ;
#22478=DIRECTION ( 'NONE',  ( 0.000000000000000000, 0.3333333333333358683, -0.9428090415820624681 ) ) ;
#22482=ORIENTED_EDGE ( 'NONE', *, *, #13405, .T. ) ;
#22484=CARTESIAN_POINT ( 'NONE',  ( -59.68658240507107138, -2.223882124562203799, 1.531065007683262591 ) ) ;
#22488=CARTESIAN_POINT ( 'NONE',  ( -59.13452994616204705, -3.117691453623976816, 1.799999999999778000 ) ) ;
#22497=EDGE_LOOP ( 'NONE', ( #8103, #5559, #20218, #16251, #17132 ) ) ;
#22499=CARTESIAN_POINT ( 'NONE',  ( -58.57202994616204705, 2.078460969082646770, 3.599999999999799805 ) ) ;
#22501=CARTESIAN_POINT ( 'NONE',  ( -59.09999999999997300, 2.650000000000008349, -1.759412204284508433E-13 ) ) ;
#22502=CARTESIAN_POINT ( 'NONE',  ( -56.70655989232412253, -3.399999999999991029, -2.112596694108398482E-13 ) ) ;
#22503=CYLINDRICAL_SURFACE ( 'NONE', #7392, 0.1000000000000000472 ) ;
#22504=CARTESIAN_POINT ( 'NONE',  ( -54.81249999999998579, -1.962990915244732015, 3.399999999999796962 ) ) ;
#22505=CARTESIAN_POINT ( 'NONE',  ( -56.56249999999997158, 3.400000000000008349, -1.863919195461974867E-13 ) ) ;
#22507=TOROIDAL_SURFACE ( 'NONE', #20008, 3.524999999999996358, 0.1000000000000000056 ) ;
#22510=CARTESIAN_POINT ( 'NONE',  ( -59.43749999999997868, 1.962990915244716028, 3.399999999999800071 ) ) ;
#22517=CARTESIAN_POINT ( 'NONE',  ( -59.41132486539680713, 3.361433066165957051, 1.250136525132557574 ) ) ;
#22524=TOROIDAL_SURFACE ( 'NONE', #23023, 0.2000000000000000111, 0.1000000000000000056 ) ;
#22532=CARTESIAN_POINT ( 'NONE',  ( -59.00952994616203284, -3.117691453623963938, -1.800000000000220757 ) ) ;
#22547=TOROIDAL_SURFACE ( 'NONE', #4336, 0.2000000000000000111, 0.1000000000000000056 ) ;
#22549=VECTOR ( 'NONE', #23051, 1000.000000000000000 ) ;
#22555=CARTESIAN_POINT ( 'NONE',  ( -59.69999999999998153, 2.120235050790597153, 1.750136525132547360 ) ) ;
#22566=EDGE_CURVE ( 'NONE', #6992, #20708, #21985, .T. ) ;
#22569=CARTESIAN_POINT ( 'NONE',  ( -56.87499999999996447, -2.944486372867076707, -1.700000000000212674 ) ) ;
#22577=CIRCLE ( 'NONE', #24084, 0.1000000000000000472 ) ;
#22583=CARTESIAN_POINT ( 'NONE',  ( -57.42306624327022746, -3.399999999999988365, -0.9110272542660364792 ) ) ;
#22588=CARTESIAN_POINT ( 'NONE',  ( -57.83155989232412253, 3.925981830489463142, -1.911011283245466534E-13 ) ) ;
#22604=EDGE_LOOP ( 'NONE', ( #21424, #19912, #12383, #24913 ) ) ;
#22610=ORIENTED_EDGE ( 'NONE', *, *, #5588, .T. ) ;
#22614=CARTESIAN_POINT ( 'NONE',  ( -59.19999999999997442, -3.382957286162487698, 0.3399999999999019362 ) ) ;
#22628=EDGE_LOOP ( 'NONE', ( #9464, #11515, #27221, #13050, #24237, #13942, #1441, #20810, #29151, #14780, #13595, #20360, #10438, #4430, #13780, #29677, #28091, #10279 ) ) ;
#22631=DIRECTION ( 'NONE',  ( -3.491481338843133355E-15, -3.491481338843133355E-15, 1.000000000000000000 ) ) ;
#22647=CARTESIAN_POINT ( 'NONE',  ( -58.45655989232413674, 1.962990915244716694, 3.399999999999802736 ) ) ;
#22649=CARTESIAN_POINT ( 'NONE',  ( -58.63452994616204705, 3.117691453623969711, 1.799999999999821299 ) ) ;
#22658=CARTESIAN_POINT ( 'NONE',  ( -54.49999999999996447, -1.993349740317589935, -2.907263629733159327 ) ) ;
#22664=CARTESIAN_POINT ( 'NONE',  ( -58.19702994616203284, -2.078460969082631227, -3.600000000000212363 ) ) ;
#22665=DIRECTION ( 'NONE',  ( 1.000000000000000000, -1.219044193948983948E-29, 3.491481338843133355E-15 ) ) ;
#22674=DIRECTION ( 'NONE',  ( 7.637891338979824674E-45, -1.000000000000000000, -3.491481338843135327E-15 ) ) ;
#22693=CARTESIAN_POINT ( 'NONE',  ( -59.59999999999997300, -2.337126060168364994, -1.249136413240117038 ) ) ;
#22701=DIRECTION ( 'NONE',  ( 0.000000000000000000, 1.000000000000000000, 3.491481338843131383E-15 ) ) ;
#22704=CARTESIAN_POINT ( 'NONE',  ( -59.69999999999997442, 8.366749974758454467E-15, -2.120534355533670266E-13 ) ) ;
#22707=CARTESIAN_POINT ( 'NONE',  ( -54.70655989232413674, 1.962990915244722245, 3.399999999999812950 ) ) ;
#22710=CYLINDRICAL_SURFACE ( 'NONE', #27351, 0.1000000000000000472 ) ;
#22715=CARTESIAN_POINT ( 'NONE',  ( -58.74999999999997158, 2.944486372867092250, 1.699999999999803002 ) ) ;
#22720=EDGE_CURVE ( 'NONE', #15281, #826, #24029, .T. ) ;
#22724=CARTESIAN_POINT ( 'NONE',  ( -59.69142724121850563, 2.412383461849218591, -1.233589124872089826 ) ) ;
#22736=CARTESIAN_POINT ( 'NONE',  ( -56.12499999999996447, -2.944486372867076707, -1.700000000000210010 ) ) ;
#22746=CARTESIAN_POINT ( 'NONE',  ( -59.15400635094606940, -3.399999999999988365, -0.9110272542660506900 ) ) ;
#22749=CARTESIAN_POINT ( 'NONE',  ( -58.70655989232410832, 1.962990915244748891, -3.400000000000199751 ) ) ;
#22760=VECTOR ( 'NONE', #11148, 1000.000000000000000 ) ;
#22771=( BOUNDED_CURVE ( )  B_SPLINE_CURVE ( 2, ( #20435, #6024, #22337, #10752, #8374, #27061, #15198, #5379, #29913 ),
 .UNSPECIFIED., .F., .T. ) 
 B_SPLINE_CURVE_WITH_KNOTS ( ( 3, 2, 2, 2, 3 ),
 ( 0.6944444444444445308, 0.7037037037037037202, 0.7222222222222222099, 0.7407407407407406996, 0.7434165071384308821 ),
 .UNSPECIFIED. ) 
 CURVE ( )  GEOMETRIC_REPRESENTATION_ITEM ( )  RATIONAL_B_SPLINE_CURVE ( ( 0.9330127018922194093, 0.9330127018922197424, 1.000000000000000000, 0.8660254037844387076, 1.000000000000000000, 0.8660254037844387076, 1.000000000000000000, 0.9806418249743238391, 0.9668778290081130322 ) ) 
 REPRESENTATION_ITEM ( '' )  );
#22795=ORIENTED_EDGE ( 'NONE', *, *, #7255, .F. ) ;
#22799=EDGE_CURVE ( 'NONE', #20905, #27818, #8841, .T. ) ;
#22803=CARTESIAN_POINT ( 'NONE',  ( -58.69702994616204705, 4.156921938165313968, -1.807992169193672380E-13 ) ) ;
#22812=CARTESIAN_POINT ( 'NONE',  ( -54.39999999999999147, 1.557046979865768677, 3.273565289174698911 ) ) ;
#22818=CARTESIAN_POINT ( 'NONE',  ( -59.88452994616203995, -3.117691453623976816, 1.799999999999775335 ) ) ;
#22821=ADVANCED_FACE ( 'NONE', ( #11000 ), #20680, .T. ) ;
#22824=CARTESIAN_POINT ( 'NONE',  ( -59.37030229529103309, 2.324290318287153490, 1.279035047872993269 ) ) ;
#22827=ORIENTED_EDGE ( 'NONE', *, *, #18373, .T. ) ;
#22832=EDGE_CURVE ( 'NONE', #17785, #11045, #13462, .T. ) ;
#22835=LINE ( 'NONE', #18666, #1855 ) ;
#22838=DIRECTION ( 'NONE',  ( -1.000000000000000000, 1.219044193948983948E-29, -3.491481338843133355E-15 ) ) ;
#22850=ORIENTED_EDGE ( 'NONE', *, *, #25501, .T. ) ;
#22853=DIRECTION ( 'NONE',  ( 0.000000000000000000, 1.000000000000000000, 3.491481338843130594E-15 ) ) ;
#22858=CARTESIAN_POINT ( 'NONE',  ( -56.14405989232413674, -3.920666489018339623E-15, 3.399999999999799627 ) ) ;
#22864=CARTESIAN_POINT ( 'NONE',  ( -57.24999999999997158, 2.944486372867092250, 1.699999999999808109 ) ) ;
#22868=CARTESIAN_POINT ( 'NONE',  ( -54.49999999999996447, 1.400000000000023670, -3.959797974644871044 ) ) ;
#22872=DIRECTION ( 'NONE',  ( 1.000000000000000000, -1.219044193948983948E-29, 3.491481338843133355E-15 ) ) ;
#22883=CARTESIAN_POINT ( 'NONE',  ( -58.74999999999997158, 2.944486372867092250, 1.699999999999803002 ) ) ;
#22894=DIRECTION ( 'NONE',  ( -0.8660254037844369313, 1.745740669421577130E-15, -0.5000000000000029976 ) ) ;
#22897=CARTESIAN_POINT ( 'NONE',  ( -58.45655989232412963, 1.962990915244722245, 3.399999999999800071 ) ) ;
#22903=CARTESIAN_POINT ( 'NONE',  ( -54.39999999999999147, 1.499999999999995781, 4.029888335921750553 ) ) ;
#22912=ORIENTED_EDGE ( 'NONE', *, *, #12571, .F. ) ;
#22918=LINE ( 'NONE', #17857, #26787 ) ;
#22931=DIRECTION ( 'NONE',  ( -1.000000000000000000, 1.219044193948983948E-29, -3.491481338843133355E-15 ) ) ;
#22941=( BOUNDED_SURFACE ( )  B_SPLINE_SURFACE ( 3, 2, ( 
 ( #15142, #725, #10385 ),
 ( #17690, #27332, #8948 ),
 ( #1512, #13539, #11170 ),
 ( #23372, #11494, #21175 ) ),
 .UNSPECIFIED., .F., .F., .F. ) 
 B_SPLINE_SURFACE_WITH_KNOTS ( ( 4, 4 ),
 ( 3, 3 ),
 ( 5.207223707550983072, 5.342072618596839462 ),
 ( 0.000000000000000000, 1.000000000000000000 ),
 .UNSPECIFIED. ) 
 GEOMETRIC_REPRESENTATION_ITEM ( )  RATIONAL_B_SPLINE_SURFACE ( (
 ( 1.000000000000000000, 0.8400189050393593870, 1.000000000000000000),
 ( 1.000000000000000000, 0.8502146092435617364, 1.000000000000000000),
 ( 1.000000000000000000, 0.8598532762618735781, 1.000000000000000000),
 ( 1.000000000000000000, 0.8689053228414193031, 1.000000000000000000) ) ) 
 REPRESENTATION_ITEM ( '' )  SURFACE ( )  );
#22944=CARTESIAN_POINT ( 'NONE',  ( -57.32202994616203995, 2.078460969082687626, -3.600000000000187494 ) ) ;
#22958=CARTESIAN_POINT ( 'NONE',  ( -60.82202994616204705, 2.078460969082646770, 3.599999999999791367 ) ) ;
#22972=CARTESIAN_POINT ( 'NONE',  ( -59.69064771065831110, -2.230806985424941047, 1.533412112958392859 ) ) ;
#22973=CARTESIAN_POINT ( 'NONE',  ( -56.62499999999996447, 2.944486372867110457, -1.700000000000181810 ) ) ;
#22982=VERTEX_POINT ( 'NONE', #29339 ) ;
#23000=VERTEX_POINT ( 'NONE', #11107 ) ;
#23001=CARTESIAN_POINT ( 'NONE',  ( -56.07202994616204705, -4.156921938165296204, -2.235752804180006664E-13 ) ) ;
#23002=CARTESIAN_POINT ( 'NONE',  ( -59.26905989232412253, 2.944486372867092250, 1.699999999999800782 ) ) ;
#23004=CARTESIAN_POINT ( 'NONE',  ( -54.39999999999997726, -3.524999999999988365, -2.336116317925493832E-13 ) ) ;
#23008=CARTESIAN_POINT ( 'NONE',  ( -58.81249999999996447, 3.925981830489463142, -1.945260624050196617E-13 ) ) ;
#23023=AXIS2_PLACEMENT_3D ( 'NONE', #4764, #4462, #2406 ) ;
#23027=B_SPLINE_CURVE_WITH_KNOTS ( 'NONE', 3,
 ( #18381, #27403, #10628, #5712, #8395, #22972, #30393 ),
 .UNSPECIFIED., .F., .F.,
 ( 4, 3, 4 ),
 ( 0.000000000000000000, 3.294740569033884786E-05, 5.798545858612056943E-05 ),
 .UNSPECIFIED. ) ;
#23032=CARTESIAN_POINT ( 'NONE',  ( -57.87499999999997868, -3.920666489018319112E-15, 3.399999999999793854 ) ) ;
#23039=AXIS2_PLACEMENT_3D ( 'NONE', #18553, #28199, #3806 ) ;
#23044=CARTESIAN_POINT ( 'NONE',  ( -59.69999999999997442, -3.399999999999991473, -2.235080921937235780E-13 ) ) ;
#23050=CARTESIAN_POINT ( 'NONE',  ( -58.51905989232412253, 2.944486372867092250, 1.699999999999803446 ) ) ;
#23051=DIRECTION ( 'NONE',  ( -0.000000000000000000, 1.000000000000000000, 3.491481338843133355E-15 ) ) ;
#23058=CARTESIAN_POINT ( 'NONE',  ( -54.49999999999998579, -1.514093959731547701, 3.183260039818139209 ) ) ;
#23077=ORIENTED_EDGE ( 'NONE', *, *, #6721, .F. ) ;
#23081=CIRCLE ( 'NONE', #23574, 0.1000000000000000472 ) ;
#23082=ORIENTED_EDGE ( 'NONE', *, *, #22566, .F. ) ;
#23086=ORIENTED_EDGE ( 'NONE', *, *, #16282, .F. ) ;
#23092=DIRECTION ( 'NONE',  ( -1.000000000000000000, 1.219044193948983948E-29, -3.491481338843133355E-15 ) ) ;
#23095=CIRCLE ( 'NONE', #4360, 0.1000000000000000472 ) ;
#23110=ORIENTED_EDGE ( 'NONE', *, *, #16676, .T. ) ;
#23113=ORIENTED_EDGE ( 'NONE', *, *, #20911, .F. ) ;
#23130=CARTESIAN_POINT ( 'NONE',  ( -59.35396298745919097, 2.308928725093315926, 1.300518551040214188 ) ) ;
#23148=CARTESIAN_POINT ( 'NONE',  ( -44.59999999999999432, -1.400000000000007017, 4.029888335921774534 ) ) ;
#23155=PLANE ( 'NONE',  #17685 ) ;
#23157=VERTEX_POINT ( 'NONE', #13018 ) ;
#23165=ORIENTED_EDGE ( 'NONE', *, *, #9527, .T. ) ;
#23169=CARTESIAN_POINT ( 'NONE',  ( -54.82202994616206126, 2.078460969082646770, 3.599999999999812683 ) ) ;
#23171=CARTESIAN_POINT ( 'NONE',  ( -56.58155989232411542, -1.962990915244706924, -3.400000000000206857 ) ) ;
#23172=ORIENTED_EDGE ( 'NONE', *, *, #15803, .T. ) ;
#23177=CARTESIAN_POINT ( 'NONE',  ( -55.31249999999997158, -1.962990915244707368, -3.400000000000203304 ) ) ;
#23188=CARTESIAN_POINT ( 'NONE',  ( -59.61639066107911589, 2.342446846742921807, -1.242019481833310568 ) ) ;
#23189=CARTESIAN_POINT ( 'NONE',  ( -59.69824320556942610, 2.099492949945970466, 1.747093667920370352 ) ) ;
#23198=CARTESIAN_POINT ( 'NONE',  ( -54.87499999999998579, -3.920666489018356189E-15, 3.399999999999804068 ) ) ;
#23208=CARTESIAN_POINT ( 'NONE',  ( -54.39999999999997726, -6.102218906431378987E-14, -2.213041600731275921E-13 ) ) ;
#23225=CARTESIAN_POINT ( 'NONE',  ( -44.49999999999997868, 2.750000000000007994, -1.490445676513672770E-13 ) ) ;
#23237=ORIENTED_EDGE ( 'NONE', *, *, #10592, .F. ) ;
#23241=ORIENTED_EDGE ( 'NONE', *, *, #4608, .F. ) ;
#23245=ORIENTED_EDGE ( 'NONE', *, *, #7085, .T. ) ;
#23248=DIRECTION ( 'NONE',  ( 0.000000000000000000, 1.000000000000000000, 4.336808689942015369E-15 ) ) ;
#23251=CARTESIAN_POINT ( 'NONE',  ( -54.39999999999999147, 1.599999999999998090, 3.363870538531247512 ) ) ;
#23254=CARTESIAN_POINT ( 'NONE',  ( -57.50952994616203995, -3.117691453623963938, -1.800000000000215206 ) ) ;
#23268=CARTESIAN_POINT ( 'NONE',  ( -44.59999999999996589, 1.500000000000023759, -3.959797974644836405 ) ) ;
#23274=CIRCLE ( 'NONE', #9120, 3.625000000000024869 ) ;
#23276=CARTESIAN_POINT ( 'NONE',  ( -60.13452994616204705, 3.117691453623979481, 1.799999999999798428 ) ) ;
#23287=ORIENTED_EDGE ( 'NONE', *, *, #5001, .T. ) ;
#23294=ADVANCED_FACE ( 'NONE', ( #4578 ), #9509, .T. ) ;
#23303=CARTESIAN_POINT ( 'NONE',  ( -59.19834903927996805, 2.558621439192835023, -0.9489102922513357186 ) ) ;
#23304=DIRECTION ( 'NONE',  ( -0.4999999999999965583, 3.023711536277464094E-15, -0.8660254037844407060 ) ) ;
#23308=DIRECTION ( 'NONE',  ( -1.000000000000000000, 1.219044193948983948E-29, -3.491481338843133355E-15 ) ) ;
#23310=DIRECTION ( 'NONE',  ( 0.000000000000000000, 1.000000000000000000, 3.491481338843133355E-15 ) ) ;
#23317=CARTESIAN_POINT ( 'NONE',  ( -57.64405989232413674, -3.920666489018320690E-15, 3.399999999999794298 ) ) ;
#23321=CARTESIAN_POINT ( 'NONE',  ( -58.06249999999997158, 3.925981830489463142, -1.919074514008873212E-13 ) ) ;
#23322=CARTESIAN_POINT ( 'NONE',  ( -54.86505354137801760, 3.400000000000011458, -0.9110272542659999528 ) ) ;
#23328=EDGE_CURVE ( 'NONE', #6022, #4064, #4678, .T. ) ;
#23329=CARTESIAN_POINT ( 'NONE',  ( -44.49999999999996447, 1.400000000000021450, -3.363870538531645416 ) ) ;
#23331=B_SPLINE_CURVE_WITH_KNOTS ( 'NONE', 3,
 ( #22693, #1132, #988, #1439, #3974, #10640, #13614, #8413, #29948, #1275, #20630, #8565, #18248, #30406, #8256, #6199 ),
 .UNSPECIFIED., .F., .F.,
 ( 4, 3, 3, 3, 3, 4 ),
 ( -2.177409780393270631E-06, 0.000000000000000000, 1.647199373531996907E-05, 5.453032561112638088E-05, 8.914430023005323329E-05, 0.0001239676331529264105 ),
 .UNSPECIFIED. ) ;
#23332=DIRECTION ( 'NONE',  ( 1.000000000000000000, -1.219044193948983948E-29, 3.491481338843133355E-15 ) ) ;
#23333=CARTESIAN_POINT ( 'NONE',  ( -59.64819772016205235, 2.360117159334230053, -1.232121303804335488 ) ) ;
#23344=CARTESIAN_POINT ( 'NONE',  ( -60.74999999999997158, -2.944486372867089141, 1.699999999999773248 ) ) ;
#23357=CARTESIAN_POINT ( 'NONE',  ( -44.59999999999998721, -1.514093959731547478, 3.183260039818173404 ) ) ;
#23359=CARTESIAN_POINT ( 'NONE',  ( -54.48232515324713177, -2.803024266087990934, -2.239002676711937312 ) ) ;
#23360=ORIENTED_EDGE ( 'NONE', *, *, #27663, .F. ) ;
#23363=CARTESIAN_POINT ( 'NONE',  ( -55.43749999999997868, -3.399999999999991473, -2.094585006122325661E-13 ) ) ;
#23365=CARTESIAN_POINT ( 'NONE',  ( -59.41132486540517021, 2.413993528760422613, 1.250136525132548027 ) ) ;
#23372=CARTESIAN_POINT ( 'NONE',  ( -59.68966108275621707, -2.222588089596432059, 1.532842483073527884 ) ) ;
#23380=ORIENTED_EDGE ( 'NONE', *, *, #30832, .T. ) ;
#23393=CARTESIAN_POINT ( 'NONE',  ( -54.49999999999999289, -1.433333333333339343, 4.054078878802656938 ) ) ;
#23394=CARTESIAN_POINT ( 'NONE',  ( -56.08155989232414385, -1.962990915244736678, 3.399999999999788969 ) ) ;
#23402=CARTESIAN_POINT ( 'NONE',  ( -58.13452994616202574, 2.093608279459371404E-14, -3.600000000000206146 ) ) ;
#23403=( BOUNDED_CURVE ( )  B_SPLINE_CURVE ( 3, ( #28957, #16934, #26578, #2048 ),
 .UNSPECIFIED., .F., .T. ) 
 B_SPLINE_CURVE_WITH_KNOTS ( ( 4, 4 ),
 ( 5.204828459469180935, 5.421579857342605280 ),
 .UNSPECIFIED. ) 
 CURVE ( )  GEOMETRIC_REPRESENTATION_ITEM ( )  RATIONAL_B_SPLINE_CURVE ( ( 1.000000000000000000, 0.9960887331235708242, 0.9960887331235708242, 1.000000000000000000 ) ) 
 REPRESENTATION_ITEM ( '' )  );
#23416=CARTESIAN_POINT ( 'NONE',  ( -57.06249999999997868, -1.962990915244744006, 3.399999999999782307 ) ) ;
#23423=CARTESIAN_POINT ( 'NONE',  ( -59.31908585006426904, -2.449738638601608010, -1.018617722459757458 ) ) ;
#23461=CARTESIAN_POINT ( 'NONE',  ( -55.38452994616205416, -3.117691453623978148, 1.799999999999789102 ) ) ;
#23463=CARTESIAN_POINT ( 'NONE',  ( -58.14405989232411542, -2.944486372867076263, -1.700000000000216893 ) ) ;
#23468=CARTESIAN_POINT ( 'NONE',  ( -55.94702994616203995, -2.078460969082631227, -3.600000000000205258 ) ) ;
#23473=CARTESIAN_POINT ( 'NONE',  ( -54.49999999999997158, -0.6998428355231358644, -3.385667905176602321 ) ) ;
#23475=DIRECTION ( 'NONE',  ( -1.000000000000000000, 1.219044193948983948E-29, -3.491481338843133355E-15 ) ) ;
#23484=EDGE_CURVE ( 'NONE', #20201, #4847, #6692, .T. ) ;
#23491=CARTESIAN_POINT ( 'NONE',  ( -54.63452994616206126, -3.117691453623976816, 1.799999999999793765 ) ) ;
#23511=EDGE_CURVE ( 'NONE', #5493, #16551, #10202, .T. ) ;
#23512=CARTESIAN_POINT ( 'NONE',  ( -59.69999999999997442, 8.366749974758454467E-15, -2.120534355533670266E-13 ) ) ;
#23514=AXIS2_PLACEMENT_3D ( 'NONE', #18724, #16820, #9052 ) ;
#23515=CARTESIAN_POINT ( 'NONE',  ( -54.39999999999996305, 1.400000000000023892, -3.959797974644871932 ) ) ;
#23541=CARTESIAN_POINT ( 'NONE',  ( -54.39999999999996305, 1.433333333333357329, -4.054078878803077934 ) ) ;
#23543=ORIENTED_EDGE ( 'NONE', *, *, #21802, .T. ) ;
#23547=ORIENTED_EDGE ( 'NONE', *, *, #12096, .T. ) ;
#23553=CARTESIAN_POINT ( 'NONE',  ( -58.19702994616203284, -2.078460969082631227, -3.600000000000212363 ) ) ;
#23565=CARTESIAN_POINT ( 'NONE',  ( -55.58155989232413674, 3.400000000000007461, -1.857527951337884861E-13 ) ) ;
#23573=ORIENTED_EDGE ( 'NONE', *, *, #8280, .F. ) ;
#23574=AXIS2_PLACEMENT_3D ( 'NONE', #26090, #4403, #23734 ) ;
#23580=VECTOR ( 'NONE', #7491, 1000.000000000000000 ) ;
#23582=CARTESIAN_POINT ( 'NONE',  ( -59.51761855918061883, -2.467398989037727031, -1.133240635510040173 ) ) ;
#23586=CARTESIAN_POINT ( 'NONE',  ( -44.59999999999997300, -3.524999999999988365, -1.993951146718866637E-13 ) ) ;
#23605=CARTESIAN_POINT ( 'NONE',  ( -59.19999999999997442, 8.366749974758448157E-15, -2.103076948839454410E-13 ) ) ;
#23606=VECTOR ( 'NONE', #24187, 1000.000000000000000 ) ;
#23614=AXIS2_PLACEMENT_3D ( 'NONE', #6984, #25960, #8852 ) ;
#23615=DIRECTION ( 'NONE',  ( -1.000000000000000000, 0.000000000000000000, 8.673617379883787770E-15 ) ) ;
#23617=EDGE_LOOP ( 'NONE', ( #920, #22827, #27117, #13469 ) ) ;
#23628=ORIENTED_EDGE ( 'NONE', *, *, #794, .F. ) ;
#23631=ORIENTED_EDGE ( 'NONE', *, *, #25233, .F. ) ;
#23643=CARTESIAN_POINT ( 'NONE',  ( -61.24999999999995026, 2.023778652682512839E-14, -3.400000000000217515 ) ) ;
#23659=EDGE_CURVE ( 'NONE', #21890, #23000, #2960, .T. ) ;
#23666=DIRECTION ( 'NONE',  ( 0.000000000000000000, -1.000000000000000000, -6.156016597943509841E-15 ) ) ;
#23671=CARTESIAN_POINT ( 'NONE',  ( -59.12499999999996447, -2.944486372867076707, -1.700000000000220446 ) ) ;
#23689=DIRECTION ( 'NONE',  ( 0.000000000000000000, -1.000000000000000000, 0.000000000000000000 ) ) ;
#23695=CARTESIAN_POINT ( 'NONE',  ( -58.95655989232411542, -3.399999999999991029, -2.281093130107142867E-13 ) ) ;
#23701=ORIENTED_EDGE ( 'NONE', *, *, #8536, .T. ) ;
#23702=AXIS2_PLACEMENT_3D ( 'NONE', #25319, #24841, #22478 ) ;
#23708=CARTESIAN_POINT ( 'NONE',  ( -55.20655989232412963, -3.399999999999991473, -2.086450695418937968E-13 ) ) ;
#23710=ORIENTED_EDGE ( 'NONE', *, *, #21241, .T. ) ;
#23720=CYLINDRICAL_SURFACE ( 'NONE', #1119, 0.1000000000000000472 ) ;
#23724=CARTESIAN_POINT ( 'NONE',  ( -57.38452994616203284, 2.093608279459370457E-14, -3.600000000000203926 ) ) ;
#23734=DIRECTION ( 'NONE',  ( 0.000000000000000000, -1.000000000000000000, 0.000000000000000000 ) ) ;
#23746=CIRCLE ( 'NONE', #4015, 4.300000000000016698 ) ;
#23747=DIRECTION ( 'NONE',  ( 1.000000000000000000, -1.219044193948983948E-29, 3.491481338843133355E-15 ) ) ;
#23781=ORIENTED_EDGE ( 'NONE', *, *, #30008, .F. ) ;
#23793=CARTESIAN_POINT ( 'NONE',  ( -59.83155989232413674, -1.962990915244731571, 3.399999999999779199 ) ) ;
#23796=CIRCLE ( 'NONE', #21282, 3.625000000000024869 ) ;
#23797=CARTESIAN_POINT ( 'NONE',  ( -59.62499999999996447, 2.944486372867106905, -1.700000000000199130 ) ) ;
#23808=ORIENTED_EDGE ( 'NONE', *, *, #30295, .T. ) ;
#23809=CARTESIAN_POINT ( 'NONE',  ( -54.83155989232413674, 3.400000000000008349, -1.845326485282803322E-13 ) ) ;
#23817=AXIS2_PLACEMENT_3D ( 'NONE', #21863, #151, #26277 ) ;
#23823=CARTESIAN_POINT ( 'NONE',  ( -60.56249999999995026, -1.962990915244707368, -3.400000000000221956 ) ) ;
#23827=VERTEX_POINT ( 'NONE', #1485 ) ;
#23829=CARTESIAN_POINT ( 'NONE',  ( -56.00952994616203995, -3.117691453623963938, -1.800000000000210099 ) ) ;
#23830=VERTEX_POINT ( 'NONE', #1783 ) ;
#23840=ORIENTED_EDGE ( 'NONE', *, *, #22799, .T. ) ;
#23843=CARTESIAN_POINT ( 'NONE',  ( -58.61505354137800339, 3.400000000000014566, -0.9110272542660011741 ) ) ;
#23848=DIRECTION ( 'NONE',  ( 0.000000000000000000, 1.000000000000000000, 8.673617379884030739E-15 ) ) ;
#23854=ORIENTED_EDGE ( 'NONE', *, *, #23659, .F. ) ;
#23863=CARTESIAN_POINT ( 'NONE',  ( -44.59999999999998721, 1.399999999999998135, 3.363870538531280818 ) ) ;
#23864=ORIENTED_EDGE ( 'NONE', *, *, #19496, .T. ) ;
#23874=CARTESIAN_POINT ( 'NONE',  ( -56.94702994616206126, -2.078460969082657872, 3.599999999999789591 ) ) ;
#23902=CARTESIAN_POINT ( 'NONE',  ( -55.45655989232413674, 1.962990915244720247, 3.399999999999811173 ) ) ;
#23907=CARTESIAN_POINT ( 'NONE',  ( -44.59999999999997300, 3.624999999999963585, -1.915392816594897430E-13 ) ) ;
#23944=CARTESIAN_POINT ( 'NONE',  ( -59.99999999999997158, -2.944486372867089141, 1.699999999999775913 ) ) ;
#23950=ADVANCED_FACE ( 'NONE', ( #19542 ), #12098, .T. ) ;
#23959=( BOUNDED_CURVE ( )  B_SPLINE_CURVE ( 2, ( #5981, #3731, #15633, #13229, #11032, #1202, #10859, #20549, #18176 ),
 .UNSPECIFIED., .F., .T. ) 
 B_SPLINE_CURVE_WITH_KNOTS ( ( 3, 2, 2, 2, 3 ),
 ( 0.7554589434467710030, 0.7592592592592593004, 0.7777777777777777901, 0.7962962962962962798, 0.7991619333968115191 ),
 .UNSPECIFIED. ) 
 CURVE ( )  GEOMETRIC_REPRESENTATION_ITEM ( )  RATIONAL_B_SPLINE_CURVE ( ( 0.9562966789351563524, 0.9725061280706346345, 1.000000000000000000, 0.8660254037844387076, 1.000000000000000000, 0.8660254037844387076, 1.000000000000000000, 0.9792681810341394844, 0.9649526279839704124 ) ) 
 REPRESENTATION_ITEM ( '' )  );
#23968=VERTEX_POINT ( 'NONE', #5116 ) ;
#23972=CARTESIAN_POINT ( 'NONE',  ( -60.43749999999995026, 1.962990915244749557, -3.400000000000205969 ) ) ;
#23978=CARTESIAN_POINT ( 'NONE',  ( -58.38452994616204705, -3.117691453623976816, 1.799999999999780442 ) ) ;
#23989=ADVANCED_FACE ( 'NONE', ( #14912 ), #827, .T. ) ;
#23997=DIRECTION ( 'NONE',  ( -3.491481338843133355E-15, -3.491481338843133355E-15, 1.000000000000000000 ) ) ;
#23998=DIRECTION ( 'NONE',  ( -1.000000000000000000, 1.219044193948983948E-29, -3.491481338843133355E-15 ) ) ;
#24020=CARTESIAN_POINT ( 'NONE',  ( -56.70655989232412253, -3.925981830489445379, -2.155497846303743205E-13 ) ) ;
#24021=CARTESIAN_POINT ( 'NONE',  ( -59.25695844465221285, 3.255054294100257817, -0.9827484482200410376 ) ) ;
#24022=ADVANCED_FACE ( 'NONE', ( #15238 ), #24739, .T. ) ;
#24028=DIRECTION ( 'NONE',  ( -0.000000000000000000, 1.000000000000000000, 3.491481338843133355E-15 ) ) ;
#24029=CIRCLE ( 'NONE', #28061, 0.1000000000000001721 ) ;
#24048=DIRECTION ( 'NONE',  ( 0.000000000000000000, -1.000000000000000000, 0.000000000000000000 ) ) ;
#24054=CARTESIAN_POINT ( 'NONE',  ( -57.68749999999996447, -3.399999999999991029, -2.155011314204633625E-13 ) ) ;
#24061=TOROIDAL_SURFACE ( 'NONE', #796, 0.2000000000000000111, 0.1000000000000000056 ) ;
#24076=FACE_OUTER_BOUND ( 'NONE', #25067, .T. ) ;
#24082=ORIENTED_EDGE ( 'NONE', *, *, #29439, .T. ) ;
#24084=AXIS2_PLACEMENT_3D ( 'NONE', #20192, #13034, #18122 ) ;
#24090=ORIENTED_EDGE ( 'NONE', *, *, #20091, .T. ) ;
#24096=EDGE_LOOP ( 'NONE', ( #11147, #29587 ) ) ;
#24100=CARTESIAN_POINT ( 'NONE',  ( -60.06249999999997868, -1.962990915244731793, 3.399999999999778755 ) ) ;
#24113=CARTESIAN_POINT ( 'NONE',  ( -59.28559899066483041, 3.161828374300069466, 1.250136525132556020 ) ) ;
#24129=VERTEX_POINT ( 'NONE', #5900 ) ;
#24131=CARTESIAN_POINT ( 'NONE',  ( -56.82202994616205416, -4.156921938165296204, -2.167734102480683039E-13 ) ) ;
#24132=ORIENTED_EDGE ( 'NONE', *, *, #13301, .F. ) ;
#24135=CARTESIAN_POINT ( 'NONE',  ( -54.49999999999997868, -6.102218906431378987E-14, -2.216533082070118739E-13 ) ) ;
#24136=EDGE_LOOP ( 'NONE', ( #400, #15319, #29033, #28283 ) ) ;
#24138=CARTESIAN_POINT ( 'NONE',  ( -54.94702994616205416, 4.156921938165313080, -1.801810997602979365E-13 ) ) ;
#24142=CARTESIAN_POINT ( 'NONE',  ( -57.68749999999996447, -3.399999999999991029, -2.155011314204633625E-13 ) ) ;
#24155=( BOUNDED_CURVE ( )  B_SPLINE_CURVE ( 2, ( #23363, #11481, #11643, #11302, #30951, #6574, #20987, #18623, #16235 ),
 .UNSPECIFIED., .F., .T. ) 
 B_SPLINE_CURVE_WITH_KNOTS ( ( 3, 2, 2, 2, 3 ),
 ( 0.1388888888888888951, 0.1481481481481481399, 0.1666666666666666574, 0.1851851851851851749, 0.1944444444444444475 ),
 .UNSPECIFIED. ) 
 CURVE ( )  GEOMETRIC_REPRESENTATION_ITEM ( )  RATIONAL_B_SPLINE_CURVE ( ( 0.9330127018922192983, 0.9330127018922194093, 1.000000000000000000, 0.8660254037844387076, 1.000000000000000000, 0.8660254037844387076, 1.000000000000000000, 0.9330127018922191873, 0.9330127018922192983 ) ) 
 REPRESENTATION_ITEM ( '' )  );
#24170=DIRECTION ( 'NONE',  ( 3.491481338843133355E-15, 3.491481338843133355E-15, -1.000000000000000000 ) ) ;
#24172=ORIENTED_EDGE ( 'NONE', *, *, #21235, .T. ) ;
#24173=EDGE_CURVE ( 'NONE', #8534, #16069, #2263, .T. ) ;
#24186=CARTESIAN_POINT ( 'NONE',  ( -56.26905989232412963, 2.944486372867092250, 1.699999999999811218 ) ) ;
#24187=DIRECTION ( 'NONE',  ( -0.000000000000000000, 1.000000000000000000, 3.491481338843133355E-15 ) ) ;
#24197=ORIENTED_EDGE ( 'NONE', *, *, #15516, .F. ) ;
#24199=DIRECTION ( 'NONE',  ( -1.000000000000000000, 1.219044193948983948E-29, -3.491481338843133355E-15 ) ) ;
#24201=VERTEX_POINT ( 'NONE', #6521 ) ;
#24208=DIRECTION ( 'NONE',  ( -0.5000000000000029976, -3.023711536277451078E-15, 0.8660254037844369313 ) ) ;
#24209=ADVANCED_FACE ( 'NONE', ( #20785 ), #16180, .F. ) ;
#24218=CARTESIAN_POINT ( 'NONE',  ( -55.06249999999997158, 3.400000000000007905, -1.826733775103631524E-13 ) ) ;
#24221=FACE_OUTER_BOUND ( 'NONE', #4371, .T. ) ;
#24224=B_SPLINE_CURVE_WITH_KNOTS ( 'NONE', 3,
 ( #4113, #6497, #9027, #21079, #20766, #15986, #16155, #13436, #18541, #25648 ),
 .UNSPECIFIED., .F., .F.,
 ( 4, 3, 3, 4 ),
 ( 0.000000000000000000, 6.454972543172422090E-05, 0.0001290994513737798294, 0.0002445102546710338021 ),
 .UNSPECIFIED. ) ;
#24236=DIRECTION ( 'NONE',  ( -3.491481338843133355E-15, -3.491481338843133355E-15, 1.000000000000000000 ) ) ;
#24237=ORIENTED_EDGE ( 'NONE', *, *, #13405, .F. ) ;
#24239=DIRECTION ( 'NONE',  ( 0.000000000000000000, 1.000000000000000000, 3.491481338843130594E-15 ) ) ;
#24240=LINE ( 'NONE', #28979, #10026 ) ;
#24242=DIRECTION ( 'NONE',  ( -1.000000000000000000, 1.219044193948983948E-29, -3.491481338843133355E-15 ) ) ;
#24251=CARTESIAN_POINT ( 'NONE',  ( -59.63511902941204568, -2.173259666074455865, 1.527495276501993349 ) ) ;
#24261=CARTESIAN_POINT ( 'NONE',  ( -59.19702994616205416, -2.078460969082657872, 3.599999999999782041 ) ) ;
#24271=CARTESIAN_POINT ( 'NONE',  ( -59.69999999999997442, 8.366749974758454467E-15, -2.120534355533670266E-13 ) ) ;
#24279=EDGE_LOOP ( 'NONE', ( #17894, #20789, #23808, #9370 ) ) ;
#24285=CARTESIAN_POINT ( 'NONE',  ( -57.63452994616205416, -3.117691453623976816, 1.799999999999783329 ) ) ;
#24292=CARTESIAN_POINT ( 'NONE',  ( -54.82202994616206126, 2.078460969082646770, 3.599999999999812683 ) ) ;
#24302=CARTESIAN_POINT ( 'NONE',  ( -59.69999999999996021, 1.397030005794335672, -3.099726949734703751 ) ) ;
#24312=ORIENTED_EDGE ( 'NONE', *, *, #8784, .F. ) ;
#24319=CARTESIAN_POINT ( 'NONE',  ( -54.68749999999998579, -3.925981830489445379, -2.085002746943179415E-13 ) ) ;
#24321=EDGE_CURVE ( 'NONE', #16500, #18983, #4795, .T. ) ;
#24334=CARTESIAN_POINT ( 'NONE',  ( -55.33155989232414385, -1.962990915244731571, 3.399999999999794742 ) ) ;
#24339=DIRECTION ( 'NONE',  ( 1.000000000000000000, -1.219044193948983948E-29, 3.491481338843133355E-15 ) ) ;
#24347=DIRECTION ( 'NONE',  ( 1.000000000000000000, -1.219044193948983948E-29, 3.491481338843133355E-15 ) ) ;
#24360=DIRECTION ( 'NONE',  ( 1.000000000000000000, -1.219044193948983948E-29, 3.491481338843133355E-15 ) ) ;
#24366=AXIS2_PLACEMENT_3D ( 'NONE', #2015, #18968, #11680 ) ;
#24372=CARTESIAN_POINT ( 'NONE',  ( -44.59999999999999432, 1.399999999999995914, 3.959797974644454488 ) ) ;
#24376=DIRECTION ( 'NONE',  ( 0.000000000000000000, 1.000000000000000000, 3.491481338843133355E-15 ) ) ;
#24381=CARTESIAN_POINT ( 'NONE',  ( -44.59999999999995879, -1.499999999999978684, -4.029888335922158227 ) ) ;
#24388=DIRECTION ( 'NONE',  ( 0.000000000000000000, -1.000000000000000000, -3.491481338843137694E-15 ) ) ;
#24396=AXIS2_PLACEMENT_3D ( 'NONE', #9798, #6736, #23848 ) ;
#24402=VERTEX_POINT ( 'NONE', #19810 ) ;
#24403=CARTESIAN_POINT ( 'NONE',  ( -58.69702994616204705, 4.156921938165313080, -1.932741547809596393E-13 ) ) ;
#24409=DIRECTION ( 'NONE',  ( 0.000000000000000000, 1.000000000000000000, 3.491481338843130594E-15 ) ) ;
#24410=DIRECTION ( 'NONE',  ( 1.000000000000000000, -1.219044193948983948E-29, 3.491481338843133355E-15 ) ) ;
#24414=DIRECTION ( 'NONE',  ( 1.000000000000000000, -1.219044193948983948E-29, 3.491481338843133355E-15 ) ) ;
#24419=DIRECTION ( 'NONE',  ( -1.000000000000000000, 1.219044193948983948E-29, -3.491481338843133355E-15 ) ) ;
#24427=CARTESIAN_POINT ( 'NONE',  ( -59.69999999999997442, 8.366749974758454467E-15, -2.120534355533670266E-13 ) ) ;
#24428=ORIENTED_EDGE ( 'NONE', *, *, #11136, .T. ) ;
#24433=CARTESIAN_POINT ( 'NONE',  ( -54.88452994616206126, 3.117691453623979481, 1.799999999999816858 ) ) ;
#24434=VERTEX_POINT ( 'NONE', #19961 ) ;
#24437=DIRECTION ( 'NONE',  ( -1.000000000000000000, 1.219044193948983948E-29, -3.491481338843133355E-15 ) ) ;
#24438=CIRCLE ( 'NONE', #3703, 2.649999999999999911 ) ;
#24444=CARTESIAN_POINT ( 'NONE',  ( -59.51007810423286770, -3.208491484513371628, -1.128887151816144963 ) ) ;
#24445=DIRECTION ( 'NONE',  ( 0.000000000000000000, 1.000000000000000000, 3.491481338843130594E-15 ) ) ;
#24452=CIRCLE ( 'NONE', #27995, 0.1000000000000000472 ) ;
#24474=CARTESIAN_POINT ( 'NONE',  ( -56.45655989232411542, 1.962990915244748891, -3.400000000000191314 ) ) ;
#24491=DIRECTION ( 'NONE',  ( 0.000000000000000000, 1.000000000000000000, 3.491481338843130594E-15 ) ) ;
#24498=DIRECTION ( 'NONE',  ( -1.000000000000000000, 1.219044193948983948E-29, -3.491481338843133355E-15 ) ) ;
#24501=LINE ( 'NONE', #7874, #11995 ) ;
#24505=CARTESIAN_POINT ( 'NONE',  ( -55.31249999999995737, -1.962990915244704260, -3.400000000000204636 ) ) ;
#24527=FACE_OUTER_BOUND ( 'NONE', #19115, .T. ) ;
#24541=CARTESIAN_POINT ( 'NONE',  ( -59.61316801158443468, -2.161784001863006566, 1.533130796914948801 ) ) ;
#24549=CARTESIAN_POINT ( 'NONE',  ( -59.44702994616203995, 4.156921938165313080, -1.958927657850919798E-13 ) ) ;
#24550=DIRECTION ( 'NONE',  ( 1.000000000000000000, -1.219044193948983948E-29, 3.491481338843133355E-15 ) ) ;
#24569=CARTESIAN_POINT ( 'NONE',  ( -58.40400635094607651, -3.399999999999988365, -0.9110272542660473594 ) ) ;
#24583=CARTESIAN_POINT ( 'NONE',  ( -55.39405989232414385, -3.920666489018348300E-15, 3.399999999999801847 ) ) ;
#24587=ADVANCED_FACE ( 'NONE', ( #4332 ), #22388, .T. ) ;
#24601=EDGE_CURVE ( 'NONE', #22982, #13311, #12405, .T. ) ;
#24611=ORIENTED_EDGE ( 'NONE', *, *, #20695, .F. ) ;
#24620=CYLINDRICAL_SURFACE ( 'NONE', #20580, 0.1000000000000000472 ) ;
#24635=AXIS2_PLACEMENT_3D ( 'NONE', #13403, #26092, #18353 ) ;
#24637=CARTESIAN_POINT ( 'NONE',  ( -60.57202994616203995, -4.156921938165296204, -2.298664652687300067E-13 ) ) ;
#24643=CARTESIAN_POINT ( 'NONE',  ( -54.49999999999996447, -1.499999999999978906, -3.959797974644881258 ) ) ;
#24664=AXIS2_PLACEMENT_3D ( 'NONE', #22416, #559, #18149 ) ;
#24668=CARTESIAN_POINT ( 'NONE',  ( -57.86505354137801049, 3.400000000000013678, -0.9110272542659997308 ) ) ;
#24680=ADVANCED_FACE ( 'NONE', ( #9221 ), #22524, .T. ) ;
#24685=CARTESIAN_POINT ( 'NONE',  ( -56.75952994616203995, -3.117691453623960829, -1.800000000000218314 ) ) ;
#24703=CARTESIAN_POINT ( 'NONE',  ( -54.39999999999997726, 1.400000000000009681, -1.886605105831180521E-13 ) ) ;
#24712=CARTESIAN_POINT ( 'NONE',  ( -57.69702994616206126, -2.078460969082657872, 3.599999999999786926 ) ) ;
#24717=CARTESIAN_POINT ( 'NONE',  ( -58.76905989232410832, 2.523434546734629592E-14, -3.400000000000208189 ) ) ;
#24718=VECTOR ( 'NONE', #1546, 1000.000000000000000 ) ;
#24738=EDGE_CURVE ( 'NONE', #26017, #11119, #29098, .T. ) ;
#24739=CYLINDRICAL_SURFACE ( 'NONE', #20994, 3.399999999999999911 ) ;
#24744=STYLED_ITEM ( 'NONE', ( #25514 ), #12322 ) ;
#24749=CARTESIAN_POINT ( 'NONE',  ( -58.69702994616204705, 4.156921938165313080, -1.932741547809596393E-13 ) ) ;
#24764=EDGE_CURVE ( 'NONE', #27693, #30654, #19046, .T. ) ;
#24779=ORIENTED_EDGE ( 'NONE', *, *, #21039, .F. ) ;
#24783=( BOUNDED_CURVE ( )  B_SPLINE_CURVE ( 3, ( #3872, #10839, #11472, #11636 ),
 .UNSPECIFIED., .F., .T. ) 
 B_SPLINE_CURVE_WITH_KNOTS ( ( 4, 4 ),
 ( 1.079950260862541311, 1.195659917899331459 ),
 .UNSPECIFIED. ) 
 CURVE ( )  GEOMETRIC_REPRESENTATION_ITEM ( )  RATIONAL_B_SPLINE_CURVE ( ( 1.000000000000000000, 0.9988845841160336469, 0.9988845841160336469, 1.000000000000000000 ) ) 
 REPRESENTATION_ITEM ( '' )  );
#24791=CARTESIAN_POINT ( 'NONE',  ( -57.45655989232412963, -3.925981830489445379, -2.181683956345066863E-13 ) ) ;
#24802=VERTEX_POINT ( 'NONE', #11079 ) ;
#24819=CARTESIAN_POINT ( 'NONE',  ( -59.69577712845196515, 2.424301977118770157, -1.236100533437267890 ) ) ;
#24820=VERTEX_POINT ( 'NONE', #10762 ) ;
#24827=CARTESIAN_POINT ( 'NONE',  ( -54.88452994616206126, 3.117691453623979481, 1.799999999999816858 ) ) ;
#24830=( GEOMETRIC_REPRESENTATION_CONTEXT ( 3 ) GLOBAL_UNCERTAINTY_ASSIGNED_CONTEXT ( ( #26905 ) ) GLOBAL_UNIT_ASSIGNED_CONTEXT ( ( #437, #19768, #14365 ) ) REPRESENTATION_CONTEXT ( 'NONE', 'WORKASPACE' ) );
#24841=DIRECTION ( 'NONE',  ( -1.163827112947710461E-15, 0.9428090415820623571, 0.3333333333333364235 ) ) ;
#24845=LINE ( 'NONE', #10608, #7310 ) ;
#24849=CARTESIAN_POINT ( 'NONE',  ( -57.25952994616203995, 3.117691453623994580, -1.800000000000189671 ) ) ;
#24857=CARTESIAN_POINT ( 'NONE',  ( -56.25952994616206126, -4.643455692769913008E-15, 3.599999999999798916 ) ) ;
#24871=FACE_OUTER_BOUND ( 'NONE', #15648, .T. ) ;
#24879=ORIENTED_EDGE ( 'NONE', *, *, #3449, .T. ) ;
#24883=ORIENTED_EDGE ( 'NONE', *, *, #7742, .F. ) ;
#24888=ORIENTED_EDGE ( 'NONE', *, *, #17242, .F. ) ;
#24891=CARTESIAN_POINT ( 'NONE',  ( -55.64405989232412253, 2.944486372867106461, -1.700000000000184919 ) ) ;
#24904=EDGE_CURVE ( 'NONE', #18790, #31281, #23403, .T. ) ;
#24913=ORIENTED_EDGE ( 'NONE', *, *, #10059, .T. ) ;
#24914=LINE ( 'NONE', #12727, #30785 ) ;
#24923=EDGE_LOOP ( 'NONE', ( #19038, #16927, #23245, #23237 ) ) ;
#24932=ADVANCED_FACE ( 'NONE', ( #24221 ), #16308, .T. ) ;
#24935=CARTESIAN_POINT ( 'NONE',  ( -58.83155989232410832, -1.962990915244706924, -3.400000000000215294 ) ) ;
#24943=CARTESIAN_POINT ( 'NONE',  ( -59.28448904087081672, 2.425384292835127464, -1.073600088316289947 ) ) ;
#24970=DIRECTION ( 'NONE',  ( 0.000000000000000000, 1.000000000000000000, 3.491481338843130594E-15 ) ) ;
#24971=CARTESIAN_POINT ( 'NONE',  ( -59.69999999999996021, -1.369200569148549373, -3.341326691469316490 ) ) ;
#24972=ADVANCED_FACE ( 'NONE', ( #12180 ), #9665, .T. ) ;
#24981=CARTESIAN_POINT ( 'NONE',  ( -59.07202994616203995, -4.156921938165296204, -2.528906867826594094E-13 ) ) ;
#24984=VERTEX_POINT ( 'NONE', #7726 ) ;
#24985=CARTESIAN_POINT ( 'NONE',  ( -54.56249999999997158, -1.962990915244707146, -3.400000000000200640 ) ) ;
#24989=CARTESIAN_POINT ( 'NONE',  ( -54.49979136068852625, -2.172130796128893149, -2.794980562871907548 ) ) ;
#24996=CARTESIAN_POINT ( 'NONE',  ( -58.88452994616202574, 2.093608279459372350E-14, -3.600000000000208811 ) ) ;
#25007=EDGE_LOOP ( 'NONE', ( #8650, #12391, #28998 ) ) ;
#25009=CARTESIAN_POINT ( 'NONE',  ( -60.75952994616205416, -4.643455692769856999E-15, 3.599999999999783373 ) ) ;
#25013=CARTESIAN_POINT ( 'NONE',  ( -54.74999999999997868, -2.944486372867089141, 1.699999999999794342 ) ) ;
#25021=CARTESIAN_POINT ( 'NONE',  ( -59.67875522479140926, 2.062422519532147280, 1.724463576965509670 ) ) ;
#25029=ORIENTED_EDGE ( 'NONE', *, *, #30716, .F. ) ;
#25036=ORIENTED_EDGE ( 'NONE', *, *, #4640, .F. ) ;
#25044=CARTESIAN_POINT ( 'NONE',  ( -59.75952994616203284, -3.117691453623963938, -1.800000000000223199 ) ) ;
#25046=CARTESIAN_POINT ( 'NONE',  ( -54.39999999999999147, 1.514093959731539263, 3.183260039818149867 ) ) ;
#25048=ADVANCED_FACE ( 'NONE', ( #294 ), #24061, .T. ) ;
#25052=ORIENTED_EDGE ( 'NONE', *, *, #19873, .T. ) ;
#25054=CARTESIAN_POINT ( 'NONE',  ( -58.31249999999995026, -1.962990915244707368, -3.400000000000213518 ) ) ;
#25057=DIRECTION ( 'NONE',  ( 1.000000000000000000, -1.219044193948983948E-29, 3.491481338843133355E-15 ) ) ;
#25063=CARTESIAN_POINT ( 'NONE',  ( -54.49999999999997868, 8.366749974758391359E-15, -1.938977325913827332E-13 ) ) ;
#25067=EDGE_LOOP ( 'NONE', ( #31317, #30012, #22482 ) ) ;
#25077=CARTESIAN_POINT ( 'NONE',  ( -56.68749999999996447, 1.962990915244749557, -3.400000000000192646 ) ) ;
#25095=AXIS2_PLACEMENT_3D ( 'NONE', #25063, #11274, #3846 ) ;
#25096=CARTESIAN_POINT ( 'NONE',  ( -58.08155989232410832, -1.962990915244706924, -3.400000000000212630 ) ) ;
#25101=CARTESIAN_POINT ( 'NONE',  ( -59.19810431338756018, -2.425676737179530917, 1.249042049956554656 ) ) ;
#25118=CARTESIAN_POINT ( 'NONE',  ( -59.19834903927997516, -2.558621439192811930, -0.9489102922513534821 ) ) ;
#25120=ADVANCED_FACE ( 'NONE', ( #15653 ), #5867, .T. ) ;
#25123=CYLINDRICAL_SURFACE ( 'NONE', #26657, 2.649999999999999911 ) ;
#25142=CARTESIAN_POINT ( 'NONE',  ( -54.49999999999999289, -1.600000000000004530, 3.363870538531237298 ) ) ;
#25148=CARTESIAN_POINT ( 'NONE',  ( -44.59999999999997300, -6.102218906431391608E-14, -1.870876429524648473E-13 ) ) ;
#25156=CARTESIAN_POINT ( 'NONE',  ( -57.19702994616204705, 4.156921938165313968, -1.775982993694543137E-13 ) ) ;
#25159=ADVANCED_FACE ( 'NONE', ( #15797 ), #8805, .F. ) ;
#25162=CARTESIAN_POINT ( 'NONE',  ( -54.68749999999998579, -3.399999999999991029, -2.060885718922576431E-13 ) ) ;
#25166=CARTESIAN_POINT ( 'NONE',  ( -59.18122760499140611, 2.520598018727130629, -0.9442920350713964739 ) ) ;
#25174=CARTESIAN_POINT ( 'NONE',  ( -57.69702994616206126, -2.078460969082657872, 3.599999999999786926 ) ) ;
#25184=EDGE_LOOP ( 'NONE', ( #2318, #15096, #30576, #1494, #14770, #19163 ) ) ;
#25185=PLANE ( 'NONE',  #27906 ) ;
#25188=CARTESIAN_POINT ( 'NONE',  ( -54.99999999999997868, 2.944486372867092250, 1.699999999999816103 ) ) ;
#25204=ORIENTED_EDGE ( 'NONE', *, *, #2865, .F. ) ;
#25215=CARTESIAN_POINT ( 'NONE',  ( -59.07202994616203995, -4.156921938165296204, -2.246292432604653256E-13 ) ) ;
#25217=DIRECTION ( 'NONE',  ( -1.499696682456171775E-15, -0.9030524935654885565, 0.4295302013422961362 ) ) ;
#25223=CARTESIAN_POINT ( 'NONE',  ( -57.49999999999995737, 2.023778652682507790E-14, -3.400000000000204636 ) ) ;
#25233=EDGE_CURVE ( 'NONE', #2157, #24201, #1804, .T. ) ;
#25244=CARTESIAN_POINT ( 'NONE',  ( -54.99999999999997868, 2.944486372867092250, 1.699999999999816103 ) ) ;
#25248=DIRECTION ( 'NONE',  ( 0.000000000000000000, -1.000000000000000000, -3.491481338843137694E-15 ) ) ;
#25258=CARTESIAN_POINT ( 'NONE',  ( -58.01905989232410832, 2.023778652682508421E-14, -3.400000000000205969 ) ) ;
#25267=CARTESIAN_POINT ( 'NONE',  ( -59.46010231732345375, 3.229909594785855376, 1.334621550118761490 ) ) ;
#25272=EDGE_CURVE ( 'NONE', #11223, #10532, #461, .T. ) ;
#25290=ORIENTED_EDGE ( 'NONE', *, *, #1798, .F. ) ;
#25292=FACE_OUTER_BOUND ( 'NONE', #15469, .T. ) ;
#25300=CARTESIAN_POINT ( 'NONE',  ( -54.57202994616205416, -4.156921938165296204, -2.089175772356712570E-13 ) ) ;
#25308=CARTESIAN_POINT ( 'NONE',  ( -58.54806624327022746, 3.400000000000001688, 0.9110272542656313588 ) ) ;
#25310=ADVANCED_FACE ( 'NONE', ( #8294 ), #16998, .T. ) ;
#25311=CARTESIAN_POINT ( 'NONE',  ( -56.44702994616205416, 4.156921938165313968, -1.759978405944979146E-13 ) ) ;
#25319=CARTESIAN_POINT ( 'NONE',  ( -44.59999999999996589, 1.400000000000023670, -3.959797974644836405 ) ) ;
#25326=CARTESIAN_POINT ( 'NONE',  ( -60.50952994616203284, -3.117691453623963938, -1.800000000000225864 ) ) ;
#25347=CARTESIAN_POINT ( 'NONE',  ( -59.51024032614731851, 3.088598804228899652, 1.421463128792039843 ) ) ;
#25350=AXIS2_PLACEMENT_3D ( 'NONE', #19138, #28777, #7090 ) ;
#25365=ORIENTED_EDGE ( 'NONE', *, *, #22250, .T. ) ;
#25368=CARTESIAN_POINT ( 'NONE',  ( -58.01905989232410832, 2.023778652682508421E-14, -3.400000000000205969 ) ) ;
#25374=TOROIDAL_SURFACE ( 'NONE', #14253, 2.750000000000000000, 0.1000000000000000056 ) ;
#25375=CARTESIAN_POINT ( 'NONE',  ( -57.37499999999996447, 2.944486372867106905, -1.700000000000191136 ) ) ;
#25396=CARTESIAN_POINT ( 'NONE',  ( -56.56249999999997158, 3.925981830489463142, -1.866702293926226148E-13 ) ) ;
#25412=CARTESIAN_POINT ( 'NONE',  ( -60.58155989232412253, -1.962990915244731571, 3.399999999999776534 ) ) ;
#25413=EDGE_CURVE ( 'NONE', #11413, #7802, #2260, .T. ) ;
#25452=ORIENTED_EDGE ( 'NONE', *, *, #29897, .T. ) ;
#25477=CARTESIAN_POINT ( 'NONE',  ( -59.37758717751765403, 2.334345179268707771, 1.271211832739848280 ) ) ;
#25479=( BOUNDED_CURVE ( )  B_SPLINE_CURVE ( 2, ( #13389, #18194, #10729, #15650, #20567, #17556, #17869, #12780, #22460 ),
 .UNSPECIFIED., .F., .T. ) 
 B_SPLINE_CURVE_WITH_KNOTS ( ( 3, 2, 2, 2, 3 ),
 ( 0.03397538932574487025, 0.03703703703703703498, 0.05555555555555555247, 0.07407407407407406996, 0.08333333333333334259 ),
 .UNSPECIFIED. ) 
 CURVE ( )  GEOMETRIC_REPRESENTATION_ITEM ( )  RATIONAL_B_SPLINE_CURVE ( ( 0.9630242692063013532, 0.9778501171427680383, 1.000000000000000000, 0.8660254037844387076, 1.000000000000000000, 0.8660254037844387076, 1.000000000000000000, 0.9330127018922191873, 0.9330127018922192983 ) ) 
 REPRESENTATION_ITEM ( '' )  );
#25480=ADVANCED_FACE ( 'NONE', ( #19990 ), #17779, .T. ) ;
#25482=CARTESIAN_POINT ( 'NONE',  ( -60.94702994616203995, 4.156921938165313080, -2.011299877933566609E-13 ) ) ;
#25486=CARTESIAN_POINT ( 'NONE',  ( -59.59999999999997300, 2.337126060168390307, -1.249136413240100607 ) ) ;
#25501=EDGE_CURVE ( 'NONE', #30038, #6036, #9450, .T. ) ;
#25509=CARTESIAN_POINT ( 'NONE',  ( -44.59999999999998721, -1.400000000000006795, 3.959797974644484242 ) ) ;
#25514=PRESENTATION_STYLE_ASSIGNMENT (( #1452 ) ) ;
#25515=CARTESIAN_POINT ( 'NONE',  ( -54.50952994616204705, -3.117691453623963938, -1.800000000000204770 ) ) ;
#25516=CARTESIAN_POINT ( 'NONE',  ( -56.76905989232412963, -2.944486372867088697, 1.699999999999787015 ) ) ;
#25518=DIRECTION ( 'NONE',  ( 0.000000000000000000, 0.4295302013422958032, 0.9030524935654886676 ) ) ;
#25520=CARTESIAN_POINT ( 'NONE',  ( -57.56249999999995737, -1.962990915244707368, -3.400000000000210854 ) ) ;
#25535=ORIENTED_EDGE ( 'NONE', *, *, #2949, .T. ) ;
#25543=CARTESIAN_POINT ( 'NONE',  ( -57.93749999999998579, 1.962990915244722689, 3.399999999999801847 ) ) ;
#25545=ORIENTED_EDGE ( 'NONE', *, *, #13832, .T. ) ;
#25552=ORIENTED_EDGE ( 'NONE', *, *, #25413, .F. ) ;
#25561=CARTESIAN_POINT ( 'NONE',  ( -54.68749999999998579, -3.399999999999991029, -2.060885718922576431E-13 ) ) ;
#25587=ORIENTED_EDGE ( 'NONE', *, *, #7687, .T. ) ;
#25590=CYLINDRICAL_SURFACE ( 'NONE', #18599, 3.399999999999999911 ) ;
#25594=DIRECTION ( 'NONE',  ( 0.000000000000000000, -4.336808689942006692E-15, 1.000000000000000000 ) ) ;
#25595=CARTESIAN_POINT ( 'NONE',  ( -56.26905989232412963, 2.944486372867089585, 1.699999999999814992 ) ) ;
#25602=CARTESIAN_POINT ( 'NONE',  ( -57.32202994616202574, 2.078460969082674747, -3.600000000000194600 ) ) ;
#25606=( BOUNDED_CURVE ( )  B_SPLINE_CURVE ( 2, ( #22505, #27874, #22973, #977, #17910, #5714, #10629, #15218, #12996 ),
 .UNSPECIFIED., .F., .T. ) 
 B_SPLINE_CURVE_WITH_KNOTS ( ( 3, 2, 2, 2, 3 ),
 ( 0.3055555555555555802, 0.3148148148148148251, 0.3333333333333333148, 0.3518518518518518601, 0.3611111111111111605 ),
 .UNSPECIFIED. ) 
 CURVE ( )  GEOMETRIC_REPRESENTATION_ITEM ( )  RATIONAL_B_SPLINE_CURVE ( ( 0.9330127018922194093, 0.9330127018922195203, 1.000000000000000000, 0.8660254037844387076, 1.000000000000000000, 0.8660254037844387076, 1.000000000000000000, 0.9330127018922189652, 0.9330127018922194093 ) ) 
 REPRESENTATION_ITEM ( '' )  );
#25608=CARTESIAN_POINT ( 'NONE',  ( -54.49999999999996447, -1.399999999999981037, -3.363870538531691601 ) ) ;
#25620=LINE ( 'NONE', #3937, #13787 ) ;
#25630=CARTESIAN_POINT ( 'NONE',  ( -59.19999999999997442, -2.449420067797476452, 1.250136525132531817 ) ) ;
#25634=CIRCLE ( 'NONE', #28680, 0.1000000000000000749 ) ;
#25644=AXIS2_PLACEMENT_3D ( 'NONE', #30374, #15960, #3481 ) ;
#25645=CARTESIAN_POINT ( 'NONE',  ( -60.57202994616203995, -4.156921938165296204, -2.298664652687300067E-13 ) ) ;
#25648=CARTESIAN_POINT ( 'NONE',  ( -59.28559899066483041, 3.161828374300069466, 1.250136525132556020 ) ) ;
#25665=TOROIDAL_SURFACE ( 'NONE', #9516, 2.750000000000000000, 0.1000000000000000056 ) ;
#25670=ORIENTED_EDGE ( 'NONE', *, *, #18744, .T. ) ;
#25673=SHAPE_REPRESENTATION ( 'Rotator Head', ( #9018 ), #5016 ) ;
#25684=CARTESIAN_POINT ( 'NONE',  ( -57.45655989232412963, -3.925981830489445379, -2.181683956345066863E-13 ) ) ;
#25689=CARTESIAN_POINT ( 'NONE',  ( -55.12499999999997158, 2.944486372867106905, -1.700000000000183364 ) ) ;
#25694=DIRECTION ( 'NONE',  ( 0.000000000000000000, 1.000000000000000000, 3.491481338843130594E-15 ) ) ;
#25700=CARTESIAN_POINT ( 'NONE',  ( -59.66272163888239533, -2.194198658389501677, 1.525022448910328121 ) ) ;
#25707=EDGE_CURVE ( 'NONE', #24984, #28363, #10554, .T. ) ;
#25712=CARTESIAN_POINT ( 'NONE',  ( -56.37499999999998579, -3.920666489018338045E-15, 3.399999999999799183 ) ) ;
#25727=ORIENTED_EDGE ( 'NONE', *, *, #17397, .F. ) ;
#25737=PLANE ( 'NONE',  #21594 ) ;
#25749=VERTEX_POINT ( 'NONE', #15622 ) ;
#25759=CIRCLE ( 'NONE', #2512, 0.1000000000000003803 ) ;
#25761=LINE ( 'NONE', #18017, #10519 ) ;
#25764=ORIENTED_EDGE ( 'NONE', *, *, #2449, .T. ) ;
#25770=CARTESIAN_POINT ( 'NONE',  ( -59.19702994616205416, -2.078460969082657872, 3.599999999999782041 ) ) ;
#25772=EDGE_CURVE ( 'NONE', #11223, #11810, #860, .T. ) ;
#25776=CARTESIAN_POINT ( 'NONE',  ( -59.41132486540516311, 2.423250918913632201, 1.250136525132548027 ) ) ;
#25792=CARTESIAN_POINT ( 'NONE',  ( -61.07202994616202574, 2.078460969082674747, -3.600000000000208367 ) ) ;
#25799=FACE_OUTER_BOUND ( 'NONE', #20029, .T. ) ;
#25809=AXIS2_PLACEMENT_3D ( 'NONE', #19854, #24437, #15093 ) ;
#25813=CARTESIAN_POINT ( 'NONE',  ( -59.40362242792826919, 3.375967812128700452, 1.250136525132546916 ) ) ;
#25819=DIRECTION ( 'NONE',  ( 0.000000000000000000, -1.000000000000000000, -3.491481338843133355E-15 ) ) ;
#25823=ORIENTED_EDGE ( 'NONE', *, *, #20965, .T. ) ;
#25834=CARTESIAN_POINT ( 'NONE',  ( -54.63452994616206126, -3.117691453623976816, 1.799999999999793765 ) ) ;
#25835=CARTESIAN_POINT ( 'NONE',  ( -57.14405989232411542, 2.944486372867106461, -1.700000000000190248 ) ) ;
#25841=CARTESIAN_POINT ( 'NONE',  ( -55.75952994616203995, 3.117691453623994580, -1.800000000000184563 ) ) ;
#25843=CARTESIAN_POINT ( 'NONE',  ( -55.08155989232412253, -1.962990915244704260, -3.400000000000203748 ) ) ;
#25866=CARTESIAN_POINT ( 'NONE',  ( -55.57202994616207548, 2.078460969082646770, 3.599999999999810019 ) ) ;
#25872=LINE ( 'NONE', #26020, #22760 ) ;
#25915=ORIENTED_EDGE ( 'NONE', *, *, #5560, .F. ) ;
#25918=CARTESIAN_POINT ( 'NONE',  ( -59.40619059199517693, 3.371123259826405594, 1.250136525132546694 ) ) ;
#25919=CARTESIAN_POINT ( 'NONE',  ( -44.59999999999997300, 8.366749974758367693E-15, -1.870876429524646202E-13 ) ) ;
#25920=CARTESIAN_POINT ( 'NONE',  ( -56.32202994616206126, 2.078460969082646770, 3.599999999999807354 ) ) ;
#25933=ORIENTED_EDGE ( 'NONE', *, *, #31168, .T. ) ;
#25937=CARTESIAN_POINT ( 'NONE',  ( -57.68749999999996447, -3.399999999999991029, -2.155011314204633625E-13 ) ) ;
#25952=CARTESIAN_POINT ( 'NONE',  ( -44.59999999999995879, 1.400000000000023892, -4.029888335922147569 ) ) ;
#25960=DIRECTION ( 'NONE',  ( -3.491481338843133355E-15, -3.491481338843133355E-15, 1.000000000000000000 ) ) ;
#25972=CARTESIAN_POINT ( 'NONE',  ( -56.33155989232412963, 3.400000000000008349, -1.856946929144785632E-13 ) ) ;
#25974=ORIENTED_EDGE ( 'NONE', *, *, #2930, .F. ) ;
#25985=CARTESIAN_POINT ( 'NONE',  ( -57.01905989232412963, 2.944486372867092250, 1.699999999999808553 ) ) ;
#25987=CARTESIAN_POINT ( 'NONE',  ( 0.000000000000000000, 0.000000000000000000, 0.000000000000000000 ) ) ;
#25989=AXIS2_PLACEMENT_3D ( 'NONE', #31324, #24208, #11850 ) ;
#25992=CARTESIAN_POINT ( 'NONE',  ( -55.88452994616203995, 2.093608279459368564E-14, -3.600000000000198597 ) ) ;
#26000=CARTESIAN_POINT ( 'NONE',  ( -44.49999999999997868, -6.102218906431391608E-14, -1.867384948185805656E-13 ) ) ;
#26004=DIRECTION ( 'NONE',  ( 0.000000000000000000, -1.000000000000000000, 0.000000000000000000 ) ) ;
#26009=CARTESIAN_POINT ( 'NONE',  ( -54.49999999999996447, 1.433333333333357329, -4.054078878803077934 ) ) ;
#26015=CARTESIAN_POINT ( 'NONE',  ( -55.13452994616203995, 2.093608279459367933E-14, -3.600000000000195932 ) ) ;
#26016=ORIENTED_EDGE ( 'NONE', *, *, #2865, .T. ) ;
#26017=VERTEX_POINT ( 'NONE', #3390 ) ;
#26020=CARTESIAN_POINT ( 'NONE',  ( -54.49999999999996447, 1.400000000000023892, -4.029888335922182208 ) ) ;
#26071=VERTEX_POINT ( 'NONE', #23329 ) ;
#26076=CARTESIAN_POINT ( 'NONE',  ( -58.32202994616204705, -4.156921938165296204, -2.220106322563329850E-13 ) ) ;
#26086=AXIS2_PLACEMENT_3D ( 'NONE', #25142, #13565, #3921 ) ;
#26090=CARTESIAN_POINT ( 'NONE',  ( -44.59999999999996589, -1.399999999999979039, -3.959797974644846619 ) ) ;
#26092=DIRECTION ( 'NONE',  ( -1.000000000000000000, -0.000000000000000000, 0.000000000000000000 ) ) ;
#26096=CARTESIAN_POINT ( 'NONE',  ( -54.49999999999997868, -3.188085654472696540, 1.181570928782897267 ) ) ;
#26100=CIRCLE ( 'NONE', #12438, 0.2000000000000000944 ) ;
#26101=VERTEX_POINT ( 'NONE', #4001 ) ;
#26102=CARTESIAN_POINT ( 'NONE',  ( -59.64457535546588218, -2.323701065654765419, -1.273936166954769300 ) ) ;
#26112=CIRCLE ( 'NONE', #19559, 3.524999999999996358 ) ;
#26128=CARTESIAN_POINT ( 'NONE',  ( -44.49999999999996447, -1.599999999999981215, -3.363870538531657406 ) ) ;
#26147=VERTEX_POINT ( 'NONE', #19370 ) ;
#26149=VECTOR ( 'NONE', #22665, 1000.000000000000000 ) ;
#26162=CARTESIAN_POINT ( 'NONE',  ( -60.43749999999995026, 1.962990915244749557, -3.400000000000205969 ) ) ;
#26190=CARTESIAN_POINT ( 'NONE',  ( -59.87499999999995737, -2.944486372867076707, -1.700000000000223332 ) ) ;
#26193=CARTESIAN_POINT ( 'NONE',  ( -59.58615951392652477, 3.226516192400048055, -1.172812774183070283 ) ) ;
#26196=CARTESIAN_POINT ( 'NONE',  ( -57.32202994616202574, 2.078460969082674747, -3.600000000000194600 ) ) ;
#26205=DIRECTION ( 'NONE',  ( 0.000000000000000000, -1.000000000000000000, -4.336808689942015369E-15 ) ) ;
#26208=DIRECTION ( 'NONE',  ( 0.000000000000000000, -0.4295302013423027421, 0.9030524935654852259 ) ) ;
#26210=CARTESIAN_POINT ( 'NONE',  ( -58.89405989232411542, -2.944486372867071822, -1.700000000000227107 ) ) ;
#26223=DIRECTION ( 'NONE',  ( 0.000000000000000000, -1.000000000000000000, -3.491481338843132961E-15 ) ) ;
#26239=DIRECTION ( 'NONE',  ( 3.491481338843133355E-15, 3.491481338843133355E-15, -1.000000000000000000 ) ) ;
#26241=CARTESIAN_POINT ( 'NONE',  ( -56.13452994616205416, -3.117691453623976816, 1.799999999999788436 ) ) ;
#26242=CARTESIAN_POINT ( 'NONE',  ( -59.18632331196522500, -2.527880932825658178, -0.9441059845029629027 ) ) ;
#26244=EDGE_CURVE ( 'NONE', #24129, #7345, #7174, .T. ) ;
#26250=CARTESIAN_POINT ( 'NONE',  ( -55.76905989232411542, 2.190330617366546077E-14, -3.400000000000197975 ) ) ;
#26251=CIRCLE ( 'NONE', #7058, 0.2000000000000000944 ) ;
#26257=EDGE_CURVE ( 'NONE', #5886, #14413, #10636, .T. ) ;
#26277=DIRECTION ( 'NONE',  ( 0.000000000000000000, -1.000000000000000000, -3.491481338843136511E-15 ) ) ;
#26287=AXIS2_PLACEMENT_3D ( 'NONE', #12498, #29296, #22185 ) ;
#26290=CARTESIAN_POINT ( 'NONE',  ( -59.64457535546588929, 2.323701065654787623, -1.273936166954758642 ) ) ;
#26295=CARTESIAN_POINT ( 'NONE',  ( -59.60304182990236654, 2.022940613791669673, 1.711857625294797680 ) ) ;
#26321=CARTESIAN_POINT ( 'NONE',  ( -55.19702994616203284, -2.078460969082631227, -3.600000000000202593 ) ) ;
#26324=DIRECTION ( 'NONE',  ( -1.000000000000000000, 1.219044193948983948E-29, -3.491481338843133355E-15 ) ) ;
#26343=CARTESIAN_POINT ( 'NONE',  ( -59.31249999999997868, -1.962990915244731793, 3.399999999999781419 ) ) ;
#26349=EDGE_CURVE ( 'NONE', #16856, #7637, #25606, .T. ) ;
#26351=CARTESIAN_POINT ( 'NONE',  ( -56.50952994616203995, 3.117691453623994580, -1.800000000000187006 ) ) ;
#26376=ORIENTED_EDGE ( 'NONE', *, *, #31282, .T. ) ;
#26380=FACE_OUTER_BOUND ( 'NONE', #18484, .T. ) ;
#26396=CARTESIAN_POINT ( 'NONE',  ( -61.07202994616202574, 2.078460969082674747, -3.600000000000208367 ) ) ;
#26413=FACE_OUTER_BOUND ( 'NONE', #20945, .T. ) ;
#26468=CARTESIAN_POINT ( 'NONE',  ( -55.32202994616205416, -4.156921938165296204, -2.115361882398036228E-13 ) ) ;
#26474=CARTESIAN_POINT ( 'NONE',  ( -59.39247302616080049, -3.117158037005095750, 1.361260878598222757 ) ) ;
#26488=CARTESIAN_POINT ( 'NONE',  ( -59.69999999999997442, 3.400000000000007905, -2.001823990013003858E-13 ) ) ;
#26492=CARTESIAN_POINT ( 'NONE',  ( -56.32202994616206126, 2.078460969082646770, 3.599999999999807354 ) ) ;
#26498=CARTESIAN_POINT ( 'NONE',  ( -56.44702994616204705, 4.156921938165313080, -1.854183217685626176E-13 ) ) ;
#26501=CARTESIAN_POINT ( 'NONE',  ( -59.36488781976483864, -2.508594352967794983, -1.045061501994807296 ) ) ;
#26505=( BOUNDED_CURVE ( )  B_SPLINE_CURVE ( 2, ( #12743, #15284, #10693, #22421, #12896, #887, #17512, #22746, #3575 ),
 .UNSPECIFIED., .F., .T. ) 
 B_SPLINE_CURVE_WITH_KNOTS ( ( 3, 2, 2, 2, 3 ),
 ( 0.6388888888888889506, 0.6481481481481481399, 0.6666666666666666297, 0.6851851851851852304, 0.6944444444444445308 ),
 .UNSPECIFIED. ) 
 CURVE ( )  GEOMETRIC_REPRESENTATION_ITEM ( )  RATIONAL_B_SPLINE_CURVE ( ( 0.9330127018922194093, 0.9330127018922197424, 1.000000000000000000, 0.8660254037844387076, 1.000000000000000000, 0.8660254037844387076, 1.000000000000000000, 0.9330127018922189652, 0.9330127018922194093 ) ) 
 REPRESENTATION_ITEM ( '' )  );
#26506=DIRECTION ( 'NONE',  ( -1.000000000000000000, 1.219044193948983948E-29, -3.491481338843133355E-15 ) ) ;
#26508=ORIENTED_EDGE ( 'NONE', *, *, #18373, .F. ) ;
#26544=CARTESIAN_POINT ( 'NONE',  ( -55.20655989232412963, -3.925981830489445379, -2.103125626221096647E-13 ) ) ;
#26545=CARTESIAN_POINT ( 'NONE',  ( -59.19151862111560547, -2.538026038378716542, -0.9449667484854825661 ) ) ;
#26546=CARTESIAN_POINT ( 'NONE',  ( -58.74999999999997158, 2.944486372867083368, 1.699999999999819655 ) ) ;
#26553=ORIENTED_EDGE ( 'NONE', *, *, #2325, .T. ) ;
#26565=B_SPLINE_CURVE_WITH_KNOTS ( 'NONE', 3,
 ( #1171, #29837, #874, #10533, #10826, #8149, #17337, #29985, #5290, #12577, #5622, #20036, #7678 ),
 .UNSPECIFIED., .F., .F.,
 ( 4, 3, 3, 3, 4 ),
 ( -2.000024084956990982E-06, 0.000000000000000000, 4.241049103993853043E-05, 9.571654392116296867E-05, 0.0001361917980506076374 ),
 .UNSPECIFIED. ) ;
#26570=CARTESIAN_POINT ( 'NONE',  ( -59.69313819382897179, 2.416215365816545724, -1.234576943822310424 ) ) ;
#26574=DIRECTION ( 'NONE',  ( 0.000000000000000000, -0.4295302013422799270, -0.9030524935654961061 ) ) ;
#26578=CARTESIAN_POINT ( 'NONE',  ( -59.60741592600796679, 2.216588895794640912, 1.589776205006679266 ) ) ;
#26581=AXIS2_PLACEMENT_3D ( 'NONE', #17995, #5642, #5491 ) ;
#26593=CARTESIAN_POINT ( 'NONE',  ( -59.50169947458163477, 2.403253767585081579, -1.124049747732222659 ) ) ;
#26596=CARTESIAN_POINT ( 'NONE',  ( -54.49999999999999289, 1.399999999999998357, 3.300094695610798823 ) ) ;
#26603=PLANE ( 'NONE',  #11053 ) ;
#26612=ADVANCED_FACE ( 'NONE', ( #11572 ), #11499, .T. ) ;
#26626=ADVANCED_FACE ( 'NONE', ( #10559 ), #8593, .T. ) ;
#26629=VECTOR ( 'NONE', #10563, 1000.000000000000000 ) ;
#26630=CARTESIAN_POINT ( 'NONE',  ( -57.44702994616203284, -2.078460969082631227, -3.600000000000210587 ) ) ;
#26634=DIRECTION ( 'NONE',  ( -3.491481338843133355E-15, -3.491481338843133355E-15, 1.000000000000000000 ) ) ;
#26636=ADVANCED_FACE ( 'NONE', ( #20071 ), #19334, .T. ) ;
#26657=AXIS2_PLACEMENT_3D ( 'NONE', #15784, #20712, #21012 ) ;
#26662=CARTESIAN_POINT ( 'NONE',  ( -59.44702994616203995, 4.156921938165313080, -1.958927657850919798E-13 ) ) ;
#26667=ORIENTED_EDGE ( 'NONE', *, *, #24904, .F. ) ;
#26671=CARTESIAN_POINT ( 'NONE',  ( -56.25952994616206126, -4.643455692769913008E-15, 3.599999999999798916 ) ) ;
#26672=ORIENTED_EDGE ( 'NONE', *, *, #29676, .F. ) ;
#26673=CARTESIAN_POINT ( 'NONE',  ( -56.52900635094608361, 3.400000000000004352, 0.9110272542656328021 ) ) ;
#26675=CIRCLE ( 'NONE', #12998, 0.1000000000000001166 ) ;
#26676=DIRECTION ( 'NONE',  ( 3.491481338843133355E-15, 3.491481338843133355E-15, -1.000000000000000000 ) ) ;
#26706=ORIENTED_EDGE ( 'NONE', *, *, #13301, .T. ) ;
#26723=CARTESIAN_POINT ( 'NONE',  ( -60.32202994616201863, 2.078460969082674747, -3.600000000000205258 ) ) ;
#26729=CARTESIAN_POINT ( 'NONE',  ( -59.69999999999997442, 8.366749974758454467E-15, -2.120534355533670266E-13 ) ) ;
#26737=ORIENTED_EDGE ( 'NONE', *, *, #29511, .F. ) ;
#26747=ORIENTED_EDGE ( 'NONE', *, *, #18427, .T. ) ;
#26755=CARTESIAN_POINT ( 'NONE',  ( -57.72099364905386665, -3.399999999999994138, 0.9110272542655947214 ) ) ;
#26762=CARTESIAN_POINT ( 'NONE',  ( -59.47497210890824704, 3.405470396758961904, -1.108618695965261969 ) ) ;
#26765=CARTESIAN_POINT ( 'NONE',  ( -59.19495429951913223, -2.548385458854336871, -0.9469503383366065785 ) ) ;
#26772=CARTESIAN_POINT ( 'NONE',  ( -59.59999999999998010, 8.366749974758452890E-15, -2.117042874194827196E-13 ) ) ;
#26775=ORIENTED_EDGE ( 'NONE', *, *, #19496, .F. ) ;
#26784=CARTESIAN_POINT ( 'NONE',  ( -60.51905989232411542, -2.944486372867088697, 1.699999999999773914 ) ) ;
#26787=VECTOR ( 'NONE', #18011, 1000.000000000000000 ) ;
#26789=CARTESIAN_POINT ( 'NONE',  ( -60.07202994616204705, 2.078460969082646770, 3.599999999999794031 ) ) ;
#26801=CARTESIAN_POINT ( 'NONE',  ( -44.49999999999996447, -1.514093959731525496, -3.183260039818558429 ) ) ;
#26806=CARTESIAN_POINT ( 'NONE',  ( -59.69999999999997442, 8.366749974758454467E-15, -2.120534355533670266E-13 ) ) ;
#26817=CARTESIAN_POINT ( 'NONE',  ( -57.44702994616203284, -2.078460969082631227, -3.600000000000210587 ) ) ;
#26838=EDGE_LOOP ( 'NONE', ( #14615, #1409, #625, #5158 ) ) ;
#26846=ORIENTED_EDGE ( 'NONE', *, *, #28595, .T. ) ;
#26852=CIRCLE ( 'NONE', #9162, 0.1000000000000000472 ) ;
#26854=EDGE_CURVE ( 'NONE', #21024, #6022, #15772, .T. ) ;
#26857=CARTESIAN_POINT ( 'NONE',  ( -55.83155989232411542, -1.962990915244706924, -3.400000000000204636 ) ) ;
#26861=MECHANICAL_DESIGN_GEOMETRIC_PRESENTATION_REPRESENTATION('',(#1084),#24830);
#26863=FACE_OUTER_BOUND ( 'NONE', #5009, .T. ) ;
#26873=DIRECTION ( 'NONE',  ( 1.000000000000000000, -1.219044193948983948E-29, 3.491481338843133355E-15 ) ) ;
#26901=EDGE_CURVE ( 'NONE', #4064, #27932, #4354, .T. ) ;
#26905=UNCERTAINTY_MEASURE_WITH_UNIT (LENGTH_MEASURE( 1.000000000000000082E-05 ), #437, 'distance_accuracy_value', 'NONE');
#26916=DIRECTION ( 'NONE',  ( 0.000000000000000000, 1.000000000000000000, 3.491481338843252079E-15 ) ) ;
#26925=ORIENTED_EDGE ( 'NONE', *, *, #27206, .T. ) ;
#26926=CARTESIAN_POINT ( 'NONE',  ( -57.94702994616203995, 4.156921938165313080, -1.906555437768272735E-13 ) ) ;
#26938=DIRECTION ( 'NONE',  ( 1.000000000000000000, -1.219044193948983948E-29, 3.491481338843133355E-15 ) ) ;
#26940=EDGE_CURVE ( 'NONE', #26017, #28731, #28190, .T. ) ;
#26948=DIRECTION ( 'NONE',  ( 1.000000000000000000, -1.219044193948983948E-29, 3.491481338843133355E-15 ) ) ;
#26952=ORIENTED_EDGE ( 'NONE', *, *, #14032, .T. ) ;
#26957=CARTESIAN_POINT ( 'NONE',  ( -60.19702994616203995, 4.156921938165313080, -1.985113767892243204E-13 ) ) ;
#26983=DIRECTION ( 'NONE',  ( 0.000000000000000000, -1.000000000000000000, -3.491481338843131383E-15 ) ) ;
#26984=PRODUCT ( 'Rotator Head', 'Rotator Head', '', ( #20442 ) ) ;
#26988=ORIENTED_EDGE ( 'NONE', *, *, #28754, .F. ) ;
#26993=EDGE_CURVE ( 'NONE', #20519, #1750, #1821, .T. ) ;
#26995=ORIENTED_EDGE ( 'NONE', *, *, #5206, .T. ) ;
#26997=CARTESIAN_POINT ( 'NONE',  ( -57.14405989232411542, 2.944486372867110457, -1.700000000000182920 ) ) ;
#27000=CARTESIAN_POINT ( 'NONE',  ( -60.82202994616204705, 2.078460969082646770, 3.599999999999791367 ) ) ;
#27034=CARTESIAN_POINT ( 'NONE',  ( -59.69999999999994600, 0.04532186801287400868, -3.495089302298031608 ) ) ;
#27039=ORIENTED_EDGE ( 'NONE', *, *, #14792, .T. ) ;
#27045=CARTESIAN_POINT ( 'NONE',  ( -59.45343688171008267, 3.370349218368761779, -1.096185326745346078 ) ) ;
#27053=ORIENTED_EDGE ( 'NONE', *, *, #16399, .F. ) ;
#27054=DIRECTION ( 'NONE',  ( 0.000000000000000000, -1.000000000000000000, -3.491481338843133355E-15 ) ) ;
#27055=CARTESIAN_POINT ( 'NONE',  ( -54.48976431536610932, -2.364211421526874357, -2.673742973752935903 ) ) ;
#27061=CARTESIAN_POINT ( 'NONE',  ( -59.20655989232412963, 1.962990915244715806, 3.399999999999800071 ) ) ;
#27065=CYLINDRICAL_SURFACE ( 'NONE', #2885, 0.1000000000000000472 ) ;
#27073=AXIS2_PLACEMENT_3D ( 'NONE', #6236, #10823, #30296 ) ;
#27075=ADVANCED_FACE ( 'NONE', ( #544, #20024 ), #14791, .F. ) ;
#27078=CARTESIAN_POINT ( 'NONE',  ( -59.94702994616205416, -2.078460969082657872, 3.599999999999778932 ) ) ;
#27084=CARTESIAN_POINT ( 'NONE',  ( -58.70655989232410832, 1.962990915244761991, -3.400000000000191314 ) ) ;
#27087=VECTOR ( 'NONE', #24339, 1000.000000000000000 ) ;
#27116=CARTESIAN_POINT ( 'NONE',  ( -58.82202994616202574, 2.078460969082674747, -3.600000000000199929 ) ) ;
#27117=ORIENTED_EDGE ( 'NONE', *, *, #9841, .F. ) ;
#27121=DIRECTION ( 'NONE',  ( -1.000000000000000000, 0.000000000000000000, -3.491481338843153471E-15 ) ) ;
#27143=CARTESIAN_POINT ( 'NONE',  ( -54.49999999999999289, 1.599999999999998090, 3.363870538531247067 ) ) ;
#27150=AXIS2_PLACEMENT_3D ( 'NONE', #15410, #25057, #24445 ) ;
#27157=EDGE_LOOP ( 'NONE', ( #9645, #10541, #14504, #8567, #14589, #27930 ) ) ;
#27160=CYLINDRICAL_SURFACE ( 'NONE', #24664, 3.399999999999999911 ) ;
#27170=CARTESIAN_POINT ( 'NONE',  ( -60.70655989232412963, 1.962990915244722245, 3.399999999999792077 ) ) ;
#27178=FACE_OUTER_BOUND ( 'NONE', #6812, .T. ) ;
#27206=EDGE_CURVE ( 'NONE', #31281, #2592, #14757, .T. ) ;
#27216=EDGE_CURVE ( 'NONE', #20056, #19660, #27767, .T. ) ;
#27221=ORIENTED_EDGE ( 'NONE', *, *, #9451, .F. ) ;
#27222=DIRECTION ( 'NONE',  ( 0.000000000000000000, -1.000000000000000000, -4.336808689942025625E-15 ) ) ;
#27224=UNCERTAINTY_MEASURE_WITH_UNIT (LENGTH_MEASURE( 1.000000000000000082E-05 ), #21276, 'distance_accuracy_value', 'NONE');
#27226=CARTESIAN_POINT ( 'NONE',  ( -54.48711142618073211, -2.373575576312949131, -2.672219526802753098 ) ) ;
#27236=CARTESIAN_POINT ( 'NONE',  ( -57.94702994616203995, 4.156921938165313080, -1.906555437768272735E-13 ) ) ;
#27239=DIRECTION ( 'NONE',  ( 0.000000000000000000, -1.000000000000000000, 0.000000000000000000 ) ) ;
#27245=CARTESIAN_POINT ( 'NONE',  ( -58.82202994616202574, 2.078460969082674747, -3.600000000000199929 ) ) ;
#27261=DIRECTION ( 'NONE',  ( 0.000000000000000000, -1.000000000000000000, -4.336808689942015369E-15 ) ) ;
#27264=CARTESIAN_POINT ( 'NONE',  ( -44.59999999999997300, 8.366749974758271452E-15, -1.593320673368357066E-13 ) ) ;
#27280=CARTESIAN_POINT ( 'NONE',  ( -55.26905989232413674, -2.944486372867088697, 1.699999999999792344 ) ) ;
#27282=DIRECTION ( 'NONE',  ( -1.000000000000000000, 1.219044193948983948E-29, -3.491481338843133355E-15 ) ) ;
#27286=ORIENTED_EDGE ( 'NONE', *, *, #16399, .T. ) ;
#27299=AXIS2_PLACEMENT_3D ( 'NONE', #21904, #19675, #2575 ) ;
#27302=CARTESIAN_POINT ( 'NONE',  ( -59.69557399992023505, -2.421670674729428985, -1.235983257124811274 ) ) ;
#27324=CARTESIAN_POINT ( 'NONE',  ( -57.01905989232412963, 2.944486372867092250, 1.699999999999808553 ) ) ;
#27332=CARTESIAN_POINT ( 'NONE',  ( -59.31739128601933686, -2.302762792303276296, 1.317912415714726393 ) ) ;
#27349=EDGE_LOOP ( 'NONE', ( #25587, #13056, #21733, #25823 ) ) ;
#27351=AXIS2_PLACEMENT_3D ( 'NONE', #25952, #11228, #13746 ) ;
#27364=CARTESIAN_POINT ( 'NONE',  ( -55.75952994616203995, 3.117691453623994580, -1.800000000000184563 ) ) ;
#27371=CARTESIAN_POINT ( 'NONE',  ( -57.57202994616204705, -4.156921938165296204, -2.308488068846171547E-13 ) ) ;
#27385=CARTESIAN_POINT ( 'NONE',  ( -59.18749999999995737, -3.399999999999991029, -2.288065396424332102E-13 ) ) ;
#27389=CARTESIAN_POINT ( 'NONE',  ( -56.44702994616204705, 4.156921938165313080, -1.854183217685626176E-13 ) ) ;
#27397=DIRECTION ( 'NONE',  ( -3.491481338843133355E-15, -3.491481338843133355E-15, 1.000000000000000000 ) ) ;
#27403=CARTESIAN_POINT ( 'NONE',  ( -59.69999999999998153, -2.268174980119396000, 1.538811659727345349 ) ) ;
#27410=CARTESIAN_POINT ( 'NONE',  ( -59.68558439773848789, 2.070002566049753856, 1.729003918826550024 ) ) ;
#27414=ADVANCED_FACE ( 'NONE', ( #10161 ), #14606, .T. ) ;
#27428=CARTESIAN_POINT ( 'NONE',  ( -55.58155989232413674, 3.400000000000007461, -1.857527951337884861E-13 ) ) ;
#27432=CARTESIAN_POINT ( 'NONE',  ( -54.83155989232412963, 3.925981830489463142, -1.806266843080172912E-13 ) ) ;
#27438=CARTESIAN_POINT ( 'NONE',  ( -57.62499999999996447, -2.944486372867076707, -1.700000000000215117 ) ) ;
#27458=CARTESIAN_POINT ( 'NONE',  ( -55.43749999999997158, -3.925981830489445379, -2.111188856984502568E-13 ) ) ;
#27470=CARTESIAN_POINT ( 'NONE',  ( -58.14405989232411542, -2.944486372867076263, -1.700000000000216893 ) ) ;
#27475=CARTESIAN_POINT ( 'NONE',  ( -59.69999999999997442, 8.366749974758454467E-15, -2.120534355533670266E-13 ) ) ;
#27477=DIRECTION ( 'NONE',  ( 1.000000000000000000, -1.219044193948983948E-29, 3.491481338843133355E-15 ) ) ;
#27478=CARTESIAN_POINT ( 'NONE',  ( -59.44986384413810043, 3.257863816608426166, 1.316887994369795978 ) ) ;
#27487=ORIENTED_EDGE ( 'NONE', *, *, #6956, .F. ) ;
#27499=CARTESIAN_POINT ( 'NONE',  ( -57.83155989232412253, 3.400000000000007905, -1.837192174579415376E-13 ) ) ;
#27507=CARTESIAN_POINT ( 'NONE',  ( -55.82202994616203995, 2.078460969082674747, -3.600000000000189715 ) ) ;
#27515=CARTESIAN_POINT ( 'NONE',  ( -58.50952994616205416, -2.184195341338215755E-14, 3.599999999999791367 ) ) ;
#27519=ADVANCED_FACE ( 'NONE', ( #24871 ), #30253, .T. ) ;
#27524=CARTESIAN_POINT ( 'NONE',  ( -54.49626650188002941, -2.282174794334375534, -2.722251751099368011 ) ) ;
#27531=CARTESIAN_POINT ( 'NONE',  ( -59.69702994616202574, -2.078460969082631227, -3.600000000000218137 ) ) ;
#27561=CARTESIAN_POINT ( 'NONE',  ( -59.59999999999998010, 8.366749974758452890E-15, -2.117042874194827196E-13 ) ) ;
#27570=AXIS2_PLACEMENT_3D ( 'NONE', #15051, #334, #14881 ) ;
#27578=CARTESIAN_POINT ( 'NONE',  ( -54.95655989232411542, 1.962990915244748891, -3.400000000000186429 ) ) ;
#27579=ORIENTED_EDGE ( 'NONE', *, *, #11207, .T. ) ;
#27589=CARTESIAN_POINT ( 'NONE',  ( -57.31249999999997158, 3.925981830489463142, -1.892888403967549806E-13 ) ) ;
#27594=TOROIDAL_SURFACE ( 'NONE', #12421, 2.750000000000000000, 0.1000000000000000056 ) ;
#27605=EDGE_CURVE ( 'NONE', #14413, #11810, #28861, .T. ) ;
#27616=CARTESIAN_POINT ( 'NONE',  ( -58.31249999999995026, -1.962990915244707368, -3.400000000000213518 ) ) ;
#27618=ORIENTED_EDGE ( 'NONE', *, *, #1272, .F. ) ;
#27620=ORIENTED_EDGE ( 'NONE', *, *, #15083, .F. ) ;
#27624=FACE_OUTER_BOUND ( 'NONE', #24136, .T. ) ;
#27629=DIRECTION ( 'NONE',  ( 1.000000000000000000, -1.219044193948983948E-29, 3.491481338843133355E-15 ) ) ;
#27634=CARTESIAN_POINT ( 'NONE',  ( -57.70655989232413674, 1.962990915244722245, 3.399999999999802291 ) ) ;
#27655=ORIENTED_EDGE ( 'NONE', *, *, #20091, .F. ) ;
#27663=EDGE_CURVE ( 'NONE', #8534, #17883, #29669, .T. ) ;
#27667=CARTESIAN_POINT ( 'NONE',  ( -54.49999999999996447, 1.500000000000023759, -3.959797974644871044 ) ) ;
#27682=FACE_OUTER_BOUND ( 'NONE', #3948, .T. ) ;
#27690=CARTESIAN_POINT ( 'NONE',  ( -56.57202994616203995, 2.078460969082686294, -3.600000000000185718 ) ) ;
#27693=VERTEX_POINT ( 'NONE', #6990 ) ;
#27703=ADVANCED_FACE ( 'NONE', ( #11877 ), #10959, .T. ) ;
#27706=CARTESIAN_POINT ( 'NONE',  ( -61.00952994616203284, 3.117691453623994580, -1.800000000000202993 ) ) ;
#27710=AXIS2_PLACEMENT_3D ( 'NONE', #9066, #11752, #1608 ) ;
#27719=CARTESIAN_POINT ( 'NONE',  ( -59.59999999999998010, 8.366749974758452890E-15, -2.117042874194827196E-13 ) ) ;
#27728=CARTESIAN_POINT ( 'NONE',  ( -44.49999999999996447, 1.400000000000023670, -3.959797974644836405 ) ) ;
#27736=DIRECTION ( 'NONE',  ( 0.000000000000000000, -1.000000000000000000, -4.379659758543256221E-15 ) ) ;
#27749=CARTESIAN_POINT ( 'NONE',  ( -59.08155989232413674, -1.962990915244731571, 3.399999999999781419 ) ) ;
#27757=CARTESIAN_POINT ( 'NONE',  ( -55.56249999999998579, -1.962990915244731793, 3.399999999999794742 ) ) ;
#27761=CARTESIAN_POINT ( 'NONE',  ( -44.49999999999997868, -1.399999999999992806, -1.638709930773317737E-13 ) ) ;
#27767=LINE ( 'NONE', #1161, #3344 ) ;
#27781=CARTESIAN_POINT ( 'NONE',  ( -56.99999999999997158, -2.944486372867089141, 1.699999999999786571 ) ) ;
#27782=CARTESIAN_POINT ( 'NONE',  ( -59.52159998169275923, 2.135188160778345612, 1.581460861012937924 ) ) ;
#27791=DIRECTION ( 'NONE',  ( 0.000000000000000000, -1.000000000000000000, -3.491481338843133355E-15 ) ) ;
#27798=CARTESIAN_POINT ( 'NONE',  ( -60.39405989232410121, -2.944486372867076263, -1.700000000000224665 ) ) ;
#27817=CARTESIAN_POINT ( 'NONE',  ( -59.19126343180466421, -2.406052454186071277, 1.245092465133171844 ) ) ;
#27818=VERTEX_POINT ( 'NONE', #4121 ) ;
#27824=DIRECTION ( 'NONE',  ( 0.000000000000000000, 1.000000000000000000, 0.000000000000000000 ) ) ;
#27839=CARTESIAN_POINT ( 'NONE',  ( -54.44702994616203995, -2.078460969082631227, -3.600000000000199485 ) ) ;
#27850=AXIS2_PLACEMENT_3D ( 'NONE', #22084, #676, #27121 ) ;
#27861=CARTESIAN_POINT ( 'NONE',  ( -44.59999999999996589, 1.557046979865791769, -3.273565289175096815 ) ) ;
#27868=CARTESIAN_POINT ( 'NONE',  ( -60.38452994616202574, 2.093608279459374244E-14, -3.600000000000214140 ) ) ;
#27874=CARTESIAN_POINT ( 'NONE',  ( -56.59599364905386665, 3.400000000000011902, -0.9110272542659995088 ) ) ;
#27899=CARTESIAN_POINT ( 'NONE',  ( -54.48926665517993229, -2.780759778332207777, -2.383582780284819513 ) ) ;
#27900=CARTESIAN_POINT ( 'NONE',  ( -59.51905989232410121, 2.023778652682510314E-14, -3.400000000000210854 ) ) ;
#27906=AXIS2_PLACEMENT_3D ( 'NONE', #15984, #17759, #27397 ) ;
#27907=CARTESIAN_POINT ( 'NONE',  ( -56.06249999999995737, -1.962990915244707368, -3.400000000000206413 ) ) ;
#27927=CARTESIAN_POINT ( 'NONE',  ( -58.56249999999997868, -1.962990915244731793, 3.399999999999783640 ) ) ;
#27930=ORIENTED_EDGE ( 'NONE', *, *, #12922, .F. ) ;
#27932=VERTEX_POINT ( 'NONE', #16802 ) ;
#27946=CARTESIAN_POINT ( 'NONE',  ( -59.19545262082412762, -2.415331713986693885, 1.247511094541249976 ) ) ;
#27949=DIRECTION ( 'NONE',  ( 1.000000000000000000, -1.219044193948983948E-29, 3.491481338843133355E-15 ) ) ;
#27960=ORIENTED_EDGE ( 'NONE', *, *, #28279, .F. ) ;
#27972=CARTESIAN_POINT ( 'NONE',  ( -56.20655989232413674, 1.962990915244719359, 3.399999999999808509 ) ) ;
#27982=CARTESIAN_POINT ( 'NONE',  ( -58.43749999999997158, -3.399999999999991029, -2.253785087031484148E-13 ) ) ;
#27983=ADVANCED_FACE ( 'NONE', ( #29751 ), #17733, .F. ) ;
#27995=AXIS2_PLACEMENT_3D ( 'NONE', #6670, #23308, #1745 ) ;
#27998=EDGE_LOOP ( 'NONE', ( #18832, #17969, #28543, #30110 ) ) ;
#28016=DIRECTION ( 'NONE',  ( -1.000000000000000000, 0.000000000000000000, -8.673617379883787770E-15 ) ) ;
#28019=EDGE_CURVE ( 'NONE', #30275, #1323, #19601, .T. ) ;
#28046=CARTESIAN_POINT ( 'NONE',  ( -58.64405989232411542, 2.944486372867106461, -1.700000000000195577 ) ) ;
#28048=DIRECTION ( 'NONE',  ( 3.491481338843133355E-15, 3.491481338843133355E-15, -1.000000000000000000 ) ) ;
#28053=CARTESIAN_POINT ( 'NONE',  ( -57.74999999999997158, -2.944486372867089141, 1.699999999999783906 ) ) ;
#28061=AXIS2_PLACEMENT_3D ( 'NONE', #30145, #15750, #18291 ) ;
#28065=CARTESIAN_POINT ( 'NONE',  ( -59.68658240507107138, -2.223882124562203799, 1.531065007683262591 ) ) ;
#28075=CARTESIAN_POINT ( 'NONE',  ( -57.31249999999997158, 3.925981830489463142, -1.892888403967549806E-13 ) ) ;
#28088=CARTESIAN_POINT ( 'NONE',  ( -44.49999999999997868, 8.366749974758269874E-15, -1.589829192029513996E-13 ) ) ;
#28090=CARTESIAN_POINT ( 'NONE',  ( -54.49150557875106671, -3.119347353020518465, -1.738776940373585767 ) ) ;
#28091=ORIENTED_EDGE ( 'NONE', *, *, #15470, .T. ) ;
#28098=CARTESIAN_POINT ( 'NONE',  ( -59.69999999999997442, -2.473915798711235237, -1.238538609462283446 ) ) ;
#28104=SPHERICAL_SURFACE ( 'NONE', #11887, 0.1000000000000000056 ) ;
#28114=VECTOR ( 'NONE', #18087, 1000.000000000000000 ) ;
#28123=ORIENTED_EDGE ( 'NONE', *, *, #21039, .T. ) ;
#28125=ADVANCED_FACE ( 'NONE', ( #21217 ), #1873, .T. ) ;
#28139=CARTESIAN_POINT ( 'NONE',  ( -58.82202994616202574, 2.078460969082674747, -3.600000000000199929 ) ) ;
#28143=CARTESIAN_POINT ( 'NONE',  ( -59.19999999999997442, -3.382957286162487698, 0.3399999999999019917 ) ) ;
#28165=DIRECTION ( 'NONE',  ( 0.000000000000000000, -1.000000000000000000, -3.491481338843132961E-15 ) ) ;
#28190=CIRCLE ( 'NONE', #7477, 4.199999999999954881 ) ;
#28193=AXIS2_PLACEMENT_3D ( 'NONE', #14379, #14227, #26574 ) ;
#28196=DIRECTION ( 'NONE',  ( -2.095850865446309212E-30, -1.000000000000000000, -2.891205793294679411E-15 ) ) ;
#28199=DIRECTION ( 'NONE',  ( -1.000000000000000000, 1.219044193948983948E-29, -3.491481338843133355E-15 ) ) ;
#28220=CARTESIAN_POINT ( 'NONE',  ( -55.00952994616204705, 3.117691453623994580, -1.800000000000181899 ) ) ;
#28221=CARTESIAN_POINT ( 'NONE',  ( -58.26905989232412253, -2.944486372867088697, 1.699999999999781686 ) ) ;
#28225=CARTESIAN_POINT ( 'NONE',  ( -55.63452994616205416, 3.117691453623979481, 1.799999999999814415 ) ) ;
#28229=CARTESIAN_POINT ( 'NONE',  ( -59.27299602954527558, -2.279082375080590417, 1.356559916049900005 ) ) ;
#28248=CARTESIAN_POINT ( 'NONE',  ( -61.24999999999995026, 2.023778652682512839E-14, -3.400000000000217515 ) ) ;
#28260=CARTESIAN_POINT ( 'NONE',  ( -54.49999999999997868, -3.396648781713578202, -1.005585003271797007 ) ) ;
#28265=CARTESIAN_POINT ( 'NONE',  ( -61.01905989232410121, 2.023778652682512207E-14, -3.400000000000216183 ) ) ;
#28279=EDGE_CURVE ( 'NONE', #10060, #15811, #12831, .T. ) ;
#28283=ORIENTED_EDGE ( 'NONE', *, *, #26349, .T. ) ;
#28289=ORIENTED_EDGE ( 'NONE', *, *, #713, .F. ) ;
#28290=ORIENTED_EDGE ( 'NONE', *, *, #27605, .F. ) ;
#28307=CARTESIAN_POINT ( 'NONE',  ( -56.82202994616205416, -4.156921938165296204, -2.167734102480683039E-13 ) ) ;
#28308=CARTESIAN_POINT ( 'NONE',  ( -59.31366000257239790, 3.244990441519633784, -1.015485107948731702 ) ) ;
#28314=DIRECTION ( 'NONE',  ( -1.000000000000000000, 1.219044193948983948E-29, -3.491481338843133355E-15 ) ) ;
#28317=CARTESIAN_POINT ( 'NONE',  ( -59.50952994616202574, 3.117691453624007014, -1.800000000000176570 ) ) ;
#28334=ORIENTED_EDGE ( 'NONE', *, *, #29897, .F. ) ;
#28339=CARTESIAN_POINT ( 'NONE',  ( -56.93749999999996447, -3.399999999999991473, -2.119568960425587465E-13 ) ) ;
#28351=DIRECTION ( 'NONE',  ( 0.000000000000000000, -1.000000000000000000, 0.000000000000000000 ) ) ;
#28354=LINE ( 'NONE', #18711, #15498 ) ;
#28355=ORIENTED_EDGE ( 'NONE', *, *, #14663, .T. ) ;
#28362=ORIENTED_EDGE ( 'NONE', *, *, #11318, .T. ) ;
#28363=VERTEX_POINT ( 'NONE', #10489 ) ;
#28373=CARTESIAN_POINT ( 'NONE',  ( -56.64405989232412253, -2.944486372867076263, -1.700000000000211786 ) ) ;
#28377=ORIENTED_EDGE ( 'NONE', *, *, #30832, .F. ) ;
#28378=CARTESIAN_POINT ( 'NONE',  ( -61.18749999999995737, 1.962990915244749557, -3.400000000000207745 ) ) ;
#28393=( BOUNDED_CURVE ( )  B_SPLINE_CURVE ( 2, ( #15835, #29779, #25013, #22504, #8096, #8553, #25188, #3343, #18237 ),
 .UNSPECIFIED., .F., .T. ) 
 B_SPLINE_CURVE_WITH_KNOTS ( ( 3, 2, 2, 2, 3 ),
 ( 0.02777777777777778317, 0.03703703703703703498, 0.05555555555555555247, 0.07407407407407406996, 0.08333333333333332871 ),
 .UNSPECIFIED. ) 
 CURVE ( )  GEOMETRIC_REPRESENTATION_ITEM ( )  RATIONAL_B_SPLINE_CURVE ( ( 0.9330127018922194093, 0.9330127018922194093, 1.000000000000000000, 0.8660254037844387076, 1.000000000000000000, 0.8660254037844387076, 1.000000000000000000, 0.9330127018922194093, 0.9330127018922194093 ) ) 
 REPRESENTATION_ITEM ( '' )  );
#28394=CARTESIAN_POINT ( 'NONE',  ( -54.39999999999996305, 1.600000000000021627, -3.363870538531679610 ) ) ;
#28398=DIRECTION ( 'NONE',  ( -1.000000000000000000, 1.219044193948983948E-29, -3.491481338843133355E-15 ) ) ;
#28404=CARTESIAN_POINT ( 'NONE',  ( -59.24999999999997158, -2.944486372867089141, 1.699999999999778799 ) ) ;
#28414=CARTESIAN_POINT ( 'NONE',  ( -59.69142724121850563, -2.412383461849193278, -1.233589124872107146 ) ) ;
#28416=LINE ( 'NONE', #23044, #30854 ) ;
#28437=CARTESIAN_POINT ( 'NONE',  ( -59.16550086808892672, -2.368432354959790320, 1.240591571384440872 ) ) ;
#28451=CARTESIAN_POINT ( 'NONE',  ( -54.39999999999997726, 1.400000000000009681, -1.886605105831180521E-13 ) ) ;
#28460=CARTESIAN_POINT ( 'NONE',  ( -58.00952994616203284, 3.117691453623994580, -1.800000000000192557 ) ) ;
#28461=CARTESIAN_POINT ( 'NONE',  ( -59.11985793442325843, -2.471172619865210862, -0.9613403835037039880 ) ) ;
#28463=DIRECTION ( 'NONE',  ( 0.000000000000000000, -1.000000000000000000, -3.613946018757958434E-15 ) ) ;
#28472=CARTESIAN_POINT ( 'NONE',  ( -44.59999999999996589, 1.600000000000021627, -3.363870538531645416 ) ) ;
#28475=ORIENTED_EDGE ( 'NONE', *, *, #7687, .F. ) ;
#28484=CARTESIAN_POINT ( 'NONE',  ( -44.59999999999999432, -1.500000000000006883, 4.029888335921774534 ) ) ;
#28487=AXIS2_PLACEMENT_3D ( 'NONE', #12051, #16955, #27222 ) ;
#28499=CARTESIAN_POINT ( 'NONE',  ( -54.39999999999999147, -1.600000000000004530, 3.363870538531237742 ) ) ;
#28515=ORIENTED_EDGE ( 'NONE', *, *, #4583, .T. ) ;
#28525=CARTESIAN_POINT ( 'NONE',  ( -60.76905989232411542, 2.944486372867092250, 1.699999999999795675 ) ) ;
#28530=CARTESIAN_POINT ( 'NONE',  ( -60.56249999999995026, -1.962990915244707368, -3.400000000000221956 ) ) ;
#28543=ORIENTED_EDGE ( 'NONE', *, *, #20843, .T. ) ;
#28544=DIRECTION ( 'NONE',  ( 0.000000000000000000, -1.000000000000000000, -3.491481338843129805E-15 ) ) ;
#28548=CARTESIAN_POINT ( 'NONE',  ( -54.49999999999999289, 1.557046979865768899, 3.273565289174698467 ) ) ;
#28556=CARTESIAN_POINT ( 'NONE',  ( -55.50952994616206126, -4.643455692769921685E-15, 3.599999999999801581 ) ) ;
#28563=CARTESIAN_POINT ( 'NONE',  ( -57.57202994616204705, -4.156921938165296204, -2.193920212522006445E-13 ) ) ;
#28578=CARTESIAN_POINT ( 'NONE',  ( -44.59999999999996589, 1.514093959731561467, -3.183260039818548659 ) ) ;
#28582=CARTESIAN_POINT ( 'NONE',  ( -58.92306624327022746, -3.399999999999988365, -0.9110272542660498019 ) ) ;
#28588=ORIENTED_EDGE ( 'NONE', *, *, #10469, .F. ) ;
#28591=TOROIDAL_SURFACE ( 'NONE', #23039, 3.524999999999996358, 0.1000000000000000056 ) ;
#28592=ORIENTED_EDGE ( 'NONE', *, *, #26901, .F. ) ;
#28595=EDGE_CURVE ( 'NONE', #6234, #17704, #21732, .T. ) ;
#28603=CIRCLE ( 'NONE', #29599, 0.1000000000000000472 ) ;
#28606=DIRECTION ( 'NONE',  ( -3.491481338843133355E-15, 5.182136041040898961E-15, 1.000000000000000000 ) ) ;
#28617=CARTESIAN_POINT ( 'NONE',  ( -57.75952994616205416, -4.643455692769894075E-15, 3.599999999999794031 ) ) ;
#28623=AXIS2_PLACEMENT_3D ( 'NONE', #21428, #26324, #31060 ) ;
#28664=CARTESIAN_POINT ( 'NONE',  ( -54.49999999999996447, 1.600000000000021627, -3.363870538531680054 ) ) ;
#28665=CARTESIAN_POINT ( 'NONE',  ( -59.09999999999997300, 2.465712773623992327, -0.9709585562669131864 ) ) ;
#28680=AXIS2_PLACEMENT_3D ( 'NONE', #28578, #19259, #26208 ) ;
#28692=EDGE_LOOP ( 'NONE', ( #25974, #11502, #21734, #3248 ) ) ;
#28703=CARTESIAN_POINT ( 'NONE',  ( -60.49999999999995737, 2.023778652682511576E-14, -3.400000000000214850 ) ) ;
#28711=VECTOR ( 'NONE', #11337, 1000.000000000000000 ) ;
#28730=CARTESIAN_POINT ( 'NONE',  ( -55.00952994616204705, 3.117691453623994580, -1.800000000000181899 ) ) ;
#28731=VERTEX_POINT ( 'NONE', #19295 ) ;
#28733=CARTESIAN_POINT ( 'NONE',  ( -59.51599740598381771, 3.364165731847367447, -1.132304662275449569 ) ) ;
#28736=CARTESIAN_POINT ( 'NONE',  ( -58.19702994616203284, -2.078460969082631227, -3.600000000000212363 ) ) ;
#28747=FACE_OUTER_BOUND ( 'NONE', #28692, .T. ) ;
#28754=EDGE_CURVE ( 'NONE', #27818, #19242, #17597, .T. ) ;
#28766=ORIENTED_EDGE ( 'NONE', *, *, #22832, .T. ) ;
#28777=DIRECTION ( 'NONE',  ( 1.000000000000000000, -1.219044193948983948E-29, 3.491481338843133355E-15 ) ) ;
#28778=CARTESIAN_POINT ( 'NONE',  ( -60.63452994616204705, -3.117691453623976816, 1.799999999999772671 ) ) ;
#28780=CARTESIAN_POINT ( 'NONE',  ( -59.13880064263039316, -2.480191926443811479, -0.9536590270807077108 ) ) ;
#28783=DIRECTION ( 'NONE',  ( -3.491481338843133355E-15, -3.613946018757868503E-15, 1.000000000000000000 ) ) ;
#28814=CARTESIAN_POINT ( 'NONE',  ( -58.06249999999996447, 3.400000000000007905, -1.844164440896605116E-13 ) ) ;
#28826=CARTESIAN_POINT ( 'NONE',  ( -59.09665968485343512, 2.466443774698494629, -0.9691001528487590555 ) ) ;
#28841=ORIENTED_EDGE ( 'NONE', *, *, #25272, .F. ) ;
#28847=CARTESIAN_POINT ( 'NONE',  ( -60.58155989232412253, -1.962990915244731571, 3.399999999999776534 ) ) ;
#28855=CARTESIAN_POINT ( 'NONE',  ( -54.69702994616206837, -2.078460969082657872, 3.599999999999797584 ) ) ;
#28859=CARTESIAN_POINT ( 'NONE',  ( -44.59999999999998721, -1.400000000000004574, 3.363870538531272825 ) ) ;
#28861=( BOUNDED_CURVE ( )  B_SPLINE_CURVE ( 2, ( #17917, #981, #20773, #12828, #6048, #22510, #20311, #15700, #25347 ),
 .UNSPECIFIED., .F., .T. ) 
 B_SPLINE_CURVE_WITH_KNOTS ( ( 3, 2, 2, 2, 3 ),
 ( 0.7011399156489748208, 0.7037037037037037202, 0.7222222222222222099, 0.7407407407407406996, 0.7424297805561814734 ),
 .UNSPECIFIED. ) 
 CURVE ( )  GEOMETRIC_REPRESENTATION_ITEM ( )  RATIONAL_B_SPLINE_CURVE ( ( 0.9680396472854365664, 0.9814519466516125057, 1.000000000000000000, 0.8660254037844387076, 1.000000000000000000, 0.8660254037844387076, 1.000000000000000000, 0.9877804249276531667, 0.9777898995284022288 ) ) 
 REPRESENTATION_ITEM ( '' )  );
#28879=CARTESIAN_POINT ( 'NONE',  ( -61.06249999999995737, 3.925981830489463142, -2.023818954174166834E-13 ) ) ;
#28882=CARTESIAN_POINT ( 'NONE',  ( -59.49584459105846435, 3.403422474738959203, -1.120669429153365870 ) ) ;
#28883=ORIENTED_EDGE ( 'NONE', *, *, #677, .F. ) ;
#28885=CARTESIAN_POINT ( 'NONE',  ( -57.88452994616205416, 3.117691453623979481, 1.799999999999806422 ) ) ;
#28908=EDGE_LOOP ( 'NONE', ( #14502, #12576, #29795, #18056 ) ) ;
#28925=CARTESIAN_POINT ( 'NONE',  ( -60.94702994616203995, 4.156921938165313080, -2.011299877933566609E-13 ) ) ;
#28928=AXIS2_PLACEMENT_3D ( 'NONE', #532, #17474, #19560 ) ;
#28930=CARTESIAN_POINT ( 'NONE',  ( -54.49999999999997868, -4.766731106216463600E-14, -1.834893917355220926E-13 ) ) ;
#28936=CARTESIAN_POINT ( 'NONE',  ( -54.49999999999996447, 1.514093959731561467, -3.183260039818583298 ) ) ;
#28957=CARTESIAN_POINT ( 'NONE',  ( -59.41132486540516311, 2.423250918913632201, 1.250136525132548027 ) ) ;
#28974=LINE ( 'NONE', #24381, #1848 ) ;
#28977=CYLINDRICAL_SURFACE ( 'NONE', #8518, 3.399999999999999911 ) ;
#28979=CARTESIAN_POINT ( 'NONE',  ( -44.59999999999995879, 1.500000000000023981, -4.029888335922147569 ) ) ;
#28992=ORIENTED_EDGE ( 'NONE', *, *, #6721, .T. ) ;
#28998=ORIENTED_EDGE ( 'NONE', *, *, #22253, .F. ) ;
#29002=CARTESIAN_POINT ( 'NONE',  ( -56.44702994616204705, 4.156921938165313080, -1.854183217685626176E-13 ) ) ;
#29011=CARTESIAN_POINT ( 'NONE',  ( -54.49999999999997868, 8.366749974758489177E-15, -2.216533082070116467E-13 ) ) ;
#29020=CARTESIAN_POINT ( 'NONE',  ( -58.24999999999995737, 3.648081215184779629E-14, -3.400000000000207301 ) ) ;
#29029=CARTESIAN_POINT ( 'NONE',  ( -59.38452994616203995, 3.117691453623979481, 1.799999999999801092 ) ) ;
#29032=CARTESIAN_POINT ( 'NONE',  ( -59.50593083503063951, 3.383800819141645100, -1.126492724825817415 ) ) ;
#29033=ORIENTED_EDGE ( 'NONE', *, *, #21764, .T. ) ;
#29035=CARTESIAN_POINT ( 'NONE',  ( -55.69702994616204705, 4.156921938165313080, -1.827997107644302771E-13 ) ) ;
#29036=ORIENTED_EDGE ( 'NONE', *, *, #713, .T. ) ;
#29045=CARTESIAN_POINT ( 'NONE',  ( -59.61589511801003738, 3.087468777912107942, -1.452347209873861456 ) ) ;
#29047=CIRCLE ( 'NONE', #15383, 0.1000000000000000472 ) ;
#29066=ORIENTED_EDGE ( 'NONE', *, *, #29487, .F. ) ;
#29078=EDGE_CURVE ( 'NONE', #11667, #826, #1956, .T. ) ;
#29081=CARTESIAN_POINT ( 'NONE',  ( -54.64405989232413674, -3.920666489018357767E-15, 3.399999999999804512 ) ) ;
#29083=CARTESIAN_POINT ( 'NONE',  ( -58.77900635094606940, 3.400000000000002132, 0.9110272542656305816 ) ) ;
#29091=CARTESIAN_POINT ( 'NONE',  ( -59.69818608288214534, -2.432011272524986278, -1.237491343926018006 ) ) ;
#29093=AXIS2_PLACEMENT_3D ( 'NONE', #18162, #12901, #1187 ) ;
#29098=CIRCLE ( 'NONE', #27570, 0.09999999999999963085 ) ;
#29101=CARTESIAN_POINT ( 'NONE',  ( -57.31249999999996447, 3.400000000000008349, -1.881930883448047941E-13 ) ) ;
#29106=CARTESIAN_POINT ( 'NONE',  ( -58.58155989232410832, 3.400000000000007905, -1.908076882137507950E-13 ) ) ;
#29113=CARTESIAN_POINT ( 'NONE',  ( -55.24999999999996447, 2.107054635024525356E-14, -3.400000000000196643 ) ) ;
#29116=CARTESIAN_POINT ( 'NONE',  ( -57.81249999999998579, -1.962990915244744228, 3.399999999999779643 ) ) ;
#29151=ORIENTED_EDGE ( 'NONE', *, *, #19481, .F. ) ;
#29160=CARTESIAN_POINT ( 'NONE',  ( -56.38452994616205416, 3.117691453623979481, 1.799999999999811751 ) ) ;
#29168=CIRCLE ( 'NONE', #1857, 0.09999999999999999167 ) ;
#29180=VECTOR ( 'NONE', #19809, 1000.000000000000000 ) ;
#29185=ORIENTED_EDGE ( 'NONE', *, *, #23484, .T. ) ;
#29196=CARTESIAN_POINT ( 'NONE',  ( -55.25952994616203995, -3.117691453623963938, -1.800000000000207434 ) ) ;
#29199=AXIS2_PLACEMENT_3D ( 'NONE', #30881, #13755, #17691 ) ;
#29204=FACE_OUTER_BOUND ( 'NONE', #3135, .T. ) ;
#29230=VECTOR ( 'NONE', #16227, 1000.000000000000000 ) ;
#29239=CARTESIAN_POINT ( 'NONE',  ( -59.09999999999997300, 8.366749974758448157E-15, -2.099585467500611340E-13 ) ) ;
#29241=CARTESIAN_POINT ( 'NONE',  ( -56.08155989232413674, -1.962990915244731571, 3.399999999999792077 ) ) ;
#29257=DIRECTION ( 'NONE',  ( 0.000000000000000000, -1.000000000000000000, -3.491481338843132961E-15 ) ) ;
#29265=PLANE ( 'NONE',  #25989 ) ;
#29274=CARTESIAN_POINT ( 'NONE',  ( -55.09599364905385954, 3.400000000000011902, -0.9110272542659996198 ) ) ;
#29284=CARTESIAN_POINT ( 'NONE',  ( -54.49999999999997158, -3.430639028629426601, -0.8101486624347474796 ) ) ;
#29285=CARTESIAN_POINT ( 'NONE',  ( -59.48573950359912743, 3.423031164920794289, -1.114835254188495162 ) ) ;
#29296=DIRECTION ( 'NONE',  ( 2.010641683997904432E-15, 0.9428090415820644665, -0.3333333333333307613 ) ) ;
#29304=CARTESIAN_POINT ( 'NONE',  ( -59.60196120585266044, -2.158270994723152647, 1.537682753760200027 ) ) ;
#29313=CARTESIAN_POINT ( 'NONE',  ( -57.00952994616205416, -4.643455692769903542E-15, 3.599999999999796696 ) ) ;
#29319=CARTESIAN_POINT ( 'NONE',  ( -57.01905989232412963, 2.944486372867089141, 1.699999999999813216 ) ) ;
#29326=EDGE_CURVE ( 'NONE', #24402, #6307, #3687, .T. ) ;
#29331=CARTESIAN_POINT ( 'NONE',  ( -58.18749999999995737, 1.962990915244761991, -3.400000000000190870 ) ) ;
#29333=CARTESIAN_POINT ( 'NONE',  ( -54.39999999999996305, 1.400000000000023670, -3.959797974644871044 ) ) ;
#29339=CARTESIAN_POINT ( 'NONE',  ( -44.59999999999996589, -1.499999999999981126, -3.363870538531657406 ) ) ;
#29343=CARTESIAN_POINT ( 'NONE',  ( -60.38452994616202574, 2.093608279459374244E-14, -3.600000000000214140 ) ) ;
#29355=ADVANCED_FACE ( 'NONE', ( #18093 ), #11098, .T. ) ;
#29361=DIRECTION ( 'NONE',  ( 0.000000000000000000, -1.000000000000000000, -4.336808689942015369E-15 ) ) ;
#29365=( BOUNDED_CURVE ( )  B_SPLINE_CURVE ( 3, ( #16752, #19289, #11827, #12147 ),
 .UNSPECIFIED., .F., .T. ) 
 B_SPLINE_CURVE_WITH_KNOTS ( ( 4, 4 ),
 ( 2.002124161478338937, 2.111507728364524272 ),
 .UNSPECIFIED. ) 
 CURVE ( )  GEOMETRIC_REPRESENTATION_ITEM ( )  RATIONAL_B_SPLINE_CURVE ( ( 1.000000000000000000, 0.9990031847838436452, 0.9990031847838436452, 1.000000000000000000 ) ) 
 REPRESENTATION_ITEM ( '' )  );
#29375=B_SPLINE_CURVE_WITH_KNOTS ( 'NONE', 3,
 ( #26765, #26545, #26242, #16754, #16276, #11994, #14351, #9155, #28780, #11682, #28461, #18971, #14200, #19140, #6764, #9635 ),
 .UNSPECIFIED., .F., .F.,
 ( 4, 3, 3, 3, 3, 4 ),
 ( 0.000000000000000000, 3.327919720224046293E-05, 6.635940013767358458E-05, 0.0001026099359405011871, 0.0001331273372812267933, 0.0001352886551855475084 ),
 .UNSPECIFIED. ) ;
#29381=DIRECTION ( 'NONE',  ( 0.000000000000000000, -1.000000000000000000, -4.336808689942015369E-15 ) ) ;
#29384=CARTESIAN_POINT ( 'NONE',  ( -54.70655989232413674, 1.962990915244722245, 3.399999999999812950 ) ) ;
#29410=CARTESIAN_POINT ( 'NONE',  ( -57.95655989232411542, 1.962990915244761103, -3.400000000000189981 ) ) ;
#29411=CARTESIAN_POINT ( 'NONE',  ( -59.69865663803934552, 2.434220863071083318, -1.237763019072676940 ) ) ;
#29412=EDGE_CURVE ( 'NONE', #11849, #6214, #21261, .T. ) ;
#29439=EDGE_CURVE ( 'NONE', #1323, #4682, #24240, .T. ) ;
#29442=LINE ( 'NONE', #14733, #29180 ) ;
#29450=CARTESIAN_POINT ( 'NONE',  ( -58.07202994616203995, 2.078460969082674747, -3.600000000000197709 ) ) ;
#29451=CARTESIAN_POINT ( 'NONE',  ( -55.20655989232412963, -3.399999999999991473, -2.086450695418937968E-13 ) ) ;
#29455=CARTESIAN_POINT ( 'NONE',  ( -56.95655989232413674, 1.962990915244718915, 3.399999999999805844 ) ) ;
#29460=DIRECTION ( 'NONE',  ( -1.000000000000000000, 1.219044193948983948E-29, -3.491481338843133355E-15 ) ) ;
#29463=ORIENTED_EDGE ( 'NONE', *, *, #24764, .T. ) ;
#29477=ORIENTED_EDGE ( 'NONE', *, *, #26993, .F. ) ;
#29479=CARTESIAN_POINT ( 'NONE',  ( -60.75952994616205416, -4.643455692769856999E-15, 3.599999999999783373 ) ) ;
#29484=AXIS2_PLACEMENT_3D ( 'NONE', #197, #10029, #14609 ) ;
#29487=EDGE_CURVE ( 'NONE', #16075, #4682, #8911, .T. ) ;
#29492=CARTESIAN_POINT ( 'NONE',  ( -59.19999999999997442, 3.161828374300071687, 1.250136525132551357 ) ) ;
#29511=EDGE_CURVE ( 'NONE', #24802, #16489, #2914, .T. ) ;
#29515=ORIENTED_EDGE ( 'NONE', *, *, #14323, .F. ) ;
#29525=CARTESIAN_POINT ( 'NONE',  ( -57.14405989232411542, 2.944486372867106461, -1.700000000000190248 ) ) ;
#29537=ORIENTED_EDGE ( 'NONE', *, *, #26854, .T. ) ;
#29557=DIRECTION ( 'NONE',  ( -1.344447539785323523E-44, 1.000000000000000000, 3.491481338843137300E-15 ) ) ;
#29577=ADVANCED_FACE ( 'NONE', ( #3629 ), #16135, .T. ) ;
#29578=CARTESIAN_POINT ( 'NONE',  ( -58.88452994616202574, 2.622655696691028948E-14, -3.600000000000208811 ) ) ;
#29579=DIRECTION ( 'NONE',  ( -1.000000000000000000, 1.219044193948983948E-29, -3.491481338843133355E-15 ) ) ;
#29587=ORIENTED_EDGE ( 'NONE', *, *, #4979, .T. ) ;
#29594=CARTESIAN_POINT ( 'NONE',  ( -58.82202994616202574, 2.078460969082674747, -3.600000000000199929 ) ) ;
#29599=AXIS2_PLACEMENT_3D ( 'NONE', #19093, #26506, #23689 ) ;
#29604=CARTESIAN_POINT ( 'NONE',  ( -56.69702994616203284, -2.078460969082631227, -3.600000000000207923 ) ) ;
#29606=CARTESIAN_POINT ( 'NONE',  ( -54.49999999999999289, -1.557046979865776448, 3.273565289174688253 ) ) ;
#29613=CYLINDRICAL_SURFACE ( 'NONE', #21623, 3.399999999999999911 ) ;
#29638=ORIENTED_EDGE ( 'NONE', *, *, #16418, .T. ) ;
#29644=CARTESIAN_POINT ( 'NONE',  ( -54.26905989232411542, 2.023778652682504003E-14, -3.400000000000192646 ) ) ;
#29645=EDGE_LOOP ( 'NONE', ( #12694, #14958, #28588, #26775 ) ) ;
#29653=AXIS2_PLACEMENT_3D ( 'NONE', #3337, #12987, #22674 ) ;
#29654=CARTESIAN_POINT ( 'NONE',  ( -59.21142689504641510, -3.199784673776251864, 1.256733846063594839 ) ) ;
#29663=CIRCLE ( 'NONE', #16014, 0.1000000000000028644 ) ;
#29665=AXIS2_PLACEMENT_3D ( 'NONE', #4835, #16256, #31121 ) ;
#29669=CIRCLE ( 'NONE', #21614, 0.1000000000000028644 ) ;
#29676=EDGE_CURVE ( 'NONE', #13776, #7345, #15071, .T. ) ;
#29677=ORIENTED_EDGE ( 'NONE', *, *, #6459, .T. ) ;
#29696=CARTESIAN_POINT ( 'NONE',  ( -60.51905989232411542, -2.944486372867088697, 1.699999999999773914 ) ) ;
#29702=VECTOR ( 'NONE', #16729, 1000.000000000000000 ) ;
#29716=ORIENTED_EDGE ( 'NONE', *, *, #20965, .F. ) ;
#29725=ORIENTED_EDGE ( 'NONE', *, *, #22253, .T. ) ;
#29726=CARTESIAN_POINT ( 'NONE',  ( -57.79806624327024878, 3.400000000000002576, 0.9110272542656324690 ) ) ;
#29733=CARTESIAN_POINT ( 'NONE',  ( -56.18749999999997868, -3.399999999999991029, -2.152687225432237971E-13 ) ) ;
#29738=CARTESIAN_POINT ( 'NONE',  ( -55.44702994616206126, -2.078460969082657872, 3.599999999999794920 ) ) ;
#29741=CIRCLE ( 'NONE', #22169, 0.1000000000000000472 ) ;
#29748=DIRECTION ( 'NONE',  ( 1.000000000000000000, -1.219044193948983948E-29, 3.491481338843133355E-15 ) ) ;
#29751=FACE_OUTER_BOUND ( 'NONE', #7619, .T. ) ;
#29758=VERTEX_POINT ( 'NONE', #22302 ) ;
#29765=CARTESIAN_POINT ( 'NONE',  ( -57.57202994616204705, -4.156921938165296204, -2.193920212522006445E-13 ) ) ;
#29779=CARTESIAN_POINT ( 'NONE',  ( -54.72099364905386665, -3.399999999999994138, 0.9110272542656107087 ) ) ;
#29795=ORIENTED_EDGE ( 'NONE', *, *, #18069, .F. ) ;
#29811=CARTESIAN_POINT ( 'NONE',  ( -60.63452994616204705, -3.117691453623976816, 1.799999999999772671 ) ) ;
#29813=CARTESIAN_POINT ( 'NONE',  ( -59.69464122902330416, 2.086944863889884871, 1.740854861534822273 ) ) ;
#29818=CARTESIAN_POINT ( 'NONE',  ( -54.74999999999997868, -2.944486372867089141, 1.699999999999794342 ) ) ;
#29826=CARTESIAN_POINT ( 'NONE',  ( -59.19999999999997442, 8.366749974758448157E-15, -2.103076948839454410E-13 ) ) ;
#29837=CARTESIAN_POINT ( 'NONE',  ( -59.10047575464341207, 2.308863783365080913, 1.300633787035090361 ) ) ;
#29839=CARTESIAN_POINT ( 'NONE',  ( -57.12499999999997868, -3.920666489018328579E-15, 3.399999999999796518 ) ) ;
#29840=CARTESIAN_POINT ( 'NONE',  ( -59.51187924496046833, 2.330100891901230487, 1.424301819445882744 ) ) ;
#29849=CARTESIAN_POINT ( 'NONE',  ( -57.26905989232410832, 2.356882582050587835E-14, -3.400000000000203304 ) ) ;
#29853=CARTESIAN_POINT ( 'NONE',  ( -57.26905989232410832, 2.023778652682507790E-14, -3.400000000000203304 ) ) ;
#29859=LINE ( 'NONE', #24643, #30147 ) ;
#29872=CARTESIAN_POINT ( 'NONE',  ( -59.19495429951913223, -2.548385458854336871, -0.9469503383366065785 ) ) ;
#29894=CARTESIAN_POINT ( 'NONE',  ( -54.82202994616206126, 2.078460969082646770, 3.599999999999812683 ) ) ;
#29897=EDGE_CURVE ( 'NONE', #27932, #24984, #11184, .T. ) ;
#29902=CARTESIAN_POINT ( 'NONE',  ( -57.38452994616203284, 2.446306557613808189E-14, -3.600000000000203926 ) ) ;
#29908=CARTESIAN_POINT ( 'NONE',  ( -59.10063086800197851, 2.465840246069578523, -0.9706348447806306678 ) ) ;
#29909=CARTESIAN_POINT ( 'NONE',  ( -54.49542095125566732, -2.304164661794668945, -2.707651631953783333 ) ) ;
#29913=CARTESIAN_POINT ( 'NONE',  ( -59.28559899066483041, 3.161828374300069466, 1.250136525132556020 ) ) ;
#29915=ADVANCED_FACE ( 'NONE', ( #30020 ), #25123, .F. ) ;
#29918=CARTESIAN_POINT ( 'NONE',  ( -58.00952994616203284, 3.117691453623994580, -1.800000000000192557 ) ) ;
#29939=DIRECTION ( 'NONE',  ( 0.000000000000000000, -0.3333333333333488580, -0.9428090415820578052 ) ) ;
#29941=CARTESIAN_POINT ( 'NONE',  ( -54.49999999999999289, -1.600000000000004530, 3.363870538531237298 ) ) ;
#29948=CARTESIAN_POINT ( 'NONE',  ( -59.63821477905805324, -2.352792697908255182, -1.234285180173736451 ) ) ;
#29962=CARTESIAN_POINT ( 'NONE',  ( -54.76905989232412963, 2.944486372867092250, 1.699999999999816769 ) ) ;
#29963=ORIENTED_EDGE ( 'NONE', *, *, #6941, .T. ) ;
#29968=CARTESIAN_POINT ( 'NONE',  ( -55.74999999999997868, 2.944486372867092250, 1.699999999999813438 ) ) ;
#29972=DIRECTION ( 'NONE',  ( 0.000000000000000000, -4.336808689942006692E-15, 1.000000000000000000 ) ) ;
#29985=CARTESIAN_POINT ( 'NONE',  ( -59.14374655978132722, 2.337443148762131440, 1.267909066924384875 ) ) ;
#29988=CARTESIAN_POINT ( 'NONE',  ( -55.49999999999997868, -2.944486372867089141, 1.699999999999791678 ) ) ;
#29999=CARTESIAN_POINT ( 'NONE',  ( -44.49999999999997868, 1.400000000000009681, -1.540948453285710255E-13 ) ) ;
#30000=CARTESIAN_POINT ( 'NONE',  ( -58.76905989232410832, 2.023778652682509368E-14, -3.400000000000208189 ) ) ;
#30005=CARTESIAN_POINT ( 'NONE',  ( -59.69999999999997442, 8.366749974758454467E-15, -2.120534355533670266E-13 ) ) ;
#30007=DIRECTION ( 'NONE',  ( 0.000000000000000000, -1.000000000000000000, -3.491481338843134933E-15 ) ) ;
#30008=EDGE_CURVE ( 'NONE', #11459, #26071, #19099, .T. ) ;
#30012=ORIENTED_EDGE ( 'NONE', *, *, #817, .F. ) ;
#30020=FACE_OUTER_BOUND ( 'NONE', #72, .T. ) ;
#30021=CARTESIAN_POINT ( 'NONE',  ( -44.49999999999996447, -1.399999999999979039, -3.959797974644846619 ) ) ;
#30024=EDGE_CURVE ( 'NONE', #19660, #8146, #14513, .T. ) ;
#30029=DIRECTION ( 'NONE',  ( -1.000000000000000000, 1.219044193948984088E-29, -3.491481338843133750E-15 ) ) ;
#30033=DIRECTION ( 'NONE',  ( 1.000000000000000000, -1.219044193948983948E-29, 3.491481338843133355E-15 ) ) ;
#30036=CARTESIAN_POINT ( 'NONE',  ( -55.50952994616206126, -4.643455692769921685E-15, 3.599999999999801581 ) ) ;
#30038=VERTEX_POINT ( 'NONE', #11664 ) ;
#30047=CARTESIAN_POINT ( 'NONE',  ( -56.50952994616203995, 3.117691453623998132, -1.800000000000180123 ) ) ;
#30063=CARTESIAN_POINT ( 'NONE',  ( -58.07202994616203995, 2.078460969082674747, -3.600000000000197709 ) ) ;
#30066=AXIS2_PLACEMENT_3D ( 'NONE', #19117, #13051, #26983 ) ;
#30086=CARTESIAN_POINT ( 'NONE',  ( -59.65431995858129710, 2.042084323596708995, 1.713960027490288862 ) ) ;
#30092=VERTEX_POINT ( 'NONE', #23708 ) ;
#30095=AXIS2_PLACEMENT_3D ( 'NONE', #13993, #8935, #1644 ) ;
#30097=ORIENTED_EDGE ( 'NONE', *, *, #12096, .F. ) ;
#30098=AXIS2_PLACEMENT_3D ( 'NONE', #9374, #6832, #16499 ) ;
#30105=CARTESIAN_POINT ( 'NONE',  ( -58.58155989232412253, 3.925981830489463142, -1.937197393286790192E-13 ) ) ;
#30109=AXIS2_PLACEMENT_3D ( 'NONE', #20114, #29748, #5680 ) ;
#30110=ORIENTED_EDGE ( 'NONE', *, *, #5952, .F. ) ;
#30112=CARTESIAN_POINT ( 'NONE',  ( -56.18749999999997158, -3.925981830489445379, -2.137374967025826226E-13 ) ) ;
#30117=CARTESIAN_POINT ( 'NONE',  ( -54.49999999999997158, -1.370882916971243537, -3.219442999905937075 ) ) ;
#30125=DIRECTION ( 'NONE',  ( 0.000000000000000000, -1.000000000000000000, -3.491481338843136116E-15 ) ) ;
#30126=CARTESIAN_POINT ( 'NONE',  ( -59.68054851456403753, 2.392282282077082378, -1.229557205448917445 ) ) ;
#30132=CARTESIAN_POINT ( 'NONE',  ( -54.49999999999997158, -3.476573872757579231, -0.4722677507125554452 ) ) ;
#30140=CARTESIAN_POINT ( 'NONE',  ( -57.18749999999998579, 1.962990915244722689, 3.399999999999804956 ) ) ;
#30145=CARTESIAN_POINT ( 'NONE',  ( -44.59999999999998721, 1.514093959731539263, 3.183260039818184062 ) ) ;
#30147=VECTOR ( 'NONE', #27477, 1000.000000000000000 ) ;
#30161=CARTESIAN_POINT ( 'NONE',  ( -59.01905989232412253, -2.944486372867088697, 1.699999999999779243 ) ) ;
#30163=CIRCLE ( 'NONE', #336, 4.299999999999954525 ) ;
#30173=DIRECTION ( 'NONE',  ( 1.000000000000000000, -1.219044193948983948E-29, 3.491481338843133355E-15 ) ) ;
#30186=FACE_OUTER_BOUND ( 'NONE', #18922, .T. ) ;
#30206=VECTOR ( 'NONE', #18271, 1000.000000000000000 ) ;
#30217=CARTESIAN_POINT ( 'NONE',  ( -58.25952994616203284, -3.117691453623959497, -1.800000000000225198 ) ) ;
#30224=CARTESIAN_POINT ( 'NONE',  ( -59.16814806244811109, 2.503608436921294533, -0.9454277352718696292 ) ) ;
#30232=LINE ( 'NONE', #11073, #26149 ) ;
#30241=ORIENTED_EDGE ( 'NONE', *, *, #864, .T. ) ;
#30252=CARTESIAN_POINT ( 'NONE',  ( -44.59999999999998721, 1.399999999999996136, 3.959797974644455376 ) ) ;
#30253=CYLINDRICAL_SURFACE ( 'NONE', #6424, 0.1000000000000000472 ) ;
#30272=ADVANCED_FACE ( 'NONE', ( #553 ), #18322, .T. ) ;
#30273=CARTESIAN_POINT ( 'NONE',  ( -58.39405989232412963, -3.920666489018312013E-15, 3.399999999999791633 ) ) ;
#30275=VERTEX_POINT ( 'NONE', #27861 ) ;
#30278=CARTESIAN_POINT ( 'NONE',  ( -56.12499999999996447, -2.944486372867076707, -1.700000000000210010 ) ) ;
#30282=CARTESIAN_POINT ( 'NONE',  ( -59.09999999999998010, -2.331118226142294247, 1.260312586522342349 ) ) ;
#30285=SPHERICAL_SURFACE ( 'NONE', #11352, 0.1000000000000000056 ) ;
#30286=AXIS2_PLACEMENT_3D ( 'NONE', #17839, #6116, #5793 ) ;
#30293=ORIENTED_EDGE ( 'NONE', *, *, #14437, .F. ) ;
#30295=EDGE_CURVE ( 'NONE', #1451, #30275, #4929, .T. ) ;
#30296=DIRECTION ( 'NONE',  ( -1.344447539785323523E-44, 1.000000000000000000, 3.491481338843137300E-15 ) ) ;
#30299=ORIENTED_EDGE ( 'NONE', *, *, #18744, .F. ) ;
#30301=CARTESIAN_POINT ( 'NONE',  ( -56.62499999999996447, 2.944486372867106905, -1.700000000000188471 ) ) ;
#30303=ORIENTED_EDGE ( 'NONE', *, *, #2930, .T. ) ;
#30326=DIRECTION ( 'NONE',  ( 0.000000000000000000, 1.000000000000000000, 3.491481338843130594E-15 ) ) ;
#30334=EDGE_LOOP ( 'NONE', ( #29638, #8671, #19937, #26016, #8365, #15752 ) ) ;
#30335=CARTESIAN_POINT ( 'NONE',  ( -59.18029295939872014, -2.385974606001367349, 1.241011964822052782 ) ) ;
#30337=ORIENTED_EDGE ( 'NONE', *, *, #8697, .F. ) ;
#30345=DIRECTION ( 'NONE',  ( 3.491481338843133355E-15, 3.491481338843133355E-15, -1.000000000000000000 ) ) ;
#30357=DIRECTION ( 'NONE',  ( -2.095850865446309212E-30, -1.000000000000000000, -2.891205793294679411E-15 ) ) ;
#30366=CIRCLE ( 'NONE', #27850, 0.1000000000000028644 ) ;
#30374=CARTESIAN_POINT ( 'NONE',  ( -59.69999999999997442, 8.366749974758454467E-15, -2.120534355533670266E-13 ) ) ;
#30379=DIRECTION ( 'NONE',  ( 0.000000000000000000, -0.3333333333333235449, 0.9428090415820667980 ) ) ;
#30387=CARTESIAN_POINT ( 'NONE',  ( -59.36246495612066809, 2.315842144512513023, 1.288740169525656176 ) ) ;
#30389=CARTESIAN_POINT ( 'NONE',  ( -60.63452994616204705, -3.117691453623976816, 1.799999999999772671 ) ) ;
#30393=CARTESIAN_POINT ( 'NONE',  ( -59.68658240507107138, -2.223882124562203799, 1.531065007683262591 ) ) ;
#30396=CARTESIAN_POINT ( 'NONE',  ( -54.39999999999996305, -1.557046979865753356, -3.273565289175142556 ) ) ;
#30406=CARTESIAN_POINT ( 'NONE',  ( -59.68054851456403753, -2.392282282077057065, -1.229557205448934099 ) ) ;
#30419=VECTOR ( 'NONE', #8439, 1000.000000000000000 ) ;
#30420=CARTESIAN_POINT ( 'NONE',  ( -55.76905989232411542, 2.023778652682505897E-14, -3.400000000000197975 ) ) ;
#30427=CARTESIAN_POINT ( 'NONE',  ( -56.68749999999996447, 1.962990915244749557, -3.400000000000192646 ) ) ;
#30431=CARTESIAN_POINT ( 'NONE',  ( -59.43987571604603914, -2.221192970515155629, 1.449404383176176037 ) ) ;
#30434=CARTESIAN_POINT ( 'NONE',  ( -54.49999999999997868, 8.366749974758489177E-15, -2.216533082070116467E-13 ) ) ;
#30436=CARTESIAN_POINT ( 'NONE',  ( -59.69997404044342915, 2.118290196927814062, 1.750091561861647493 ) ) ;
#30441=VERTEX_POINT ( 'NONE', #29106 ) ;
#30444=ORIENTED_EDGE ( 'NONE', *, *, #2949, .F. ) ;
#30447=CARTESIAN_POINT ( 'NONE',  ( -56.06249999999995737, -1.962990915244707368, -3.400000000000206413 ) ) ;
#30460=CARTESIAN_POINT ( 'NONE',  ( -54.48571443722132557, -2.918663338619467140, -2.077054936585725819 ) ) ;
#30500=VECTOR ( 'NONE', #19451, 1000.000000000000000 ) ;
#30501=CARTESIAN_POINT ( 'NONE',  ( -58.57202994616204705, 2.078460969082646770, 3.599999999999799805 ) ) ;
#30507=CARTESIAN_POINT ( 'NONE',  ( -54.49999999999996447, 1.557046979865791991, -3.273565289175131454 ) ) ;
#30515=CARTESIAN_POINT ( 'NONE',  ( -57.18749999999997868, 1.962990915244718915, 3.399999999999805844 ) ) ;
#30524=DIRECTION ( 'NONE',  ( -1.000000000000000000, 1.219044193948983948E-29, -3.491481338843133355E-15 ) ) ;
#30525=CARTESIAN_POINT ( 'NONE',  ( -61.13452994616202574, 2.093608279459375190E-14, -3.600000000000216804 ) ) ;
#30536=EDGE_CURVE ( 'NONE', #10254, #24129, #21572, .T. ) ;
#30548=CIRCLE ( 'NONE', #16929, 0.2000000000000000944 ) ;
#30565=CARTESIAN_POINT ( 'NONE',  ( -54.49999999999999289, -1.500000000000006883, 4.029888335921739895 ) ) ;
#30567=CARTESIAN_POINT ( 'NONE',  ( -59.69999999999996021, -2.194112688547747325, -2.851241005161186504 ) ) ;
#30569=CARTESIAN_POINT ( 'NONE',  ( -54.75952994616206837, -4.643455692769931152E-15, 3.599999999999804245 ) ) ;
#30570=CARTESIAN_POINT ( 'NONE',  ( -57.95655989232411542, 1.962990915244748891, -3.400000000000197087 ) ) ;
#30571=ORIENTED_EDGE ( 'NONE', *, *, #24738, .F. ) ;
#30573=VERTEX_POINT ( 'NONE', #3459 ) ;
#30576=ORIENTED_EDGE ( 'NONE', *, *, #26993, .T. ) ;
#30578=CARTESIAN_POINT ( 'NONE',  ( -58.43749999999997158, -3.925981830489445379, -2.215933297149796442E-13 ) ) ;
#30588=CARTESIAN_POINT ( 'NONE',  ( -59.61160122551025609, 2.340542558125672912, -1.243912201914818771 ) ) ;
#30603=CARTESIAN_POINT ( 'NONE',  ( -55.19702994616203284, -2.078460969082631227, -3.600000000000202593 ) ) ;
#30605=ORIENTED_EDGE ( 'NONE', *, *, #13044, .T. ) ;
#30635=AXIS2_PLACEMENT_3D ( 'NONE', #19409, #9894, #396 ) ;
#30643=VERTEX_POINT ( 'NONE', #3914 ) ;
#30654=VERTEX_POINT ( 'NONE', #15790 ) ;
#30659=CIRCLE ( 'NONE', #27710, 3.399999999999999911 ) ;
#30660=CARTESIAN_POINT ( 'NONE',  ( -55.95655989232413674, -3.399999999999990585, -2.144552914728849520E-13 ) ) ;
#30670=CARTESIAN_POINT ( 'NONE',  ( -59.44702994616203995, 4.156921938165313080, -1.958927657850919798E-13 ) ) ;
#30712=CARTESIAN_POINT ( 'NONE',  ( -54.39999999999997726, 8.366749974758487600E-15, -2.213041600731273397E-13 ) ) ;
#30716=EDGE_CURVE ( 'NONE', #30654, #20368, #25761, .T. ) ;
#30735=CARTESIAN_POINT ( 'NONE',  ( -59.19999999999996732, 2.569786949633446671, -0.9498634748674490424 ) ) ;
#30751=CARTESIAN_POINT ( 'NONE',  ( -55.69702994616204705, 4.156921938165313968, -1.817815585352543609E-13 ) ) ;
#30752=CARTESIAN_POINT ( 'NONE',  ( -58.83155989232410832, -1.962990915244706924, -3.400000000000215294 ) ) ;
#30756=CARTESIAN_POINT ( 'NONE',  ( -59.68749999999995737, 1.962990915244749557, -3.400000000000203304 ) ) ;
#30779=CARTESIAN_POINT ( 'NONE',  ( -59.43749999999997868, 1.962990915244722689, 3.399999999999796962 ) ) ;
#30785=VECTOR ( 'NONE', #7996, 1000.000000000000000 ) ;
#30801=FACE_OUTER_BOUND ( 'NONE', #3323, .T. ) ;
#30832=EDGE_CURVE ( 'NONE', #26017, #7227, #29741, .T. ) ;
#30836=CARTESIAN_POINT ( 'NONE',  ( -59.88452994616203995, -3.117691453623976816, 1.799999999999775335 ) ) ;
#30849=ORIENTED_EDGE ( 'NONE', *, *, #412, .T. ) ;
#30854=VECTOR ( 'NONE', #4337, 1000.000000000000000 ) ;
#30858=VERTEX_POINT ( 'NONE', #31296 ) ;
#30881=CARTESIAN_POINT ( 'NONE',  ( -54.39999999999997726, 8.366749974758389781E-15, -1.935485844574984262E-13 ) ) ;
#30884=DIRECTION ( 'NONE',  ( 5.182136041040955759E-15, -3.491481338843133355E-15, 1.000000000000000000 ) ) ;
#30895=ADVANCED_FACE ( 'NONE', ( #17977 ), #4029, .T. ) ;
#30911=CARTESIAN_POINT ( 'NONE',  ( -59.37499999999997868, -3.920666489018300969E-15, 3.399999999999788525 ) ) ;
#30912=DIRECTION ( 'NONE',  ( 1.000000000000000000, -1.219044193948983948E-29, 3.491481338843133355E-15 ) ) ;
#30915=EDGE_CURVE ( 'NONE', #17824, #15088, #24783, .T. ) ;
#30936=CARTESIAN_POINT ( 'NONE',  ( -60.87499999999997158, -3.920666489018282036E-15, 3.399999999999783196 ) ) ;
#30951=CARTESIAN_POINT ( 'NONE',  ( -55.62499999999998579, -4.753426312438546834E-15, 3.399999999999801403 ) ) ;
#30959=EDGE_CURVE ( 'NONE', #3568, #21890, #21628, .T. ) ;
#30973=ORIENTED_EDGE ( 'NONE', *, *, #20017, .F. ) ;
#30976=ORIENTED_EDGE ( 'NONE', *, *, #22799, .F. ) ;
#30983=CARTESIAN_POINT ( 'NONE',  ( -59.40362242792826919, 3.375967812128700452, 1.250136525132546916 ) ) ;
#30985=CARTESIAN_POINT ( 'NONE',  ( -59.13452994616204705, -3.117691453623976816, 1.799999999999778000 ) ) ;
#30991=AXIS2_PLACEMENT_3D ( 'NONE', #21777, #2111, #31255 ) ;
#31009=ORIENTED_EDGE ( 'NONE', *, *, #26349, .F. ) ;
#31056=CARTESIAN_POINT ( 'NONE',  ( -60.74999999999997158, -2.944486372867089141, 1.699999999999773248 ) ) ;
#31060=DIRECTION ( 'NONE',  ( -2.095850865446309212E-30, -1.000000000000000000, -2.891205793294679411E-15 ) ) ;
#31067=ORIENTED_EDGE ( 'NONE', *, *, #28019, .F. ) ;
#31074=DIRECTION ( 'NONE',  ( 1.000000000000000000, -1.219044193948983948E-29, 3.491481338843133355E-15 ) ) ;
#31081=CARTESIAN_POINT ( 'NONE',  ( -54.88452994616206126, 3.117691453623979481, 1.799999999999816858 ) ) ;
#31088=CARTESIAN_POINT ( 'NONE',  ( -58.13452994616202574, 2.093608279459371404E-14, -3.600000000000206146 ) ) ;
#31117=CARTESIAN_POINT ( 'NONE',  ( -59.17288345746447220, -2.377187522396925434, 1.240801385673783841 ) ) ;
#31121=DIRECTION ( 'NONE',  ( 0.000000000000000000, -1.000000000000000000, -3.491481338843130594E-15 ) ) ;
#31126=EDGE_LOOP ( 'NONE', ( #22850, #17174, #12453 ) ) ;
#31127=DIRECTION ( 'NONE',  ( 1.000000000000000000, -1.219044193948983948E-29, 3.491481338843133355E-15 ) ) ;
#31128=EDGE_LOOP ( 'NONE', ( #23172, #12422, #17273 ) ) ;
#31130=CARTESIAN_POINT ( 'NONE',  ( -59.69999999999997442, 3.166389444283797872, -1.238538609462263462 ) ) ;
#31133=DIRECTION ( 'NONE',  ( -3.491481338843133355E-15, -3.491481338843133355E-15, 1.000000000000000000 ) ) ;
#31141=CARTESIAN_POINT ( 'NONE',  ( -56.44702994616204705, 4.156921938165313080, -1.854183217685626176E-13 ) ) ;
#31145=CARTESIAN_POINT ( 'NONE',  ( -58.56249999999998579, -1.962990915244733792, 3.399999999999783196 ) ) ;
#31168=EDGE_CURVE ( 'NONE', #1825, #16856, #14874, .T. ) ;
#31179=CARTESIAN_POINT ( 'NONE',  ( -55.20655989232412963, -3.399999999999991473, -2.086450695418937968E-13 ) ) ;
#31202=CARTESIAN_POINT ( 'NONE',  ( -59.60202821895190795, 2.022779453259406779, 1.712000320153392208 ) ) ;
#31204=FACE_OUTER_BOUND ( 'NONE', #19021, .T. ) ;
#31214=ADVANCED_FACE ( 'NONE', ( #17636 ), #8520, .T. ) ;
#31215=ORIENTED_EDGE ( 'NONE', *, *, #18261, .T. ) ;
#31230=CARTESIAN_POINT ( 'NONE',  ( -60.18749999999998579, 1.962990915244722689, 3.399999999999794742 ) ) ;
#31255=DIRECTION ( 'NONE',  ( 0.000000000000000000, 1.000000000000000000, 3.491481338843132961E-15 ) ) ;
#31256=CARTESIAN_POINT ( 'NONE',  ( -59.93749999999996447, -3.925981830489445379, -2.268305517232443506E-13 ) ) ;
#31261=CARTESIAN_POINT ( 'NONE',  ( -56.88452994616205416, -3.117691453623976816, 1.799999999999785993 ) ) ;
#31273=CARTESIAN_POINT ( 'NONE',  ( -59.41007723054021028, 2.404624529862326554, 1.250136525132548027 ) ) ;
#31281=VERTEX_POINT ( 'NONE', #29813 ) ;
#31282=EDGE_CURVE ( 'NONE', #11667, #20201, #2470, .T. ) ;
#31283=CARTESIAN_POINT ( 'NONE',  ( -59.10658905376791949, -2.332889649973222568, 1.257260963603446635 ) ) ;
#31296=CARTESIAN_POINT ( 'NONE',  ( -59.19126343180466421, -2.406052454186071277, 1.245092465133171844 ) ) ;
#31297=CARTESIAN_POINT ( 'NONE',  ( -59.69142724121850563, 2.412383461849218591, -1.233589124872089826 ) ) ;
#31301=CARTESIAN_POINT ( 'NONE',  ( -54.51905989232412963, -2.944486372867088697, 1.699999999999795008 ) ) ;
#31302=CARTESIAN_POINT ( 'NONE',  ( -57.08155989232412963, 3.400000000000007905, -1.873796572744660248E-13 ) ) ;
#31312=CARTESIAN_POINT ( 'NONE',  ( -59.69999999999997442, -2.450988139641045560, -1.238538609462283668 ) ) ;
#31316=AXIS2_PLACEMENT_3D ( 'NONE', #4573, #30524, #14221 ) ;
#31317=ORIENTED_EDGE ( 'NONE', *, *, #27216, .F. ) ;
#31318=EDGE_CURVE ( 'NONE', #9593, #5117, #19662, .T. ) ;
#31324=CARTESIAN_POINT ( 'NONE',  ( -59.19999999999997442, 4.156921938165317520, -0.9498634748674451567 ) ) ;
#31325=COLOUR_RGB ( '', 0.31764706, 0.68627451, 0.89019608) ;
ENDSEC;
END-ISO-10303-21;
